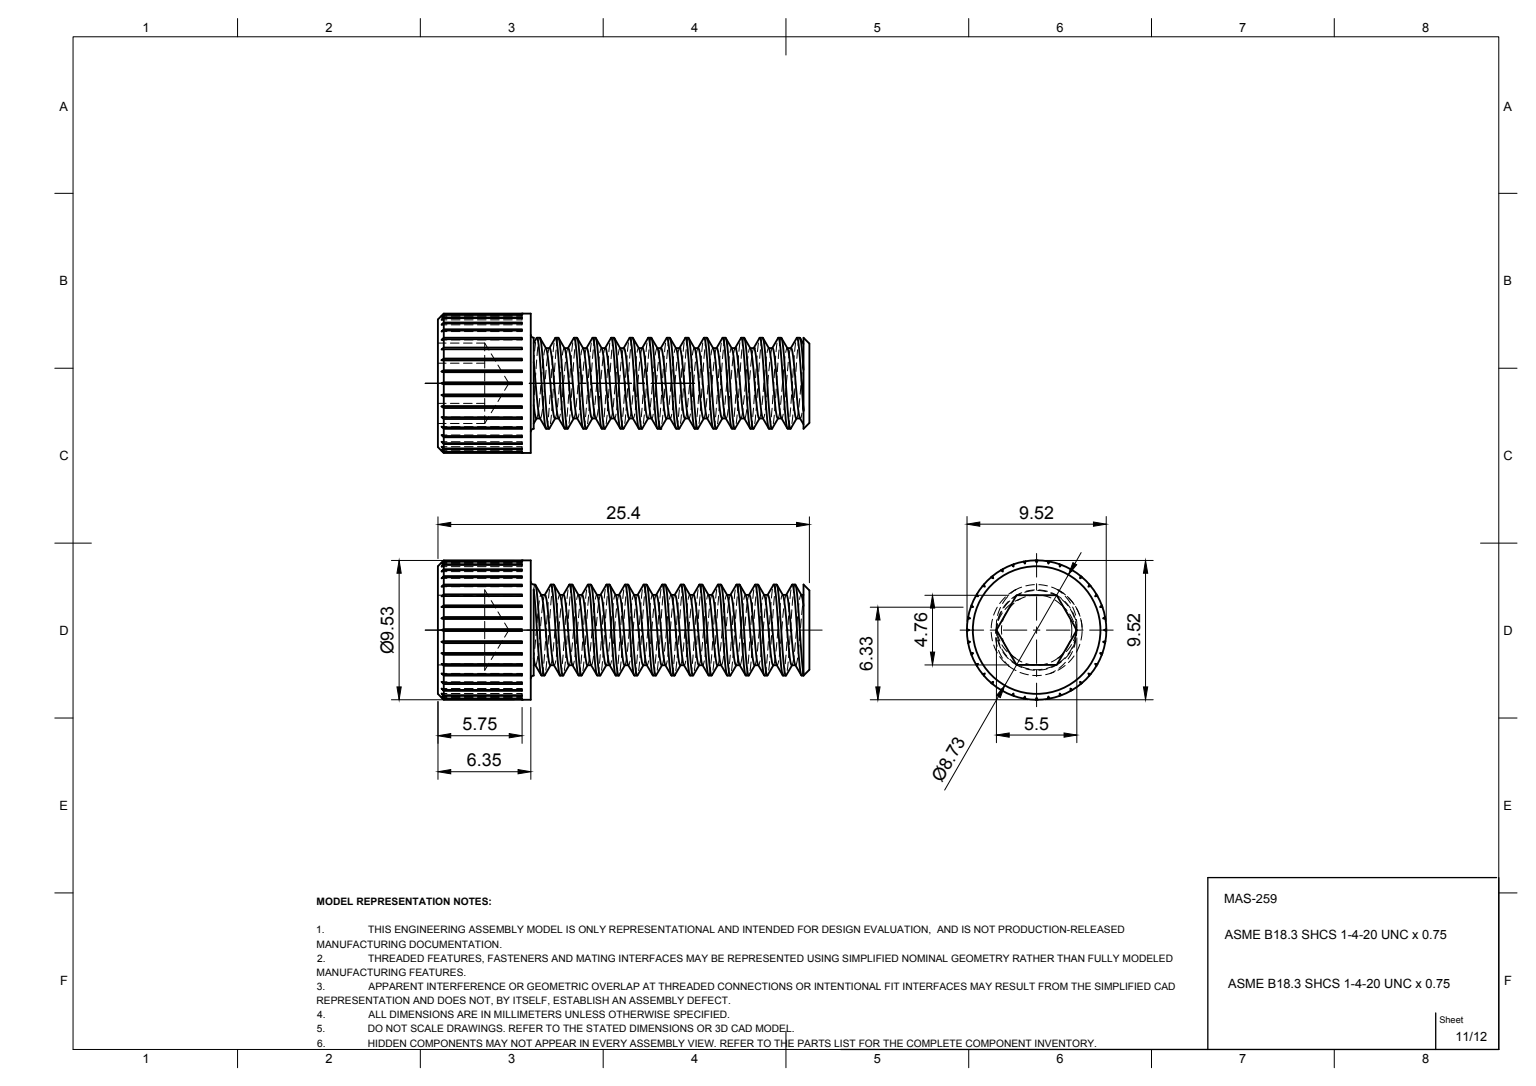
ISO-10303-21;
HEADER;
/* Generated by software containing ST-Developer
 * from STEP Tools, Inc. (www.steptools.com) 
 */

FILE_DESCRIPTION(
/* description */ (''),
/* implementation_level */ '2;1');

FILE_NAME(
/* name */ 'ASME B18.3 SHCS 1-4-20 UNC x 0.75.step',
/* time_stamp */ '2026-10-15T13:30:17-07:00',
/* author */ (''),
/* organization */ (''),
/* preprocessor_version */ 'ST-DEVELOPER v20.2',
/* originating_system */ 'Autodesk Translation Framework v15.15.0.0',
/* authorisation */ '');

FILE_SCHEMA (('AUTOMOTIVE_DESIGN { 1 0 10303 214 3 1 1 }'));
ENDSEC;

DATA;
#10=MECHANICAL_DESIGN_GEOMETRIC_PRESENTATION_REPRESENTATION('',(#1042),#71795);
#931=(
BOUNDED_CURVE()
B_SPLINE_CURVE(2,(#70734,#70735,#70736),.UNSPECIFIED.,.F.,.F.)
B_SPLINE_CURVE_WITH_KNOTS((3,3),(0.,0.0215367144649105),.UNSPECIFIED.)
CURVE()
GEOMETRIC_REPRESENTATION_ITEM()
RATIONAL_B_SPLINE_CURVE((1.,1.00042008979832,1.00053542481542))
REPRESENTATION_ITEM('')
);
#932=(
BOUNDED_CURVE()
B_SPLINE_CURVE(2,(#70741,#70742,#70743),.UNSPECIFIED.,.F.,.F.)
B_SPLINE_CURVE_WITH_KNOTS((3,3),(0.0378379342266191,0.0593746486914489),
 .UNSPECIFIED.)
CURVE()
GEOMETRIC_REPRESENTATION_ITEM()
RATIONAL_B_SPLINE_CURVE((1.00053542482002,1.00042008980193,1.))
REPRESENTATION_ITEM('')
);
#933=(
BOUNDED_CURVE()
B_SPLINE_CURVE(2,(#70750,#70751,#70752),.UNSPECIFIED.,.F.,.F.)
B_SPLINE_CURVE_WITH_KNOTS((3,3),(0.0378379342265495,0.0593746486914482),
 .UNSPECIFIED.)
CURVE()
GEOMETRIC_REPRESENTATION_ITEM()
RATIONAL_B_SPLINE_CURVE((1.00053542481289,1.00042008979634,1.))
REPRESENTATION_ITEM('')
);
#934=(
BOUNDED_CURVE()
B_SPLINE_CURVE(2,(#70756,#70757,#70758),.UNSPECIFIED.,.F.,.F.)
B_SPLINE_CURVE_WITH_KNOTS((3,3),(0.,0.0215367144649402),.UNSPECIFIED.)
CURVE()
GEOMETRIC_REPRESENTATION_ITEM()
RATIONAL_B_SPLINE_CURVE((1.,1.00042008979471,1.00053542481081))
REPRESENTATION_ITEM('')
);
#935=(
BOUNDED_CURVE()
B_SPLINE_CURVE(2,(#70760,#70761,#70762),.UNSPECIFIED.,.F.,.F.)
B_SPLINE_CURVE_WITH_KNOTS((3,3),(0.0378379342265241,0.0593746486914486),
 .UNSPECIFIED.)
CURVE()
GEOMETRIC_REPRESENTATION_ITEM()
RATIONAL_B_SPLINE_CURVE((1.00053542481258,1.0004200897961,1.))
REPRESENTATION_ITEM('')
);
#936=(
BOUNDED_CURVE()
B_SPLINE_CURVE(2,(#70766,#70767,#70768),.UNSPECIFIED.,.F.,.F.)
B_SPLINE_CURVE_WITH_KNOTS((3,3),(0.,0.0215367144649098),.UNSPECIFIED.)
CURVE()
GEOMETRIC_REPRESENTATION_ITEM()
RATIONAL_B_SPLINE_CURVE((1.,1.00042008979542,1.00053542481172))
REPRESENTATION_ITEM('')
);
#937=(
BOUNDED_CURVE()
B_SPLINE_CURVE(2,(#70770,#70771,#70772),.UNSPECIFIED.,.F.,.F.)
B_SPLINE_CURVE_WITH_KNOTS((3,3),(0.0378379342265049,0.0593746486914484),
 .UNSPECIFIED.)
CURVE()
GEOMETRIC_REPRESENTATION_ITEM()
RATIONAL_B_SPLINE_CURVE((1.00053542481297,1.0004200897964,1.))
REPRESENTATION_ITEM('')
);
#938=(
BOUNDED_CURVE()
B_SPLINE_CURVE(2,(#70776,#70777,#70778),.UNSPECIFIED.,.F.,.F.)
B_SPLINE_CURVE_WITH_KNOTS((3,3),(0.,0.0215367144648988),.UNSPECIFIED.)
CURVE()
GEOMETRIC_REPRESENTATION_ITEM()
RATIONAL_B_SPLINE_CURVE((1.,1.00042008979632,1.00053542481287))
REPRESENTATION_ITEM('')
);
#939=(
BOUNDED_CURVE()
B_SPLINE_CURVE(2,(#70780,#70781,#70782),.UNSPECIFIED.,.F.,.F.)
B_SPLINE_CURVE_WITH_KNOTS((3,3),(0.0378379342265885,0.0593746486914481),
 .UNSPECIFIED.)
CURVE()
GEOMETRIC_REPRESENTATION_ITEM()
RATIONAL_B_SPLINE_CURVE((1.00053542481452,1.00042008979762,1.))
REPRESENTATION_ITEM('')
);
#940=(
BOUNDED_CURVE()
B_SPLINE_CURVE(2,(#70786,#70787,#70788),.UNSPECIFIED.,.F.,.F.)
B_SPLINE_CURVE_WITH_KNOTS((3,3),(0.,0.021536714464922),.UNSPECIFIED.)
CURVE()
GEOMETRIC_REPRESENTATION_ITEM()
RATIONAL_B_SPLINE_CURVE((1.,1.0004200897977,1.00053542481463))
REPRESENTATION_ITEM('')
);
#941=(
BOUNDED_CURVE()
B_SPLINE_CURVE(2,(#70790,#70791,#70792),.UNSPECIFIED.,.F.,.F.)
B_SPLINE_CURVE_WITH_KNOTS((3,3),(0.0378379342265092,0.0593746486914482),
 .UNSPECIFIED.)
CURVE()
GEOMETRIC_REPRESENTATION_ITEM()
RATIONAL_B_SPLINE_CURVE((1.00053542481205,1.00042008979567,1.))
REPRESENTATION_ITEM('')
);
#942=(
BOUNDED_CURVE()
B_SPLINE_CURVE(2,(#70796,#70797,#70798),.UNSPECIFIED.,.F.,.F.)
B_SPLINE_CURVE_WITH_KNOTS((3,3),(0.,0.0215367144648869),.UNSPECIFIED.)
CURVE()
GEOMETRIC_REPRESENTATION_ITEM()
RATIONAL_B_SPLINE_CURVE((1.,1.00042008979756,1.00053542481445))
REPRESENTATION_ITEM('')
);
#943=(
BOUNDED_CURVE()
B_SPLINE_CURVE(2,(#70800,#70801,#70802),.UNSPECIFIED.,.F.,.F.)
B_SPLINE_CURVE_WITH_KNOTS((3,3),(0.0378379342265307,0.0593746486914478),
 .UNSPECIFIED.)
CURVE()
GEOMETRIC_REPRESENTATION_ITEM()
RATIONAL_B_SPLINE_CURVE((1.00053542481432,1.00042008979746,1.))
REPRESENTATION_ITEM('')
);
#944=(
BOUNDED_CURVE()
B_SPLINE_CURVE(2,(#70806,#70807,#70808),.UNSPECIFIED.,.F.,.F.)
B_SPLINE_CURVE_WITH_KNOTS((3,3),(0.,0.0215367144649457),.UNSPECIFIED.)
CURVE()
GEOMETRIC_REPRESENTATION_ITEM()
RATIONAL_B_SPLINE_CURVE((1.,1.00042008979626,1.00053542481279))
REPRESENTATION_ITEM('')
);
#945=(
BOUNDED_CURVE()
B_SPLINE_CURVE(2,(#70810,#70811,#70812),.UNSPECIFIED.,.F.,.F.)
B_SPLINE_CURVE_WITH_KNOTS((3,3),(0.0378379342264978,0.0593746486914476),
 .UNSPECIFIED.)
CURVE()
GEOMETRIC_REPRESENTATION_ITEM()
RATIONAL_B_SPLINE_CURVE((1.00053542480725,1.00042008979192,1.))
REPRESENTATION_ITEM('')
);
#946=(
BOUNDED_CURVE()
B_SPLINE_CURVE(2,(#70816,#70817,#70818),.UNSPECIFIED.,.F.,.F.)
B_SPLINE_CURVE_WITH_KNOTS((3,3),(0.,0.0215367144648818),.UNSPECIFIED.)
CURVE()
GEOMETRIC_REPRESENTATION_ITEM()
RATIONAL_B_SPLINE_CURVE((1.,1.00042008979656,1.00053542481317))
REPRESENTATION_ITEM('')
);
#947=(
BOUNDED_CURVE()
B_SPLINE_CURVE(2,(#70820,#70821,#70822),.UNSPECIFIED.,.F.,.F.)
B_SPLINE_CURVE_WITH_KNOTS((3,3),(0.0378379342265614,0.0593746486914475),
 .UNSPECIFIED.)
CURVE()
GEOMETRIC_REPRESENTATION_ITEM()
RATIONAL_B_SPLINE_CURVE((1.00053542481625,1.00042008979897,1.))
REPRESENTATION_ITEM('')
);
#948=(
BOUNDED_CURVE()
B_SPLINE_CURVE(2,(#70826,#70827,#70828),.UNSPECIFIED.,.F.,.F.)
B_SPLINE_CURVE_WITH_KNOTS((3,3),(0.,0.0215367144648944),.UNSPECIFIED.)
CURVE()
GEOMETRIC_REPRESENTATION_ITEM()
RATIONAL_B_SPLINE_CURVE((1.,1.00042008979746,1.00053542481432))
REPRESENTATION_ITEM('')
);
#949=(
BOUNDED_CURVE()
B_SPLINE_CURVE(2,(#70830,#70831,#70832),.UNSPECIFIED.,.F.,.F.)
B_SPLINE_CURVE_WITH_KNOTS((3,3),(0.0378379342265643,0.0593746486914474),
 .UNSPECIFIED.)
CURVE()
GEOMETRIC_REPRESENTATION_ITEM()
RATIONAL_B_SPLINE_CURVE((1.00053542481547,1.00042008979836,1.))
REPRESENTATION_ITEM('')
);
#950=(
BOUNDED_CURVE()
B_SPLINE_CURVE(2,(#70836,#70837,#70838),.UNSPECIFIED.,.F.,.F.)
B_SPLINE_CURVE_WITH_KNOTS((3,3),(0.,0.0215367144648979),.UNSPECIFIED.)
CURVE()
GEOMETRIC_REPRESENTATION_ITEM()
RATIONAL_B_SPLINE_CURVE((1.,1.00042008979658,1.00053542481321))
REPRESENTATION_ITEM('')
);
#951=(
BOUNDED_CURVE()
B_SPLINE_CURVE(2,(#70840,#70841,#70842),.UNSPECIFIED.,.F.,.F.)
B_SPLINE_CURVE_WITH_KNOTS((3,3),(0.037837934226498,0.0593746486914474),
 .UNSPECIFIED.)
CURVE()
GEOMETRIC_REPRESENTATION_ITEM()
RATIONAL_B_SPLINE_CURVE((1.00053542481105,1.0004200897949,1.))
REPRESENTATION_ITEM('')
);
#952=(
BOUNDED_CURVE()
B_SPLINE_CURVE(2,(#70846,#70847,#70848),.UNSPECIFIED.,.F.,.F.)
B_SPLINE_CURVE_WITH_KNOTS((3,3),(0.,0.021536714464896),.UNSPECIFIED.)
CURVE()
GEOMETRIC_REPRESENTATION_ITEM()
RATIONAL_B_SPLINE_CURVE((1.,1.00042008979607,1.00053542481255))
REPRESENTATION_ITEM('')
);
#953=(
BOUNDED_CURVE()
B_SPLINE_CURVE(2,(#70850,#70851,#70852),.UNSPECIFIED.,.F.,.F.)
B_SPLINE_CURVE_WITH_KNOTS((3,3),(0.0378379342264847,0.0593746486914478),
 .UNSPECIFIED.)
CURVE()
GEOMETRIC_REPRESENTATION_ITEM()
RATIONAL_B_SPLINE_CURVE((1.00053542480987,1.00042008979397,1.))
REPRESENTATION_ITEM('')
);
#954=(
BOUNDED_CURVE()
B_SPLINE_CURVE(2,(#70856,#70857,#70858),.UNSPECIFIED.,.F.,.F.)
B_SPLINE_CURVE_WITH_KNOTS((3,3),(0.,0.0215367144649515),.UNSPECIFIED.)
CURVE()
GEOMETRIC_REPRESENTATION_ITEM()
RATIONAL_B_SPLINE_CURVE((1.,1.00042008979379,1.00053542480965))
REPRESENTATION_ITEM('')
);
#955=(
BOUNDED_CURVE()
B_SPLINE_CURVE(2,(#70860,#70861,#70862),.UNSPECIFIED.,.F.,.F.)
B_SPLINE_CURVE_WITH_KNOTS((3,3),(0.0378379342265934,0.0593746486914471),
 .UNSPECIFIED.)
CURVE()
GEOMETRIC_REPRESENTATION_ITEM()
RATIONAL_B_SPLINE_CURVE((1.00053542481303,1.00042008979644,1.))
REPRESENTATION_ITEM('')
);
#956=(
BOUNDED_CURVE()
B_SPLINE_CURVE(2,(#70866,#70867,#70868),.UNSPECIFIED.,.F.,.F.)
B_SPLINE_CURVE_WITH_KNOTS((3,3),(0.,0.0215367144649196),.UNSPECIFIED.)
CURVE()
GEOMETRIC_REPRESENTATION_ITEM()
RATIONAL_B_SPLINE_CURVE((1.,1.00042008979619,1.00053542481271))
REPRESENTATION_ITEM('')
);
#957=(
BOUNDED_CURVE()
B_SPLINE_CURVE(2,(#70870,#70871,#70872),.UNSPECIFIED.,.F.,.F.)
B_SPLINE_CURVE_WITH_KNOTS((3,3),(0.0378379342265594,0.0593746486914476),
 .UNSPECIFIED.)
CURVE()
GEOMETRIC_REPRESENTATION_ITEM()
RATIONAL_B_SPLINE_CURVE((1.00053542481439,1.00042008979752,1.))
REPRESENTATION_ITEM('')
);
#958=(
BOUNDED_CURVE()
B_SPLINE_CURVE(2,(#70876,#70877,#70878),.UNSPECIFIED.,.F.,.F.)
B_SPLINE_CURVE_WITH_KNOTS((3,3),(0.,0.0215367144649124),.UNSPECIFIED.)
CURVE()
GEOMETRIC_REPRESENTATION_ITEM()
RATIONAL_B_SPLINE_CURVE((1.,1.00042008979906,1.00053542481637))
REPRESENTATION_ITEM('')
);
#959=(
BOUNDED_CURVE()
B_SPLINE_CURVE(2,(#70880,#70881,#70882),.UNSPECIFIED.,.F.,.F.)
B_SPLINE_CURVE_WITH_KNOTS((3,3),(0.0378379342265818,0.0593746486914467),
 .UNSPECIFIED.)
CURVE()
GEOMETRIC_REPRESENTATION_ITEM()
RATIONAL_B_SPLINE_CURVE((1.00053542480684,1.00042008979159,1.))
REPRESENTATION_ITEM('')
);
#960=(
BOUNDED_CURVE()
B_SPLINE_CURVE(2,(#70886,#70887,#70888),.UNSPECIFIED.,.F.,.F.)
B_SPLINE_CURVE_WITH_KNOTS((3,3),(0.,0.021536714464952),.UNSPECIFIED.)
CURVE()
GEOMETRIC_REPRESENTATION_ITEM()
RATIONAL_B_SPLINE_CURVE((1.,1.00042008979707,1.00053542481383))
REPRESENTATION_ITEM('')
);
#961=(
BOUNDED_CURVE()
B_SPLINE_CURVE(2,(#70890,#70891,#70892),.UNSPECIFIED.,.F.,.F.)
B_SPLINE_CURVE_WITH_KNOTS((3,3),(0.0378379342265293,0.0593746486914474),
 .UNSPECIFIED.)
CURVE()
GEOMETRIC_REPRESENTATION_ITEM()
RATIONAL_B_SPLINE_CURVE((1.00053542480889,1.0004200897932,1.))
REPRESENTATION_ITEM('')
);
#962=(
BOUNDED_CURVE()
B_SPLINE_CURVE(2,(#70896,#70897,#70898),.UNSPECIFIED.,.F.,.F.)
B_SPLINE_CURVE_WITH_KNOTS((3,3),(0.,0.0215367144649713),.UNSPECIFIED.)
CURVE()
GEOMETRIC_REPRESENTATION_ITEM()
RATIONAL_B_SPLINE_CURVE((1.,1.00042008978867,1.00053542480312))
REPRESENTATION_ITEM('')
);
#963=(
BOUNDED_CURVE()
B_SPLINE_CURVE(2,(#70900,#70901,#70902),.UNSPECIFIED.,.F.,.F.)
B_SPLINE_CURVE_WITH_KNOTS((3,3),(0.0378379342265233,0.0593746486914479),
 .UNSPECIFIED.)
CURVE()
GEOMETRIC_REPRESENTATION_ITEM()
RATIONAL_B_SPLINE_CURVE((1.00053542481454,1.00042008979763,1.))
REPRESENTATION_ITEM('')
);
#964=(
BOUNDED_CURVE()
B_SPLINE_CURVE(2,(#70906,#70907,#70908),.UNSPECIFIED.,.F.,.F.)
B_SPLINE_CURVE_WITH_KNOTS((3,3),(0.,0.0215367144648066),.UNSPECIFIED.)
CURVE()
GEOMETRIC_REPRESENTATION_ITEM()
RATIONAL_B_SPLINE_CURVE((1.,1.00042008980092,1.00053542481873))
REPRESENTATION_ITEM('')
);
#965=(
BOUNDED_CURVE()
B_SPLINE_CURVE(2,(#70910,#70911,#70912),.UNSPECIFIED.,.F.,.F.)
B_SPLINE_CURVE_WITH_KNOTS((3,3),(0.0378379342265035,0.0593746486914475),
 .UNSPECIFIED.)
CURVE()
GEOMETRIC_REPRESENTATION_ITEM()
RATIONAL_B_SPLINE_CURVE((1.00053542481437,1.0004200897975,1.))
REPRESENTATION_ITEM('')
);
#966=(
BOUNDED_CURVE()
B_SPLINE_CURVE(2,(#70916,#70917,#70918),.UNSPECIFIED.,.F.,.F.)
B_SPLINE_CURVE_WITH_KNOTS((3,3),(0.,0.0215367144649832),.UNSPECIFIED.)
CURVE()
GEOMETRIC_REPRESENTATION_ITEM()
RATIONAL_B_SPLINE_CURVE((1.,1.00042008978849,1.00053542480288))
REPRESENTATION_ITEM('')
);
#967=(
BOUNDED_CURVE()
B_SPLINE_CURVE(2,(#70920,#70921,#70922),.UNSPECIFIED.,.F.,.F.)
B_SPLINE_CURVE_WITH_KNOTS((3,3),(0.0378379342264869,0.0593746486914472),
 .UNSPECIFIED.)
CURVE()
GEOMETRIC_REPRESENTATION_ITEM()
RATIONAL_B_SPLINE_CURVE((1.00053542480856,1.00042008979294,1.))
REPRESENTATION_ITEM('')
);
#968=(
BOUNDED_CURVE()
B_SPLINE_CURVE(2,(#70926,#70927,#70928),.UNSPECIFIED.,.F.,.F.)
B_SPLINE_CURVE_WITH_KNOTS((3,3),(0.,0.0215367144648701),.UNSPECIFIED.)
CURVE()
GEOMETRIC_REPRESENTATION_ITEM()
RATIONAL_B_SPLINE_CURVE((1.,1.00042008979633,1.00053542481289))
REPRESENTATION_ITEM('')
);
#969=(
BOUNDED_CURVE()
B_SPLINE_CURVE(2,(#70930,#70931,#70932),.UNSPECIFIED.,.F.,.F.)
B_SPLINE_CURVE_WITH_KNOTS((3,3),(0.0378379342266196,0.0593746486914466),
 .UNSPECIFIED.)
CURVE()
GEOMETRIC_REPRESENTATION_ITEM()
RATIONAL_B_SPLINE_CURVE((1.00053542481627,1.00042008979899,1.))
REPRESENTATION_ITEM('')
);
#970=(
BOUNDED_CURVE()
B_SPLINE_CURVE(2,(#70937,#70938,#70939),.UNSPECIFIED.,.F.,.F.)
B_SPLINE_CURVE_WITH_KNOTS((3,3),(0.,0.0215367144649364),.UNSPECIFIED.)
CURVE()
GEOMETRIC_REPRESENTATION_ITEM()
RATIONAL_B_SPLINE_CURVE((1.,1.00042008979495,1.00053542481112))
REPRESENTATION_ITEM('')
);
#971=(
BOUNDED_CURVE()
B_SPLINE_CURVE(2,(#70941,#70942,#70943),.UNSPECIFIED.,.F.,.F.)
B_SPLINE_CURVE_WITH_KNOTS((3,3),(0.0378379342265907,0.0593746486914489),
 .UNSPECIFIED.)
CURVE()
GEOMETRIC_REPRESENTATION_ITEM()
RATIONAL_B_SPLINE_CURVE((1.00053542481339,1.00042008979673,1.))
REPRESENTATION_ITEM('')
);
#972=(
BOUNDED_CURVE()
B_SPLINE_CURVE(2,(#70947,#70948,#70949),.UNSPECIFIED.,.F.,.F.)
B_SPLINE_CURVE_WITH_KNOTS((3,3),(0.,0.0215367144648983),.UNSPECIFIED.)
CURVE()
GEOMETRIC_REPRESENTATION_ITEM()
RATIONAL_B_SPLINE_CURVE((1.,1.00042008979758,1.00053542481447))
REPRESENTATION_ITEM('')
);
#973=(
BOUNDED_CURVE()
B_SPLINE_CURVE(2,(#70951,#70952,#70953),.UNSPECIFIED.,.F.,.F.)
B_SPLINE_CURVE_WITH_KNOTS((3,3),(0.0378379342266009,0.0593746486914487),
 .UNSPECIFIED.)
CURVE()
GEOMETRIC_REPRESENTATION_ITEM()
RATIONAL_B_SPLINE_CURVE((1.00053542481762,1.00042008980005,1.))
REPRESENTATION_ITEM('')
);
#974=(
BOUNDED_CURVE()
B_SPLINE_CURVE(2,(#70957,#70958,#70959),.UNSPECIFIED.,.F.,.F.)
B_SPLINE_CURVE_WITH_KNOTS((3,3),(0.,0.0215367144648523),.UNSPECIFIED.)
CURVE()
GEOMETRIC_REPRESENTATION_ITEM()
RATIONAL_B_SPLINE_CURVE((1.,1.00042008980162,1.00053542481963))
REPRESENTATION_ITEM('')
);
#975=(
BOUNDED_CURVE()
B_SPLINE_CURVE(2,(#70961,#70962,#70963),.UNSPECIFIED.,.F.,.F.)
B_SPLINE_CURVE_WITH_KNOTS((3,3),(0.0378379342266166,0.0593746486914488),
 .UNSPECIFIED.)
CURVE()
GEOMETRIC_REPRESENTATION_ITEM()
RATIONAL_B_SPLINE_CURVE((1.00053542482459,1.00042008980551,1.))
REPRESENTATION_ITEM('')
);
#976=(
BOUNDED_CURVE()
B_SPLINE_CURVE(2,(#70967,#70968,#70969),.UNSPECIFIED.,.F.,.F.)
B_SPLINE_CURVE_WITH_KNOTS((3,3),(0.,0.0215367144649508),.UNSPECIFIED.)
CURVE()
GEOMETRIC_REPRESENTATION_ITEM()
RATIONAL_B_SPLINE_CURVE((1.,1.00042008979412,1.00053542481006))
REPRESENTATION_ITEM('')
);
#977=(
BOUNDED_CURVE()
B_SPLINE_CURVE(2,(#70971,#70972,#70973),.UNSPECIFIED.,.F.,.F.)
B_SPLINE_CURVE_WITH_KNOTS((3,3),(0.0378379342265848,0.0593746486914484),
 .UNSPECIFIED.)
CURVE()
GEOMETRIC_REPRESENTATION_ITEM()
RATIONAL_B_SPLINE_CURVE((1.00053542481552,1.0004200897984,1.))
REPRESENTATION_ITEM('')
);
#978=(
BOUNDED_CURVE()
B_SPLINE_CURVE(2,(#70977,#70978,#70979),.UNSPECIFIED.,.F.,.F.)
B_SPLINE_CURVE_WITH_KNOTS((3,3),(0.,0.0215367144649591),.UNSPECIFIED.)
CURVE()
GEOMETRIC_REPRESENTATION_ITEM()
RATIONAL_B_SPLINE_CURVE((1.,1.00042008979621,1.00053542481272))
REPRESENTATION_ITEM('')
);
#979=(
BOUNDED_CURVE()
B_SPLINE_CURVE(2,(#70981,#70982,#70983),.UNSPECIFIED.,.F.,.F.)
B_SPLINE_CURVE_WITH_KNOTS((3,3),(0.037837934226528,0.0593746486914486),
 .UNSPECIFIED.)
CURVE()
GEOMETRIC_REPRESENTATION_ITEM()
RATIONAL_B_SPLINE_CURVE((1.00053542481249,1.00042008979602,1.))
REPRESENTATION_ITEM('')
);
#980=(
BOUNDED_CURVE()
B_SPLINE_CURVE(2,(#70987,#70988,#70989),.UNSPECIFIED.,.F.,.F.)
B_SPLINE_CURVE_WITH_KNOTS((3,3),(0.,0.0215367144649439),.UNSPECIFIED.)
CURVE()
GEOMETRIC_REPRESENTATION_ITEM()
RATIONAL_B_SPLINE_CURVE((1.,1.00042008979311,1.00053542480878))
REPRESENTATION_ITEM('')
);
#981=(
BOUNDED_CURVE()
B_SPLINE_CURVE(2,(#70991,#70992,#70993),.UNSPECIFIED.,.F.,.F.)
B_SPLINE_CURVE_WITH_KNOTS((3,3),(0.0378379342265471,0.0593746486914486),
 .UNSPECIFIED.)
CURVE()
GEOMETRIC_REPRESENTATION_ITEM()
RATIONAL_B_SPLINE_CURVE((1.00053542480963,1.00042008979378,1.))
REPRESENTATION_ITEM('')
);
#982=(
BOUNDED_CURVE()
B_SPLINE_CURVE(2,(#70997,#70998,#70999),.UNSPECIFIED.,.F.,.F.)
B_SPLINE_CURVE_WITH_KNOTS((3,3),(0.,0.0215367144649546),.UNSPECIFIED.)
CURVE()
GEOMETRIC_REPRESENTATION_ITEM()
RATIONAL_B_SPLINE_CURVE((1.,1.00042008979267,1.00053542480822))
REPRESENTATION_ITEM('')
);
#983=(
BOUNDED_CURVE()
B_SPLINE_CURVE(2,(#71001,#71002,#71003),.UNSPECIFIED.,.F.,.F.)
B_SPLINE_CURVE_WITH_KNOTS((3,3),(0.0378379342265707,0.0593746486914487),
 .UNSPECIFIED.)
CURVE()
GEOMETRIC_REPRESENTATION_ITEM()
RATIONAL_B_SPLINE_CURVE((1.0005354248134,1.00042008979673,1.))
REPRESENTATION_ITEM('')
);
#984=(
BOUNDED_CURVE()
B_SPLINE_CURVE(2,(#71007,#71008,#71009),.UNSPECIFIED.,.F.,.F.)
B_SPLINE_CURVE_WITH_KNOTS((3,3),(0.,0.0215367144649525),.UNSPECIFIED.)
CURVE()
GEOMETRIC_REPRESENTATION_ITEM()
RATIONAL_B_SPLINE_CURVE((1.,1.0004200897947,1.0005354248108))
REPRESENTATION_ITEM('')
);
#985=(
BOUNDED_CURVE()
B_SPLINE_CURVE(2,(#71011,#71012,#71013),.UNSPECIFIED.,.F.,.F.)
B_SPLINE_CURVE_WITH_KNOTS((3,3),(0.0378379342265302,0.059374648691449),
 .UNSPECIFIED.)
CURVE()
GEOMETRIC_REPRESENTATION_ITEM()
RATIONAL_B_SPLINE_CURVE((1.00053542480972,1.00042008979385,1.))
REPRESENTATION_ITEM('')
);
#986=(
BOUNDED_CURVE()
B_SPLINE_CURVE(2,(#71017,#71018,#71019),.UNSPECIFIED.,.F.,.F.)
B_SPLINE_CURVE_WITH_KNOTS((3,3),(0.,0.0215367144649366),.UNSPECIFIED.)
CURVE()
GEOMETRIC_REPRESENTATION_ITEM()
RATIONAL_B_SPLINE_CURVE((1.,1.00042008979726,1.00053542481407))
REPRESENTATION_ITEM('')
);
#987=(
BOUNDED_CURVE()
B_SPLINE_CURVE(2,(#71021,#71022,#71023),.UNSPECIFIED.,.F.,.F.)
B_SPLINE_CURVE_WITH_KNOTS((3,3),(0.0378379342265197,0.0593746486914487),
 .UNSPECIFIED.)
CURVE()
GEOMETRIC_REPRESENTATION_ITEM()
RATIONAL_B_SPLINE_CURVE((1.00053542480866,1.00042008979301,1.))
REPRESENTATION_ITEM('')
);
#988=(
BOUNDED_CURVE()
B_SPLINE_CURVE(2,(#71027,#71028,#71029),.UNSPECIFIED.,.F.,.F.)
B_SPLINE_CURVE_WITH_KNOTS((3,3),(0.,0.0215367144649012),.UNSPECIFIED.)
CURVE()
GEOMETRIC_REPRESENTATION_ITEM()
RATIONAL_B_SPLINE_CURVE((1.,1.00042008979525,1.0005354248115))
REPRESENTATION_ITEM('')
);
#989=(
BOUNDED_CURVE()
B_SPLINE_CURVE(2,(#71031,#71032,#71033),.UNSPECIFIED.,.F.,.F.)
B_SPLINE_CURVE_WITH_KNOTS((3,3),(0.0378379342265321,0.0593746486914488),
 .UNSPECIFIED.)
CURVE()
GEOMETRIC_REPRESENTATION_ITEM()
RATIONAL_B_SPLINE_CURVE((1.00053542481087,1.00042008979475,1.))
REPRESENTATION_ITEM('')
);
#990=(
BOUNDED_CURVE()
B_SPLINE_CURVE(2,(#71037,#71038,#71039),.UNSPECIFIED.,.F.,.F.)
B_SPLINE_CURVE_WITH_KNOTS((3,3),(0.,0.0215367144649128),.UNSPECIFIED.)
CURVE()
GEOMETRIC_REPRESENTATION_ITEM()
RATIONAL_B_SPLINE_CURVE((1.,1.00042008979245,1.00053542480793))
REPRESENTATION_ITEM('')
);
#991=(
BOUNDED_CURVE()
B_SPLINE_CURVE(2,(#71041,#71042,#71043),.UNSPECIFIED.,.F.,.F.)
B_SPLINE_CURVE_WITH_KNOTS((3,3),(0.0378379342265115,0.0593746486914485),
 .UNSPECIFIED.)
CURVE()
GEOMETRIC_REPRESENTATION_ITEM()
RATIONAL_B_SPLINE_CURVE((1.0005354248112,1.00042008979501,1.))
REPRESENTATION_ITEM('')
);
#992=(
BOUNDED_CURVE()
B_SPLINE_CURVE(2,(#71047,#71048,#71049),.UNSPECIFIED.,.F.,.F.)
B_SPLINE_CURVE_WITH_KNOTS((3,3),(0.,0.0215367144649508),.UNSPECIFIED.)
CURVE()
GEOMETRIC_REPRESENTATION_ITEM()
RATIONAL_B_SPLINE_CURVE((1.,1.00042008979591,1.00053542481235))
REPRESENTATION_ITEM('')
);
#993=(
BOUNDED_CURVE()
B_SPLINE_CURVE(2,(#71051,#71052,#71053),.UNSPECIFIED.,.F.,.F.)
B_SPLINE_CURVE_WITH_KNOTS((3,3),(0.0378379342265331,0.0593746486914485),
 .UNSPECIFIED.)
CURVE()
GEOMETRIC_REPRESENTATION_ITEM()
RATIONAL_B_SPLINE_CURVE((1.00053542481272,1.0004200897962,1.))
REPRESENTATION_ITEM('')
);
#994=(
BOUNDED_CURVE()
B_SPLINE_CURVE(2,(#71057,#71058,#71059),.UNSPECIFIED.,.F.,.F.)
B_SPLINE_CURVE_WITH_KNOTS((3,3),(0.,0.0215367144649045),.UNSPECIFIED.)
CURVE()
GEOMETRIC_REPRESENTATION_ITEM()
RATIONAL_B_SPLINE_CURVE((1.,1.0004200897958,1.00053542481221))
REPRESENTATION_ITEM('')
);
#995=(
BOUNDED_CURVE()
B_SPLINE_CURVE(2,(#71061,#71062,#71063),.UNSPECIFIED.,.F.,.F.)
B_SPLINE_CURVE_WITH_KNOTS((3,3),(0.0378379342265301,0.0593746486914479),
 .UNSPECIFIED.)
CURVE()
GEOMETRIC_REPRESENTATION_ITEM()
RATIONAL_B_SPLINE_CURVE((1.00053542481236,1.00042008979592,1.))
REPRESENTATION_ITEM('')
);
#996=(
BOUNDED_CURVE()
B_SPLINE_CURVE(2,(#71067,#71068,#71069),.UNSPECIFIED.,.F.,.F.)
B_SPLINE_CURVE_WITH_KNOTS((3,3),(0.,0.0215367144649068),.UNSPECIFIED.)
CURVE()
GEOMETRIC_REPRESENTATION_ITEM()
RATIONAL_B_SPLINE_CURVE((1.,1.00042008979466,1.00053542481075))
REPRESENTATION_ITEM('')
);
#997=(
BOUNDED_CURVE()
B_SPLINE_CURVE(2,(#71071,#71072,#71073),.UNSPECIFIED.,.F.,.F.)
B_SPLINE_CURVE_WITH_KNOTS((3,3),(0.0378379342265604,0.0593746486914483),
 .UNSPECIFIED.)
CURVE()
GEOMETRIC_REPRESENTATION_ITEM()
RATIONAL_B_SPLINE_CURVE((1.00053542481646,1.00042008979914,1.))
REPRESENTATION_ITEM('')
);
#998=(
BOUNDED_CURVE()
B_SPLINE_CURVE(2,(#71077,#71078,#71079),.UNSPECIFIED.,.F.,.F.)
B_SPLINE_CURVE_WITH_KNOTS((3,3),(0.,0.0215367144649594),.UNSPECIFIED.)
CURVE()
GEOMETRIC_REPRESENTATION_ITEM()
RATIONAL_B_SPLINE_CURVE((1.,1.00042008979357,1.00053542480936))
REPRESENTATION_ITEM('')
);
#999=(
BOUNDED_CURVE()
B_SPLINE_CURVE(2,(#71081,#71082,#71083),.UNSPECIFIED.,.F.,.F.)
B_SPLINE_CURVE_WITH_KNOTS((3,3),(0.0378379342265812,0.0593746486914485),
 .UNSPECIFIED.)
CURVE()
GEOMETRIC_REPRESENTATION_ITEM()
RATIONAL_B_SPLINE_CURVE((1.00053542481548,1.00042008979837,1.))
REPRESENTATION_ITEM('')
);
#1000=(
BOUNDED_CURVE()
B_SPLINE_CURVE(2,(#71087,#71088,#71089),.UNSPECIFIED.,.F.,.F.)
B_SPLINE_CURVE_WITH_KNOTS((3,3),(0.,0.0215367144649258),.UNSPECIFIED.)
CURVE()
GEOMETRIC_REPRESENTATION_ITEM()
RATIONAL_B_SPLINE_CURVE((1.,1.00042008979633,1.00053542481288))
REPRESENTATION_ITEM('')
);
#1001=(
BOUNDED_CURVE()
B_SPLINE_CURVE(2,(#71091,#71092,#71093),.UNSPECIFIED.,.F.,.F.)
B_SPLINE_CURVE_WITH_KNOTS((3,3),(0.0378379342265631,0.0593746486914488),
 .UNSPECIFIED.)
CURVE()
GEOMETRIC_REPRESENTATION_ITEM()
RATIONAL_B_SPLINE_CURVE((1.00053542481617,1.00042008979891,1.))
REPRESENTATION_ITEM('')
);
#1002=(
BOUNDED_CURVE()
B_SPLINE_CURVE(2,(#71096,#71097,#71098),.UNSPECIFIED.,.F.,.F.)
B_SPLINE_CURVE_WITH_KNOTS((3,3),(0.,0.0215367144650048),.UNSPECIFIED.)
CURVE()
GEOMETRIC_REPRESENTATION_ITEM()
RATIONAL_B_SPLINE_CURVE((1.,1.00042008979356,1.00053542480934))
REPRESENTATION_ITEM('')
);
#1005=TOROIDAL_SURFACE('',#14637,3.31023,0.2);
#1010=B_SPLINE_SURFACE_WITH_KNOTS('',3,3,((#69746,#69747,#69748,#69749,
#69750,#69751,#69752,#69753,#69754,#69755,#69756,#69757,#69758,#69759,#69760,
#69761,#69762,#69763,#69764,#69765,#69766,#69767,#69768,#69769,#69770,#69771,
#69772,#69773,#69774,#69775,#69776,#69777,#69778,#69779,#69780,#69781,#69782,
#69783,#69784,#69785,#69786,#69787,#69788,#69789,#69790,#69791,#69792,#69793,
#69794,#69795,#69796,#69797,#69798,#69799,#69800,#69801,#69802,#69803,#69804,
#69805,#69806,#69807,#69808,#69809,#69810,#69811,#69812,#69813,#69814,#69815,
#69816,#69817,#69818,#69819,#69820,#69821,#69822,#69823,#69824,#69825,#69826,
#69827,#69828,#69829,#69830,#69831,#69832,#69833,#69834,#69835,#69836,#69837,
#69838,#69839,#69840,#69841,#69842),(#69843,#69844,#69845,#69846,#69847,
#69848,#69849,#69850,#69851,#69852,#69853,#69854,#69855,#69856,#69857,#69858,
#69859,#69860,#69861,#69862,#69863,#69864,#69865,#69866,#69867,#69868,#69869,
#69870,#69871,#69872,#69873,#69874,#69875,#69876,#69877,#69878,#69879,#69880,
#69881,#69882,#69883,#69884,#69885,#69886,#69887,#69888,#69889,#69890,#69891,
#69892,#69893,#69894,#69895,#69896,#69897,#69898,#69899,#69900,#69901,#69902,
#69903,#69904,#69905,#69906,#69907,#69908,#69909,#69910,#69911,#69912,#69913,
#69914,#69915,#69916,#69917,#69918,#69919,#69920,#69921,#69922,#69923,#69924,
#69925,#69926,#69927,#69928,#69929,#69930,#69931,#69932,#69933,#69934,#69935,
#69936,#69937,#69938,#69939),(#69940,#69941,#69942,#69943,#69944,#69945,
#69946,#69947,#69948,#69949,#69950,#69951,#69952,#69953,#69954,#69955,#69956,
#69957,#69958,#69959,#69960,#69961,#69962,#69963,#69964,#69965,#69966,#69967,
#69968,#69969,#69970,#69971,#69972,#69973,#69974,#69975,#69976,#69977,#69978,
#69979,#69980,#69981,#69982,#69983,#69984,#69985,#69986,#69987,#69988,#69989,
#69990,#69991,#69992,#69993,#69994,#69995,#69996,#69997,#69998,#69999,#70000,
#70001,#70002,#70003,#70004,#70005,#70006,#70007,#70008,#70009,#70010,#70011,
#70012,#70013,#70014,#70015,#70016,#70017,#70018,#70019,#70020,#70021,#70022,
#70023,#70024,#70025,#70026,#70027,#70028,#70029,#70030,#70031,#70032,#70033,
#70034,#70035,#70036),(#70037,#70038,#70039,#70040,#70041,#70042,#70043,
#70044,#70045,#70046,#70047,#70048,#70049,#70050,#70051,#70052,#70053,#70054,
#70055,#70056,#70057,#70058,#70059,#70060,#70061,#70062,#70063,#70064,#70065,
#70066,#70067,#70068,#70069,#70070,#70071,#70072,#70073,#70074,#70075,#70076,
#70077,#70078,#70079,#70080,#70081,#70082,#70083,#70084,#70085,#70086,#70087,
#70088,#70089,#70090,#70091,#70092,#70093,#70094,#70095,#70096,#70097,#70098,
#70099,#70100,#70101,#70102,#70103,#70104,#70105,#70106,#70107,#70108,#70109,
#70110,#70111,#70112,#70113,#70114,#70115,#70116,#70117,#70118,#70119,#70120,
#70121,#70122,#70123,#70124,#70125,#70126,#70127,#70128,#70129,#70130,#70131,
#70132,#70133)),.UNSPECIFIED.,.F.,.F.,.F.,(4,4),(4,1,1,1,1,1,1,1,1,1,1,
1,1,1,1,1,1,1,1,1,1,1,1,1,1,1,1,1,1,1,1,1,1,1,1,1,1,1,1,1,1,1,1,1,1,1,1,
1,1,1,1,1,1,1,1,1,1,1,1,1,1,1,1,1,1,1,1,1,1,1,1,1,1,1,1,1,1,1,1,1,1,1,1,
1,1,1,1,1,1,1,1,1,1,1,4),(-0.000489567166405237,0.0818460149219149),(8.32561554604337,
9.31809068326254,10.3105658204817,11.3030409577009,12.29551609492,13.2879912321392,
14.2804663693584,15.2729415065776,16.2654166437967,17.2578917810159,18.2503669182351,
19.2428420554542,20.2353171926734,21.2277923298926,22.2202674671117,23.2127426043309,
24.2052177415501,25.1976928787692,26.1901680159884,27.1826431532076,28.1751182904267,
29.1675934276459,30.1600685648651,31.1525437020842,32.1450188393034,33.1374939765226,
34.1299691137418,35.1224442509609,36.1149193881801,37.1073945253993,38.0998696626184,
39.0923447998376,40.0848199370568,41.0772950742759,42.0697702114951,43.0622453487143,
44.0547204859334,45.0471956231526,46.0396707603718,47.032145897591,48.0246210348101,
49.0170961720293,50.0095713092485,51.0020464464676,51.9945215836868,52.986996720906,
53.9794718581251,54.9719469953443,55.9644221325635,56.9568972697826,57.9493724070018,
58.941847544221,59.9343226814401,60.9267978186593,61.9192729558785,62.9117480930976,
63.9042232303168,64.896698367536,65.8891735047551,66.8816486419743,67.8741237791935,
68.8665989164127,69.8590740536318,70.851549190851,71.8440243280702,72.8364994652893,
73.8289746025085,74.8214497397277,75.8139248769468,76.806400014166,77.7988751513852,
78.7913502886043,79.7838254258235,80.7763005630427,81.7687757002619,82.761250837481,
83.7537259747002,84.7462011119194,85.7386762491385,86.7311513863577,87.7236265235769,
88.716101660796,89.7085767980152,90.7010519352344,91.6935270724535,92.6860022096727,
93.6784773468919,94.670952484111,95.6634276213302,96.6559027585494,97.6483778957685,
98.6408530329877,99.6333281702069,100.625803307426,101.618768011811),
 .UNSPECIFIED.);
#1011=B_SPLINE_SURFACE_WITH_KNOTS('',3,3,((#70322,#70323,#70324,#70325,
#70326,#70327,#70328,#70329,#70330,#70331,#70332,#70333,#70334,#70335,#70336,
#70337,#70338,#70339,#70340,#70341,#70342,#70343,#70344,#70345,#70346,#70347,
#70348,#70349,#70350,#70351,#70352,#70353,#70354,#70355,#70356,#70357,#70358,
#70359,#70360,#70361,#70362,#70363,#70364,#70365,#70366,#70367,#70368,#70369,
#70370,#70371,#70372,#70373,#70374,#70375,#70376,#70377,#70378,#70379,#70380,
#70381,#70382,#70383,#70384,#70385,#70386,#70387,#70388,#70389,#70390,#70391,
#70392,#70393,#70394,#70395,#70396,#70397,#70398,#70399,#70400,#70401,#70402,
#70403,#70404,#70405,#70406,#70407,#70408,#70409,#70410,#70411,#70412,#70413,
#70414,#70415,#70416,#70417,#70418),(#70419,#70420,#70421,#70422,#70423,
#70424,#70425,#70426,#70427,#70428,#70429,#70430,#70431,#70432,#70433,#70434,
#70435,#70436,#70437,#70438,#70439,#70440,#70441,#70442,#70443,#70444,#70445,
#70446,#70447,#70448,#70449,#70450,#70451,#70452,#70453,#70454,#70455,#70456,
#70457,#70458,#70459,#70460,#70461,#70462,#70463,#70464,#70465,#70466,#70467,
#70468,#70469,#70470,#70471,#70472,#70473,#70474,#70475,#70476,#70477,#70478,
#70479,#70480,#70481,#70482,#70483,#70484,#70485,#70486,#70487,#70488,#70489,
#70490,#70491,#70492,#70493,#70494,#70495,#70496,#70497,#70498,#70499,#70500,
#70501,#70502,#70503,#70504,#70505,#70506,#70507,#70508,#70509,#70510,#70511,
#70512,#70513,#70514,#70515),(#70516,#70517,#70518,#70519,#70520,#70521,
#70522,#70523,#70524,#70525,#70526,#70527,#70528,#70529,#70530,#70531,#70532,
#70533,#70534,#70535,#70536,#70537,#70538,#70539,#70540,#70541,#70542,#70543,
#70544,#70545,#70546,#70547,#70548,#70549,#70550,#70551,#70552,#70553,#70554,
#70555,#70556,#70557,#70558,#70559,#70560,#70561,#70562,#70563,#70564,#70565,
#70566,#70567,#70568,#70569,#70570,#70571,#70572,#70573,#70574,#70575,#70576,
#70577,#70578,#70579,#70580,#70581,#70582,#70583,#70584,#70585,#70586,#70587,
#70588,#70589,#70590,#70591,#70592,#70593,#70594,#70595,#70596,#70597,#70598,
#70599,#70600,#70601,#70602,#70603,#70604,#70605,#70606,#70607,#70608,#70609,
#70610,#70611,#70612),(#70613,#70614,#70615,#70616,#70617,#70618,#70619,
#70620,#70621,#70622,#70623,#70624,#70625,#70626,#70627,#70628,#70629,#70630,
#70631,#70632,#70633,#70634,#70635,#70636,#70637,#70638,#70639,#70640,#70641,
#70642,#70643,#70644,#70645,#70646,#70647,#70648,#70649,#70650,#70651,#70652,
#70653,#70654,#70655,#70656,#70657,#70658,#70659,#70660,#70661,#70662,#70663,
#70664,#70665,#70666,#70667,#70668,#70669,#70670,#70671,#70672,#70673,#70674,
#70675,#70676,#70677,#70678,#70679,#70680,#70681,#70682,#70683,#70684,#70685,
#70686,#70687,#70688,#70689,#70690,#70691,#70692,#70693,#70694,#70695,#70696,
#70697,#70698,#70699,#70700,#70701,#70702,#70703,#70704,#70705,#70706,#70707,
#70708,#70709)),.UNSPECIFIED.,.F.,.F.,.F.,(4,4),(4,1,1,1,1,1,1,1,1,1,1,
1,1,1,1,1,1,1,1,1,1,1,1,1,1,1,1,1,1,1,1,1,1,1,1,1,1,1,1,1,1,1,1,1,1,1,1,
1,1,1,1,1,1,1,1,1,1,1,1,1,1,1,1,1,1,1,1,1,1,1,1,1,1,1,1,1,1,1,1,1,1,1,1,
1,1,1,1,1,1,1,1,1,1,1,4),(-0.000437088768894676,0.0818785329593794),(11.6517262692733,
12.6446908720042,13.6371660092234,14.6296411464425,15.6221162836617,16.6145914208809,
17.6070665581,18.5995416953192,19.5920168325384,20.5844919697575,21.5769671069767,
22.5694422441959,23.5619173814151,24.5543925186342,25.5468676558534,26.5393427930726,
27.5318179302917,28.5242930675109,29.5167682047301,30.5092433419492,31.5017184791684,
32.4941936163876,33.4866687536067,34.4791438908259,35.4716190280451,36.4640941652642,
37.4565693024834,38.4490444397026,39.4415195769218,40.4339947141409,41.4264698513601,
42.4189449885793,43.4114201257984,44.4038952630176,45.3963704002368,46.3888455374559,
47.3813206746751,48.3737958118943,49.3662709491134,50.3587460863326,51.3512212235518,
52.3436963607709,53.3361714979901,54.3286466352093,55.3211217724285,56.3135969096476,
57.3060720468668,58.298547184086,59.2910223213051,60.2834974585243,61.2759725957435,
62.2684477329626,63.2609228701818,64.253398007401,65.2458731446201,66.2383482818393,
67.2308234190585,68.2232985562776,69.2157736934968,70.208248830716,71.2007239679351,
72.1931991051543,73.1856742423735,74.1781493795927,75.1706245168118,76.163099654031,
77.1555747912502,78.1480499284693,79.1405250656885,80.1330002029077,81.1254753401268,
82.117950477346,83.1104256145652,84.1029007517843,85.0953758890035,86.0878510262227,
87.0803261634419,88.072801300661,89.0652764378802,90.0577515750994,91.0502267123185,
92.0427018495377,93.0351769867569,94.027652123976,95.0201272611952,96.0126023984144,
97.0050775356335,97.9975526728527,98.9900278100719,99.982502947291,100.97497808451,
101.967453221729,102.959928358949,103.952403496168,104.944878633387),
 .UNSPECIFIED.);
#1022=SHAPE_REPRESENTATION_RELATIONSHIP('SRR','None',#72026,#1032);
#1032=ADVANCED_BREP_SHAPE_REPRESENTATION('',(#1052),#71794);
#1042=STYLED_ITEM('',(#72085),#1052);
#1052=MANIFOLD_SOLID_BREP('Body1',#13644);
#1100=CONICAL_SURFACE('',#14642,2.91023,0.785398163397448);
#1101=CONICAL_SURFACE('',#14649,4.5625,0.785398163397448);
#1102=CONICAL_SURFACE('',#14842,2.74963065701559,1.02974425867665);
#1399=B_SPLINE_CURVE_WITH_KNOTS('',3,(#59763,#59764,#59765,#59766,#59767,
#59768,#59769,#59770,#59771,#59772,#59773,#59774,#59775,#59776,#59777,#59778,
#59779,#59780,#59781,#59782,#59783,#59784,#59785,#59786,#59787,#59788,#59789,
#59790,#59791,#59792,#59793,#59794,#59795,#59796,#59797,#59798,#59799,#59800,
#59801,#59802,#59803,#59804,#59805,#59806,#59807,#59808,#59809,#59810,#59811,
#59812,#59813,#59814,#59815,#59816,#59817,#59818,#59819,#59820,#59821,#59822,
#59823,#59824,#59825,#59826,#59827,#59828,#59829,#59830,#59831,#59832,#59833,
#59834,#59835,#59836,#59837,#59838,#59839,#59840,#59841,#59842,#59843,#59844,
#59845,#59846,#59847,#59848,#59849,#59850,#59851,#59852,#59853,#59854,#59855,
#59856,#59857,#59858,#59859,#59860,#59861,#59862,#59863,#59864,#59865,#59866,
#59867,#59868,#59869,#59870,#59871,#59872,#59873,#59874,#59875,#59876,#59877,
#59878,#59879,#59880,#59881,#59882,#59883,#59884,#59885,#59886,#59887,#59888,
#59889,#59890,#59891,#59892,#59893,#59894,#59895,#59896,#59897,#59898,#59899,
#59900,#59901,#59902,#59903,#59904,#59905,#59906,#59907,#59908,#59909,#59910,
#59911,#59912,#59913,#59914,#59915,#59916),.UNSPECIFIED.,.F.,.F.,(4,3,3,
3,3,3,3,3,3,3,3,3,3,3,3,3,3,3,3,3,3,3,3,3,3,3,3,3,3,3,3,3,3,3,3,3,3,3,3,
3,3,3,3,3,3,3,3,3,3,3,3,4),(10.3390665670415,10.4389102386922,10.5386120657231,
10.6382011799414,10.7377295317413,10.8372284404688,10.9367291874285,11.0363271732773,
11.1359765274803,11.2357929021649,11.3030409577009,11.4034304911592,11.5036806043933,
11.6038203870021,11.7039000735038,11.8039502250711,11.9040013654047,12.0041527633794,
12.1043532357862,12.2047323921906,12.29551609492,12.3956256070617,12.495590671401,
12.5954391831491,12.6952239510319,12.7949759540912,12.8947261306514,12.9945742327021,
13.0944696581655,13.1945443542051,13.2879912321392,13.3882408851107,13.4883478478747,
13.5883402367819,13.6882700202373,13.788167975337,13.8880648394668,13.9880597667956,
14.0881023267245,14.1883229634351,14.2804663693584,14.3807107513822,14.4808127485467,
14.5808006601333,14.6807262662731,14.7806203507897,14.880513658085,14.9805055515609,
15.0805453590138,15.1807637564913,15.2729415065776,15.3376015162611),
 .UNSPECIFIED.);
#1400=B_SPLINE_CURVE_WITH_KNOTS('',3,(#59919,#59920,#59921,#59922,#59923,
#59924,#59925,#59926,#59927,#59928,#59929,#59930,#59931,#59932,#59933,#59934,
#59935,#59936,#59937,#59938,#59939,#59940,#59941,#59942,#59943,#59944,#59945,
#59946,#59947,#59948,#59949,#59950,#59951,#59952,#59953,#59954,#59955,#59956,
#59957,#59958,#59959,#59960,#59961,#59962,#59963,#59964,#59965,#59966,#59967,
#59968,#59969,#59970,#59971,#59972,#59973,#59974,#59975,#59976,#59977,#59978,
#59979,#59980,#59981,#59982,#59983,#59984,#59985,#59986,#59987,#59988,#59989,
#59990,#59991,#59992,#59993,#59994,#59995,#59996,#59997,#59998,#59999,#60000,
#60001,#60002,#60003,#60004,#60005,#60006,#60007,#60008,#60009,#60010,#60011,
#60012,#60013,#60014,#60015,#60016,#60017,#60018,#60019,#60020,#60021,#60022,
#60023,#60024,#60025,#60026,#60027,#60028,#60029,#60030),.UNSPECIFIED.,
 .F.,.F.,(4,3,3,3,3,3,3,3,3,3,3,3,3,3,3,3,3,3,3,3,3,3,3,3,3,3,3,3,3,3,3,
3,3,3,3,3,3,4),(11.652215734785,11.7547070075903,11.8571355266317,11.9595527584582,
12.0619674638986,12.1644046457875,12.2668893252805,12.3695249047339,12.4722399736612,
12.5751521582194,12.6446908720042,12.7439827386589,12.8431176847019,12.9423737252671,
13.0413040056414,13.1401936380512,13.239074595373,13.3385974488356,13.437614586494,
13.5373902978587,13.6371660092234,13.7375076850693,13.8377063835552,13.9377896041002,
14.0378096181711,14.1377970659549,14.2377825472796,14.3378640637924,14.4379922357335,
14.5382958050033,14.6296411464425,14.7300085256656,14.8302468999216,14.9303870192367,
15.0319699674751,15.132021670872,15.2343702415311,15.3367188121902),
 .UNSPECIFIED.);
#1401=B_SPLINE_CURVE_WITH_KNOTS('',3,(#60036,#60037,#60038,#60039,#60040,
#60041,#60042,#60043,#60044,#60045,#60046,#60047,#60048,#60049,#60050,#60051,
#60052,#60053,#60054,#60055,#60056,#60057,#60058,#60059,#60060,#60061,#60062,
#60063,#60064,#60065,#60066,#60067,#60068,#60069,#60070,#60071,#60072,#60073,
#60074,#60075,#60076,#60077,#60078,#60079,#60080,#60081,#60082,#60083,#60084,
#60085,#60086,#60087,#60088,#60089,#60090,#60091,#60092,#60093,#60094,#60095,
#60096,#60097,#60098,#60099,#60100,#60101,#60102,#60103,#60104,#60105,#60106,
#60107,#60108,#60109,#60110,#60111,#60112,#60113,#60114,#60115,#60116,#60117,
#60118,#60119,#60120,#60121,#60122,#60123,#60124,#60125,#60126,#60127,#60128,
#60129,#60130,#60131,#60132,#60133,#60134,#60135,#60136,#60137,#60138,#60139,
#60140,#60141,#60142,#60143,#60144,#60145,#60146,#60147,#60148,#60149,#60150,
#60151,#60152,#60153,#60154,#60155,#60156,#60157,#60158,#60159,#60160,#60161,
#60162,#60163,#60164,#60165,#60166,#60167,#60168,#60169,#60170,#60171,#60172,
#60173,#60174,#60175,#60176,#60177,#60178,#60179,#60180,#60181,#60182,#60183,
#60184,#60185,#60186,#60187,#60188,#60189,#60190,#60191,#60192,#60193,#60194,
#60195,#60196,#60197,#60198,#60199,#60200,#60201,#60202,#60203,#60204,#60205,
#60206,#60207,#60208,#60209,#60210,#60211,#60212,#60213,#60214,#60215,#60216,
#60217,#60218,#60219),.UNSPECIFIED.,.F.,.F.,(4,2,2,2,2,2,2,2,2,2,2,2,2,
2,2,2,2,2,2,2,2,2,2,2,2,2,2,2,2,2,2,2,2,2,2,2,2,2,2,2,2,2,2,2,2,2,2,2,2,
2,2,2,2,2,2,2,2,2,2,2,2,2,2,2,2,2,2,2,2,2,2,2,2,2,2,2,2,2,2,2,2,2,2,2,2,
2,2,2,2,2,2,4),(-1.42848528216476,-1.42739208805283,-1.40622437849851,-1.37846524486598,
-1.34657535696718,-1.33883007564381,-1.33489574589015,-1.33162098640515,
-1.32724990685484,-1.31707848245199,-1.30184135568175,-1.2440054143437,
-1.22640650465069,-1.21930244668961,-1.21340903375455,-1.20728796914555,
-1.19797336948744,-1.16486381749814,-1.13832634160604,-1.10687028411865,
-1.09914870424514,-1.09521904201124,-1.0919435878892,-1.0875655697369,-1.07735263012905,
-1.06202631501776,-1.02701163633883,-0.99072024806915,-0.981091898523054,
-0.974907304539464,-0.968985415790711,-0.960729553647196,-0.93895219195785,
-0.902576709035968,-0.867259014621424,-0.859527123122242,-0.85559532311957,
-0.852649105374209,-0.848472133247894,-0.839432498748516,-0.82652740309081,
-0.781966379937639,-0.750621313112192,-0.74121096101936,-0.735070976584003,
-0.72912287543821,-0.720713336379773,-0.697669608872822,-0.655842253620788,
-0.624860267805108,-0.618726418991694,-0.615124692485654,-0.611749712508817,
-0.606697270805978,-0.59153848349238,-0.526698428947319,-0.507822294607592,
-0.500570464141505,-0.495179109831771,-0.489204942127855,-0.480653259324066,
-0.45636568118876,-0.409544142972789,-0.384772235321615,-0.378832639248688,
-0.37527212144002,-0.371868856187233,-0.366677083966318,-0.350238001381969,
-0.313600705714356,-0.275411889141533,-0.263978910450126,-0.257359804474307,
-0.251621122789868,-0.244348652964047,-0.229148024112924,-0.208004865655459,
-0.180208760771186,-0.148302160491255,-0.140555510837425,-0.136620566999789,
-0.133347468785993,-0.128980844388615,-0.118823328013448,-0.0841312902037792,
-0.0601569568124256,-0.0311100578728027,-0.0219411437467501,-0.0164602522482374,
-0.0109348595217452,-0.00583149434787779,-0.000697598800115113),
 .UNSPECIFIED.);
#1402=B_SPLINE_CURVE_WITH_KNOTS('',3,(#60220,#60221,#60222,#60223,#60224,
#60225,#60226,#60227,#60228,#60229,#60230,#60231,#60232),.UNSPECIFIED.,
 .F.,.F.,(4,3,3,3,4),(15.3376015162611,15.4459524370878,15.5540381009166,
15.6617322199476,15.7079632677065),.UNSPECIFIED.);
#1403=B_SPLINE_CURVE_WITH_KNOTS('',3,(#60234,#60235,#60236,#60237,#60238,
#60239,#60240,#60241,#60242,#60243,#60244,#60245,#60246),.UNSPECIFIED.,
 .F.,.F.,(4,3,3,3,4),(15.3367188121902,15.4369232050171,15.5373043800419,
15.6221162836617,15.7079632679489),.UNSPECIFIED.);
#1404=B_SPLINE_CURVE_WITH_KNOTS('',3,(#60247,#60248,#60249,#60250,#60251,
#60252,#60253,#60254,#60255,#60256,#60257,#60258,#60259,#60260,#60261,#60262,
#60263,#60264,#60265,#60266,#60267,#60268,#60269,#60270,#60271,#60272,#60273,
#60274,#60275,#60276,#60277,#60278,#60279,#60280,#60281,#60282,#60283,#60284,
#60285,#60286,#60287,#60288,#60289,#60290,#60291,#60292,#60293,#60294,#60295,
#60296,#60297,#60298,#60299,#60300,#60301,#60302,#60303,#60304,#60305,#60306,
#60307,#60308,#60309,#60310,#60311,#60312,#60313,#60314,#60315,#60316,#60317,
#60318,#60319,#60320,#60321,#60322,#60323,#60324,#60325,#60326,#60327,#60328,
#60329,#60330,#60331,#60332,#60333,#60334,#60335,#60336,#60337,#60338,#60339,
#60340,#60341,#60342,#60343,#60344,#60345,#60346,#60347,#60348,#60349,#60350,
#60351,#60352,#60353,#60354,#60355,#60356,#60357,#60358,#60359,#60360,#60361,
#60362,#60363,#60364,#60365,#60366,#60367,#60368,#60369,#60370,#60371,#60372,
#60373,#60374,#60375,#60376,#60377,#60378,#60379,#60380,#60381,#60382,#60383,
#60384,#60385,#60386,#60387,#60388,#60389,#60390,#60391,#60392,#60393,#60394,
#60395,#60396,#60397,#60398,#60399,#60400,#60401,#60402,#60403,#60404,#60405,
#60406,#60407,#60408,#60409,#60410,#60411,#60412,#60413,#60414,#60415,#60416,
#60417,#60418,#60419,#60420,#60421,#60422,#60423,#60424,#60425,#60426,#60427,
#60428,#60429,#60430),.UNSPECIFIED.,.F.,.F.,(4,3,3,3,3,3,3,3,3,3,3,3,3,
3,3,3,3,3,3,3,3,3,3,3,3,3,3,3,3,3,3,3,3,3,3,3,3,3,3,3,3,3,3,3,3,3,3,3,3,
3,3,3,3,3,3,3,3,3,3,3,3,4),(15.7079632682029,15.8069001649058,15.9078615719027,
16.0065672226263,16.105223531544,16.2038627572048,16.3065449231238,16.4053067134902,
16.504134708423,16.6031149328184,16.6145914208809,16.7148412113139,16.814948312949,
16.9149408421862,17.0148707667914,17.1147688636603,17.2146658699796,17.3146609391629,
17.4147036409847,17.5149244179969,17.6070665581,17.7073109691657,17.8074129962093,
17.9074009388044,18.0073265766264,18.1072206934565,18.2071140336548,18.3071059607411,
18.4071458022442,18.5073642341291,18.5995416953192,18.6997523138288,18.7998199110768,
18.8997726256092,18.9996625659994,19.0995205661086,19.1993774199548,19.2993325318716,
19.3993353204137,19.4995167269311,19.5920168325384,19.6922477331165,19.7923358882727,
19.8923094785937,19.9922204783603,20.0920996917434,20.1919778832322,20.2919543795833,
20.3919786118565,20.4921813122795,20.5844919697575,20.684720363369,20.7848060235463,
20.8847771493862,20.984685704486,21.0845624965693,21.1844382936973,21.2844124553515,
21.3844343818922,21.4846348531285,21.5769671069767,21.6206806328394),
 .UNSPECIFIED.);
#1405=B_SPLINE_CURVE_WITH_KNOTS('',3,(#60435,#60436,#60437,#60438,#60439,
#60440,#60441,#60442,#60443,#60444,#60445,#60446,#60447,#60448,#60449,#60450,
#60451,#60452,#60453,#60454,#60455,#60456,#60457,#60458,#60459,#60460,#60461,
#60462,#60463,#60464,#60465,#60466,#60467,#60468,#60469,#60470,#60471,#60472,
#60473,#60474,#60475,#60476,#60477,#60478,#60479,#60480,#60481,#60482,#60483,
#60484,#60485,#60486,#60487,#60488,#60489,#60490,#60491,#60492,#60493,#60494,
#60495,#60496,#60497,#60498,#60499,#60500,#60501,#60502,#60503,#60504,#60505,
#60506,#60507,#60508,#60509,#60510,#60511,#60512,#60513,#60514,#60515,#60516,
#60517,#60518,#60519,#60520,#60521,#60522,#60523,#60524,#60525,#60526,#60527,
#60528,#60529,#60530,#60531,#60532,#60533,#60534,#60535,#60536,#60537,#60538,
#60539,#60540,#60541,#60542,#60543,#60544,#60545,#60546,#60547,#60548,#60549,
#60550,#60551,#60552,#60553,#60554,#60555,#60556,#60557,#60558,#60559,#60560,
#60561,#60562,#60563,#60564,#60565,#60566,#60567,#60568,#60569,#60570,#60571,
#60572,#60573,#60574,#60575,#60576,#60577,#60578,#60579,#60580,#60581,#60582,
#60583,#60584,#60585,#60586,#60587,#60588,#60589,#60590,#60591,#60592,#60593,
#60594,#60595,#60596,#60597,#60598,#60599,#60600,#60601,#60602,#60603,#60604,
#60605,#60606,#60607,#60608,#60609,#60610,#60611,#60612,#60613,#60614,#60615,
#60616,#60617,#60618,#60619,#60620,#60621,#60622),.UNSPECIFIED.,.F.,.F.,
(4,2,2,2,2,2,2,2,2,2,2,2,2,2,2,2,2,2,2,2,2,2,2,2,2,2,2,2,2,2,2,2,2,2,2,
2,2,2,2,2,2,2,2,2,2,2,2,2,2,2,2,2,2,2,2,2,2,2,2,2,2,2,2,2,2,2,2,2,2,2,2,
2,2,2,2,2,2,2,2,2,2,2,2,2,2,2,2,2,2,2,2,2,2,4),(-2.94547660919547,-2.92715951863759,
-2.90491281398846,-2.89658309479856,-2.89065023542024,-2.88449051745253,
-2.87497678642284,-2.84188205597475,-2.79891063631364,-2.78017752241277,
-2.77477174139842,-2.77132673082468,-2.76782588801094,-2.76215869957292,
-2.74216853520164,-2.69697053561332,-2.66704132024668,-2.65795951456132,
-2.6518859347408,-2.64596039778645,-2.63734050048888,-2.61435597554483,
-2.5557181451002,-2.53996704981601,-2.53485000233545,-2.53146327982842,
-2.52833043434775,-2.52277723967755,-2.50397545608757,-2.4576406988326,
-2.42746780756053,-2.41836637106877,-2.41228870741671,-2.40636589255893,
-2.39913762629131,-2.38057510656985,-2.32369276554082,-2.30865138491331,
-2.29857321265352,-2.29421807217505,-2.2909749043216,-2.28704487873791,
-2.27931864954599,-2.24397780354891,-2.20761978748256,-2.18591629316678,
-2.17767160516265,-2.17175292792489,-2.16556747572321,-2.15592902911769,
-2.11919719196462,-2.08438688513021,-2.06918249298325,-2.05902805959242,
-2.05466039020284,-2.05138665475765,-2.04745158870617,-2.03969957014487,
-2.00767291423227,-1.97966500619704,-1.94845983158126,-1.93927952133529,
-1.93318607931048,-1.92727499095709,-1.92009479439843,-1.90198554166627,
-1.84450148839802,-1.82946409779941,-1.81938762936905,-1.81503261857501,
-1.81178928627479,-1.80785872123584,-1.80013056578035,-1.7648674211659,
-1.72853639704151,-1.71373626053258,-1.70200281033097,-1.69538864939144,
-1.68959791623671,-1.68229926328989,-1.66693457796284,-1.59028407420276,
-1.57982636048455,-1.57540866172712,-1.57215880505185,-1.56826987461383,
-1.56097542836035,-1.51819938272134,-1.47364490395837,-1.46222720235396,
-1.45561289864828,-1.44987621721666,-1.44260354589539,-1.42848528216476),
 .UNSPECIFIED.);
#1406=B_SPLINE_CURVE_WITH_KNOTS('',3,(#60624,#60625,#60626,#60627,#60628,
#60629,#60630,#60631,#60632,#60633,#60634,#60635,#60636),.UNSPECIFIED.,
 .F.,.F.,(4,3,3,3,4),(21.6206806328394,21.7304850229789,21.8399813708388,
21.9490014055409,21.9911485751285),.UNSPECIFIED.);
#1407=B_SPLINE_CURVE_WITH_KNOTS('',3,(#60637,#60638,#60639,#60640,#60641,
#60642,#60643,#60644,#60645,#60646),.UNSPECIFIED.,.F.,.F.,(4,1,1,1,1,1,
1,4),(21.9911485751285,22.5694422441959,23.5619173814151,24.5543925186342,
25.5468676558534,26.5393427930726,27.5318179302917,27.9042171936241),
 .UNSPECIFIED.);
#1408=B_SPLINE_CURVE_WITH_KNOTS('',3,(#60652,#60653,#60654,#60655,#60656,
#60657,#60658,#60659,#60660,#60661),.UNSPECIFIED.,.F.,.F.,(4,1,1,1,1,1,
1,4),(28.2743423585487,29.1675934276459,30.1600685648651,31.1525437020842,
32.1450188393034,33.1374939765226,34.1299691137418,34.1871485763958),
 .UNSPECIFIED.);
#1409=B_SPLINE_CURVE_WITH_KNOTS('',3,(#60662,#60663,#60664,#60665,#60666,
#60667,#60668,#60669,#60670,#60671,#60672,#60673,#60674,#60675,#60676,#60677,
#60678,#60679),.UNSPECIFIED.,.F.,.F.,(4,2,2,2,2,2,2,2,4),(-3.03482422073094,
-3.02093589767063,-3.01648477335601,-3.01320992380041,-3.01000493469182,
-3.0061869062627,-2.99921991151881,-2.96963288453497,-2.94547660919547),
 .UNSPECIFIED.);
#1410=B_SPLINE_CURVE_WITH_KNOTS('',3,(#60681,#60682,#60683,#60684),
 .UNSPECIFIED.,.F.,.F.,(4,4),(27.9042171936241,28.2743338823081),
 .UNSPECIFIED.);
#1411=B_SPLINE_CURVE_WITH_KNOTS('',3,(#60685,#60686,#60687,#60688,#60689,
#60690,#60691,#60692,#60693,#60694,#60695,#60696,#60697,#60698,#60699,#60700,
#60701,#60702,#60703,#60704,#60705,#60706,#60707,#60708,#60709,#60710,#60711,
#60712,#60713,#60714,#60715,#60716,#60717,#60718,#60719,#60720,#60721,#60722,
#60723,#60724,#60725,#60726,#60727,#60728,#60729,#60730,#60731,#60732,#60733,
#60734,#60735,#60736,#60737,#60738,#60739,#60740,#60741,#60742,#60743,#60744,
#60745,#60746,#60747,#60748,#60749,#60750,#60751,#60752,#60753,#60754,#60755,
#60756,#60757,#60758,#60759,#60760,#60761,#60762,#60763,#60764,#60765,#60766,
#60767,#60768,#60769,#60770,#60771,#60772,#60773,#60774,#60775,#60776,#60777,
#60778,#60779,#60780,#60781,#60782,#60783,#60784,#60785,#60786,#60787,#60788,
#60789,#60790,#60791,#60792,#60793,#60794,#60795,#60796,#60797,#60798,#60799,
#60800,#60801,#60802,#60803,#60804,#60805,#60806,#60807,#60808,#60809,#60810,
#60811,#60812,#60813,#60814,#60815,#60816,#60817,#60818,#60819,#60820,#60821,
#60822,#60823,#60824,#60825,#60826,#60827,#60828,#60829,#60830,#60831,#60832,
#60833,#60834,#60835,#60836,#60837,#60838,#60839,#60840,#60841,#60842,#60843,
#60844,#60845,#60846,#60847,#60848,#60849,#60850,#60851,#60852,#60853,#60854,
#60855,#60856,#60857,#60858,#60859,#60860,#60861,#60862,#60863,#60864,#60865,
#60866,#60867,#60868),.UNSPECIFIED.,.F.,.F.,(4,2,2,2,2,2,2,2,2,2,2,2,2,
2,2,2,2,2,2,2,2,2,2,2,2,2,2,2,2,2,2,2,2,2,2,2,2,2,2,2,2,2,2,2,2,2,2,2,2,
2,2,2,2,2,2,2,2,2,2,2,2,2,2,2,2,2,2,2,2,2,2,2,2,2,2,2,2,2,2,2,2,2,2,2,2,
2,2,2,2,2,2,4),(-3.03525809594091,-2.99530510455854,-2.98648465697967,-2.98153112966352,
-2.97715190408744,-2.97387772211438,-2.96995227776847,-2.96224708361332,
-2.92617184921776,-2.8900353978971,-2.87551811930468,-2.86416755335944,
-2.86355662129243,-2.86297158538743,-2.86240273472369,-2.86184056032287,
-2.8557304818867,-2.8498335138595,-2.84270782976043,-2.82495866459474,-2.76759922190144,
-2.75217560558485,-2.74191930528804,-2.7375352662932,-2.73426049483457,
-2.73033801647843,-2.72288007573829,-2.67560075104725,-2.64679427291659,
-2.62812637763949,-2.62029788425523,-2.61444593320707,-2.6081142940785,
-2.59775935510852,-2.53896765011272,-2.50862575543308,-2.50095197670286,
-2.49703243920211,-2.4937570172262,-2.48944373613989,-2.47973881677227,
-2.4288368497774,-2.40442990828462,-2.38766264458717,-2.3801286386934,-2.374314951281,
-2.36784332257269,-2.35680862029876,-2.28743411801071,-2.2724777429273,
-2.26243907974251,-2.25809030174714,-2.25481791905695,-2.25086890059642,
-2.24328603372607,-2.2069682738424,-2.17025447330345,-2.14947286402478,
-2.14134712036435,-2.13544814062835,-2.12922483550164,-2.1194017489489,
-2.0790861103925,-2.04081829647575,-2.02466899008175,-2.01950918265168,
-2.01611389187263,-2.0125466334586,-2.00657231114134,-1.98087515647114,
-1.9348634158103,-1.91076585898542,-1.9022365321442,-1.89626734347457,-1.89015886705032,
-1.88090381567415,-1.85098553563016,-1.80491683310782,-1.78561302608664,
-1.7801580636809,-1.77670231403423,-1.77363404125072,-1.7684249814729,-1.75308146713379,
-1.70813827133112,-1.68471288182818,-1.66840178175483,-1.66094215067751,
-1.6551360838361,-1.648621777786,-1.63738098762808,-1.60771239371903),
 .UNSPECIFIED.);
#1412=B_SPLINE_CURVE_WITH_KNOTS('',3,(#60874,#60875,#60876,#60877,#60878,
#60879,#60880,#60881,#60882,#60883,#60884,#60885,#60886,#60887,#60888,#60889,
#60890,#60891,#60892,#60893,#60894,#60895,#60896,#60897,#60898,#60899,#60900,
#60901,#60902,#60903,#60904,#60905,#60906,#60907,#60908,#60909,#60910,#60911,
#60912,#60913,#60914,#60915,#60916,#60917,#60918,#60919,#60920,#60921,#60922,
#60923,#60924,#60925,#60926,#60927,#60928,#60929,#60930,#60931,#60932,#60933,
#60934,#60935,#60936,#60937,#60938,#60939,#60940,#60941,#60942,#60943,#60944,
#60945,#60946,#60947,#60948,#60949,#60950,#60951,#60952,#60953,#60954,#60955,
#60956,#60957,#60958,#60959,#60960,#60961,#60962,#60963,#60964,#60965,#60966,
#60967,#60968,#60969,#60970,#60971,#60972,#60973,#60974,#60975,#60976,#60977,
#60978,#60979,#60980,#60981,#60982,#60983,#60984,#60985,#60986,#60987,#60988,
#60989,#60990,#60991,#60992,#60993,#60994,#60995,#60996,#60997,#60998,#60999,
#61000,#61001,#61002,#61003,#61004,#61005,#61006,#61007,#61008,#61009,#61010,
#61011,#61012,#61013,#61014,#61015,#61016,#61017,#61018,#61019,#61020,#61021,
#61022,#61023,#61024,#61025,#61026,#61027,#61028,#61029,#61030,#61031,#61032,
#61033,#61034,#61035,#61036,#61037,#61038,#61039,#61040,#61041,#61042,#61043,
#61044,#61045,#61046,#61047,#61048,#61049),.UNSPECIFIED.,.F.,.F.,(4,2,2,
2,2,2,2,2,2,2,2,2,2,2,2,2,2,2,2,2,2,2,2,2,2,2,2,2,2,2,2,2,2,2,2,2,2,2,2,
2,2,2,2,2,2,2,2,2,2,2,2,2,2,2,2,2,2,2,2,2,2,2,2,2,2,2,2,2,2,2,2,2,2,2,2,
2,2,2,2,2,2,2,2,2,2,2,2,4),(-1.42901813234523,-1.40868918639051,-1.38082821385019,
-1.34889189041069,-1.341142083987,-1.33720611739261,-1.33393038528493,-1.32955850340953,
-1.31938728428427,-1.30415255338032,-1.24562145912397,-1.22847768934837,
-1.22144371224105,-1.21556573631506,-1.20941650070952,-1.19996771526432,
-1.16466995722726,-1.1189272236897,-1.10434979953971,-1.09923082955223,
-1.09617765291173,-1.09269654495528,-1.08712798846818,-1.06640069741722,
-1.01073415151283,-0.99002340742071,-0.981689381315718,-0.975811935944632,
-0.969661929679125,-0.960209201978839,-0.924839737117272,-0.878821125394451,
-0.86452435312988,-0.859440316816066,-0.856092115270448,-0.852509918715487,
-0.846470918604121,-0.816991460743075,-0.756380869664702,-0.745158785979234,
-0.738585376845186,-0.733366636134898,-0.726290996277387,-0.71218053347784,
-0.693147610310051,-0.663078028557834,-0.627038852563289,-0.620813755110829,
-0.617191859349139,-0.61382648714436,-0.608828812233951,-0.594153733754266,
-0.523948374676302,-0.5080485897618,-0.500656679893208,-0.494855961053586,
-0.488298055215494,-0.47684927032268,-0.439193070240063,-0.39611072986621,
-0.384253838712058,-0.379505126310676,-0.376182750311603,-0.372462110122931,
-0.365769912031505,-0.357166039822251,-0.336462832183888,-0.284363510761708,
-0.268386507001057,-0.260981645092294,-0.255179790536097,-0.248630064165351,
-0.237220994085274,-0.199872769812796,-0.157423527947901,-0.144826906813248,
-0.13996128996307,-0.136652652997935,-0.132993966334978,-0.126595094124896,
-0.118483480024856,-0.0613115477139129,-0.0328598753366852,-0.0237337666203509,
-0.0182573289756244,-0.012733045052215,-0.00686466933992766,-0.000717267781909915),
 .UNSPECIFIED.);
#1413=B_SPLINE_CURVE_WITH_KNOTS('',3,(#61050,#61051,#61052,#61053),
 .UNSPECIFIED.,.F.,.F.,(4,4),(34.1871485763958,34.5575142542),
 .UNSPECIFIED.);
#1414=B_SPLINE_CURVE_WITH_KNOTS('',3,(#61054,#61055,#61056,#61057,#61058,
#61059,#61060,#61061,#61062,#61063,#61064,#61065,#61066,#61067,#61068,#61069,
#61070,#61071,#61072,#61073,#61074,#61075,#61076,#61077,#61078,#61079,#61080,
#61081,#61082,#61083,#61084,#61085,#61086,#61087,#61088,#61089,#61090,#61091,
#61092,#61093,#61094,#61095,#61096,#61097,#61098,#61099,#61100,#61101,#61102,
#61103,#61104,#61105,#61106,#61107,#61108,#61109,#61110,#61111,#61112,#61113,
#61114,#61115,#61116,#61117,#61118,#61119,#61120,#61121,#61122,#61123,#61124,
#61125,#61126,#61127,#61128,#61129,#61130,#61131,#61132,#61133,#61134,#61135,
#61136,#61137,#61138,#61139,#61140,#61141,#61142,#61143,#61144,#61145,#61146,
#61147,#61148,#61149,#61150,#61151,#61152,#61153,#61154,#61155,#61156,#61157,
#61158,#61159,#61160,#61161,#61162,#61163,#61164,#61165,#61166,#61167,#61168,
#61169,#61170,#61171,#61172,#61173,#61174,#61175,#61176,#61177,#61178,#61179,
#61180,#61181,#61182,#61183,#61184,#61185,#61186,#61187,#61188,#61189,#61190,
#61191,#61192,#61193,#61194,#61195,#61196,#61197,#61198,#61199,#61200,#61201,
#61202,#61203,#61204,#61205,#61206,#61207,#61208,#61209,#61210,#61211,#61212,
#61213,#61214,#61215,#61216,#61217,#61218,#61219,#61220,#61221,#61222,#61223,
#61224,#61225,#61226,#61227,#61228,#61229,#61230,#61231,#61232,#61233,#61234,
#61235,#61236,#61237,#61238,#61239,#61240,#61241,#61242,#61243,#61244,#61245,
#61246,#61247,#61248,#61249,#61250,#61251),.UNSPECIFIED.,.F.,.F.,(4,2,2,
2,2,2,2,2,2,2,2,2,2,2,2,2,2,2,2,2,2,2,2,2,2,2,2,2,2,2,2,2,2,2,2,2,2,2,2,
2,2,2,2,2,2,2,2,2,2,2,2,2,2,2,2,2,2,2,2,2,2,2,2,2,2,2,2,2,2,2,2,2,2,2,2,
2,2,2,2,2,2,2,2,2,2,2,2,2,2,2,2,2,2,2,2,2,2,2,4),(-1.60771239371903,-1.58563232463443,
-1.54840195198594,-1.54161572852876,-1.53787602866725,-1.5345611530345,
-1.52985711170048,-1.51828242587957,-1.49938915117538,-1.43588506213879,
-1.42514860532117,-1.41873759394151,-1.4129082316278,-1.40525211849731,
-1.38772508560634,-1.36162369375314,-1.32186689920125,-1.30585903271183,
-1.30057415911958,-1.29749198579621,-1.29405362894285,-1.28868192036419,
-1.27034209092257,-1.22935250564103,-1.19401513014059,-1.18441277683645,
-1.17823426950886,-1.17231077052991,-1.1640403669311,-1.14214020236068,
-1.10581254455995,-1.07059933557428,-1.0628655918787,-1.05893380673687,
-1.05565923122297,-1.05128599563974,-1.0410996057581,-1.0258301172431,-0.971066521313685,
-0.951219963718141,-0.943021165674417,-0.937168388556777,-0.930982541490285,
-0.921344042240624,-0.881994264506287,-0.841803736747118,-0.826361613906376,
-0.821140750775315,-0.818070249532416,-0.814617069181905,-0.809174946846298,
-0.790022969790914,-0.74479562126903,-0.714154249915272,-0.70478946959568,
-0.69865879577729,-0.692704804882873,-0.684261284134163,-0.660925791722852,
-0.618006043352791,-0.588440109606404,-0.582325987843649,-0.578728568103269,
-0.575351456241607,-0.570286861002946,-0.555017707422506,-0.491431433983151,
-0.471733119521139,-0.463564449598397,-0.457658213014066,-0.451448529497508,
-0.441692850745728,-0.398778972855953,-0.352020667522152,-0.343940377447059,
-0.339941187063523,-0.337000583153999,-0.332903517818516,-0.324303506431401,
-0.31225617506193,-0.274048395568041,-0.235500715995794,-0.225757784064002,
-0.219550477930858,-0.214058167563003,-0.213409934812446,-0.212873479311974,
-0.212390648398338,-0.211928280322896,-0.211462625087586,-0.205030353579788,
-0.19554681253086,-0.167410218601886,-0.121909949769982,-0.107091260004682,
-0.101943963336318,-0.0988865612075943,-0.0954147961160319,-0.0901927161961946),
 .UNSPECIFIED.);
#1415=B_SPLINE_CURVE_WITH_KNOTS('',3,(#61256,#61257,#61258,#61259,#61260,
#61261,#61262,#61263,#61264,#61265,#61266,#61267,#61268,#61269,#61270,#61271,
#61272,#61273,#61274,#61275,#61276,#61277,#61278,#61279,#61280,#61281,#61282,
#61283,#61284,#61285,#61286,#61287,#61288,#61289,#61290,#61291,#61292,#61293,
#61294,#61295,#61296,#61297,#61298,#61299,#61300,#61301,#61302,#61303,#61304,
#61305,#61306,#61307,#61308,#61309,#61310,#61311,#61312,#61313,#61314,#61315,
#61316,#61317,#61318,#61319,#61320,#61321,#61322,#61323,#61324,#61325,#61326,
#61327,#61328,#61329,#61330,#61331,#61332,#61333,#61334,#61335,#61336,#61337,
#61338,#61339,#61340,#61341,#61342,#61343,#61344,#61345,#61346,#61347,#61348,
#61349,#61350,#61351,#61352,#61353,#61354,#61355,#61356,#61357,#61358,#61359,
#61360,#61361,#61362,#61363,#61364,#61365,#61366,#61367,#61368,#61369,#61370,
#61371,#61372,#61373,#61374,#61375,#61376,#61377,#61378,#61379,#61380,#61381,
#61382,#61383,#61384,#61385,#61386,#61387,#61388,#61389,#61390,#61391,#61392,
#61393,#61394,#61395,#61396,#61397,#61398,#61399,#61400,#61401,#61402,#61403,
#61404,#61405,#61406,#61407,#61408,#61409,#61410,#61411,#61412,#61413,#61414,
#61415,#61416,#61417,#61418,#61419,#61420,#61421,#61422,#61423,#61424,#61425,
#61426,#61427,#61428,#61429,#61430,#61431,#61432,#61433,#61434,#61435,#61436,
#61437,#61438,#61439,#61440,#61441,#61442,#61443,#61444,#61445,#61446,#61447,
#61448,#61449),.UNSPECIFIED.,.F.,.F.,(4,2,2,2,2,2,2,2,2,2,2,2,2,2,2,2,2,
2,2,2,2,2,2,2,2,2,2,2,2,2,2,2,2,2,2,2,2,2,2,2,2,2,2,2,2,2,2,2,2,2,2,2,2,
2,2,2,2,2,2,2,2,2,2,2,2,2,2,2,2,2,2,2,2,2,2,2,2,2,2,2,2,2,2,2,2,2,2,2,2,
2,2,2,2,2,2,2,4),(-2.94656220223364,-2.93107157250197,-2.90797912015355,
-2.89956315218436,-2.89361301984311,-2.88747302235605,-2.87806691297442,
-2.84680988552935,-2.80210780122725,-2.78918075954208,-2.78013051841647,
-2.77595108272143,-2.77300427068659,-2.769073291396,-2.76134674760497,-2.72586603616624,
-2.68944658537902,-2.66786572504297,-2.65963455908693,-2.65371651274769,
-2.64826260731479,-2.63926585838981,-2.61243376898799,-2.56330187262677,
-2.54348931356536,-2.53799166875045,-2.53452607891713,-2.53146302746631,
-2.52628695963156,-2.51123270060586,-2.46600501977972,-2.43085657052876,
-2.42141802421395,-2.41527132918213,-2.4093928232568,-2.40235459270603,
-2.38486164014381,-2.32665822285386,-2.31141090628959,-2.30123502262828,
-2.29686257175623,-2.29358707646706,-2.28965212164009,-2.28190641247196,
-2.25002586350779,-2.22226666793862,-2.19066748122149,-2.1814552974564,
-2.17535354957512,-2.16944379043507,-2.16227684142528,-2.14427713905496,
-2.08659909619292,-2.07155602553697,-2.06147548744532,-2.05711855501576,
-2.05387373706919,-2.04994131688916,-2.04220931722343,-2.00694322932635,
-1.97060118404076,-1.94879031191285,-1.94052920568066,-1.93460536335289,
-1.92842030129443,-1.91879467064947,-1.88279554603591,-1.84737247307824,
-1.83204383725341,-1.82182992023604,-1.8174510865857,-1.81417488392062,
-1.81024405432679,-1.80252001829571,-1.77103674633988,-1.74439987043636,
-1.71143818871409,-1.70213193664404,-1.69601123128642,-1.69011443012222,
-1.68166983281236,-1.66016213402194,-1.60536671541315,-1.59139282959725,
-1.58182324519615,-1.57755228477352,-1.57459623208069,-1.57073230872319,
-1.56355882476752,-1.51875550452783,-1.47603426478969,-1.46459152267197,
-1.45797059449349,-1.45223271153204,-1.44496454922729,-1.42978686594534,
-1.42901813234523),.UNSPECIFIED.);
#1416=B_SPLINE_CURVE_WITH_KNOTS('',3,(#61451,#61452,#61453,#61454,#61455,
#61456,#61457,#61458),.UNSPECIFIED.,.F.,.F.,(4,2,2,4),(-0.0901927161961946,
-0.0898859350082424,-0.0696626742519121,-0.00069517407964766),
 .UNSPECIFIED.);
#1417=B_SPLINE_CURVE_WITH_KNOTS('',3,(#61459,#61460,#61461,#61462,#61463,
#61464,#61465,#61466,#61467,#61468,#61469,#61470,#61471,#61472,#61473,#61474,
#61475,#61476,#61477,#61478,#61479,#61480,#61481,#61482,#61483,#61484,#61485,
#61486,#61487,#61488,#61489,#61490,#61491,#61492,#61493,#61494,#61495,#61496,
#61497,#61498,#61499,#61500,#61501,#61502,#61503,#61504,#61505,#61506,#61507,
#61508,#61509,#61510,#61511,#61512,#61513,#61514,#61515,#61516,#61517,#61518,
#61519,#61520,#61521,#61522,#61523,#61524,#61525,#61526,#61527,#61528,#61529,
#61530,#61531,#61532,#61533,#61534,#61535,#61536,#61537,#61538,#61539,#61540,
#61541,#61542,#61543,#61544,#61545,#61546,#61547,#61548,#61549,#61550,#61551,
#61552,#61553,#61554,#61555,#61556,#61557,#61558,#61559,#61560,#61561,#61562,
#61563,#61564,#61565,#61566,#61567,#61568,#61569,#61570,#61571,#61572,#61573,
#61574,#61575,#61576,#61577,#61578,#61579,#61580,#61581,#61582,#61583,#61584,
#61585,#61586,#61587,#61588,#61589,#61590,#61591,#61592,#61593,#61594,#61595,
#61596,#61597,#61598,#61599,#61600,#61601,#61602,#61603,#61604,#61605,#61606,
#61607,#61608,#61609,#61610,#61611,#61612,#61613,#61614,#61615,#61616,#61617,
#61618,#61619,#61620,#61621,#61622,#61623,#61624,#61625,#61626,#61627,#61628,
#61629,#61630,#61631,#61632,#61633,#61634,#61635,#61636),.UNSPECIFIED.,
 .F.,.F.,(4,2,2,2,2,2,2,2,2,2,2,2,2,2,2,2,2,2,2,2,2,2,2,2,2,2,2,2,2,2,2,
2,2,2,2,2,2,2,2,2,2,2,2,2,2,2,2,2,2,2,2,2,2,2,2,2,2,2,2,2,2,2,2,2,2,2,2,
2,2,2,2,2,2,2,2,2,2,2,2,2,2,2,2,2,2,2,2,2,4),(-3.03528425599135,-3.02396005249311,
-3.01821358683809,-3.01268720184321,-3.00720482041017,-2.9980336783293,
-2.96896968647659,-2.91266369537032,-2.90953754827863,-2.89989664775877,
-2.89561540810208,-2.89266009869233,-2.88880857383738,-2.88168501434852,
-2.83631742787498,-2.79315532775536,-2.7821219362015,-2.77565119907522,
-2.76983832760626,-2.76243075545287,-2.74594381814187,-2.69436048568999,
-2.66411404658158,-2.65805087440207,-2.65446504640402,-2.65112268622414,
-2.64606135836705,-2.63192637368942,-2.5907630621108,-2.55335300487471,
-2.54241432349103,-2.53596270165716,-2.53014505464891,-2.52270124197044,
-2.50599231645271,-2.44587343122491,-2.43085503741057,-2.42078758064652,
-2.41643436596033,-2.41316199265588,-2.40921708739238,-2.40165258090245,
-2.36512766873907,-2.32834068630927,-2.30775772511052,-2.29965912861901,
-2.293765156788,-2.28753392246816,-2.27766950112804,-2.23660984209929,-2.20052138600566,
-2.18326929602024,-2.17799890007728,-2.17458178139168,-2.17148161467711,
-2.1660987422454,-2.14916956010022,-2.10573551548009,-2.07107094692933,
-2.0616631535585,-2.05552465527732,-2.04964565738719,-2.04259683073055,
-2.02501647593209,-1.96660132232056,-1.95156915718805,-1.94149507868237,
-1.93714063149586,-1.93389759071763,-1.92996737037985,-1.92224003247172,
-1.89064639072072,-1.86367457468669,-1.83113425382627,-1.82185942249268,
-1.81574723687957,-1.80984992834648,-1.8027259133918,-1.78499279174484,
-1.72694380532815,-1.71190772053385,-1.7018315967207,-1.69747662867949,
-1.69420376659426,-1.69025928797621,-1.68269818608245,-1.64605070440242,
-1.60921153310692,-1.60751603659748),.UNSPECIFIED.);
#1418=B_SPLINE_CURVE_WITH_KNOTS('',3,(#61642,#61643,#61644,#61645,#61646,
#61647,#61648,#61649,#61650,#61651,#61652,#61653,#61654,#61655,#61656,#61657,
#61658,#61659,#61660,#61661,#61662,#61663,#61664,#61665,#61666,#61667,#61668,
#61669,#61670,#61671,#61672,#61673,#61674,#61675,#61676,#61677,#61678,#61679,
#61680,#61681,#61682,#61683,#61684,#61685,#61686,#61687,#61688,#61689,#61690,
#61691,#61692,#61693,#61694,#61695,#61696,#61697,#61698,#61699,#61700,#61701,
#61702,#61703,#61704,#61705,#61706,#61707,#61708,#61709,#61710,#61711,#61712,
#61713,#61714,#61715,#61716,#61717,#61718,#61719,#61720,#61721,#61722,#61723,
#61724,#61725,#61726,#61727,#61728,#61729,#61730,#61731,#61732,#61733,#61734,
#61735,#61736,#61737,#61738,#61739,#61740,#61741,#61742,#61743,#61744,#61745,
#61746,#61747,#61748,#61749,#61750,#61751,#61752,#61753,#61754,#61755,#61756,
#61757,#61758,#61759,#61760,#61761,#61762,#61763,#61764,#61765,#61766,#61767,
#61768,#61769,#61770,#61771,#61772,#61773,#61774,#61775,#61776,#61777,#61778,
#61779,#61780,#61781,#61782,#61783,#61784,#61785,#61786,#61787,#61788,#61789,
#61790,#61791,#61792,#61793,#61794,#61795,#61796,#61797,#61798,#61799,#61800,
#61801,#61802,#61803,#61804,#61805,#61806,#61807,#61808,#61809,#61810,#61811,
#61812,#61813,#61814,#61815,#61816,#61817,#61818,#61819,#61820,#61821,#61822,
#61823,#61824,#61825,#61826,#61827,#61828,#61829,#61830,#61831,#61832,#61833,
#61834,#61835,#61836,#61837,#61838,#61839,#61840,#61841,#61842,#61843,#61844,
#61845,#61846,#61847,#61848,#61849,#61850,#61851,#61852,#61853,#61854,#61855,
#61856,#61857,#61858,#61859,#61860,#61861,#61862,#61863,#61864,#61865,#61866,
#61867,#61868,#61869,#61870,#61871,#61872,#61873,#61874,#61875,#61876,#61877,
#61878,#61879,#61880,#61881,#61882,#61883,#61884,#61885),.UNSPECIFIED.,
 .F.,.F.,(4,2,2,2,2,2,2,2,2,2,2,2,2,2,2,2,2,2,2,2,2,2,2,2,2,2,2,2,2,2,2,
2,2,2,2,2,2,2,2,2,2,2,2,2,2,2,2,2,2,2,2,2,2,2,2,2,2,2,2,2,2,2,2,2,2,2,2,
2,2,2,2,2,2,2,2,2,2,2,2,2,2,2,2,2,2,2,2,2,2,2,2,2,2,2,2,2,2,2,2,2,2,2,2,
2,2,2,2,2,2,2,2,2,2,2,2,2,2,2,2,2,2,4),(-1.42845108479066,-1.42143216311403,
-1.41758627357992,-1.41462899073518,-1.41033661236475,-1.40063413152217,
-1.38638506044704,-1.32809077973996,-1.30963254464462,-1.30241329235493,
-1.29649229261596,-1.29041096578148,-1.28129322476405,-1.25092988990403,
-1.20375959232591,-1.18578806005888,-1.18030639936041,-1.17718711163717,
-1.17378764847098,-1.16860727252622,-1.1522584519666,-1.11493846960333,
-1.07414430063867,-1.0642556710435,-1.05801878957064,-1.05212596392673,
-1.0440393376434,-1.02355317112203,-0.986690161992489,-0.950047148183531,
-0.942483440886864,-0.938538274846616,-0.93526514916804,-0.930910167126929,
-0.920834734191991,-0.905801979162551,-0.848912044381502,-0.830386547693013,
-0.823161212722347,-0.81723851696378,-0.811158738900404,-0.802049809877046,
-0.77180323958155,-0.72518152112645,-0.706622602390665,-0.701090568418409,
-0.697961487151243,-0.694570508182388,-0.689433808381316,-0.673502902656044,
-0.63446189318228,-0.59460958159339,-0.584851694904917,-0.578641341993393,
-0.572734876945046,-0.564566503029301,-0.543465588412021,-0.506842146047196,
-0.470918783349053,-0.463173005355096,-0.459238741253637,-0.455964220132156,
-0.451593684452382,-0.441424450938279,-0.426191495766157,-0.368087255942739,
-0.350576365455206,-0.343536975728104,-0.337659312475759,-0.331515422549332,
-0.322085271345438,-0.287068915929982,-0.242361170518768,-0.226738444819332,
-0.221496770065138,-0.218422374284001,-0.215084828686073,-0.215047741239131,
-0.215011024064946,-0.214974615849982,-0.214938457914119,-0.214902493739294,
-0.214866668611279,-0.214830929268752,-0.214795223557888,-0.21475950011054,
-0.2147237079959,-0.214687796485903,-0.214651714799997,-0.21461541177425,
-0.214578835577679,-0.214541933469283,-0.214504651522058,-0.214466934257536,
-0.214428724394927,-0.214389962543958,-0.214350586853511,-0.214310532635308,
-0.214269731962686,-0.214228113321684,-0.214185601096374,-0.214142115101583,
-0.214097570059814,-0.214051874961794,-0.214004932461522,-0.2139566381116,
-0.213906879592602,-0.213855535806203,-0.21380247587604,-0.213747558012905,
-0.213690628277317,-0.209633536400428,-0.203161230754096,-0.18992986547316,
-0.142565256877873,-0.114263719858855,-0.10501542840349,-0.0989078195222654,
-0.0929367070542661,-0.08439970750449,-0.0602410135355151,-0.000695333887311579),
 .UNSPECIFIED.);
#1419=B_SPLINE_CURVE_WITH_KNOTS('',3,(#61886,#61887,#61888,#61889,#61890,
#61891,#61892,#61893,#61894,#61895,#61896,#61897,#61898,#61899,#61900,#61901,
#61902,#61903),.UNSPECIFIED.,.F.,.F.,(4,2,2,2,2,2,2,2,4),(-3.03596232598265,
-3.02651077198456,-3.0199354130703,-3.01655933429411,-3.0134607107987,-3.00984676424624,
-3.00365792931449,-2.97487168403078,-2.94656220223364),.UNSPECIFIED.);
#1420=B_SPLINE_CURVE_WITH_KNOTS('',3,(#61904,#61905,#61906,#61907,#61908,
#61909,#61910,#61911,#61912,#61913,#61914,#61915,#61916,#61917,#61918,#61919,
#61920,#61921,#61922,#61923,#61924,#61925,#61926,#61927,#61928,#61929,#61930,
#61931,#61932,#61933,#61934,#61935,#61936,#61937,#61938,#61939,#61940,#61941,
#61942,#61943,#61944,#61945,#61946,#61947,#61948,#61949,#61950,#61951,#61952,
#61953,#61954,#61955,#61956,#61957,#61958,#61959,#61960,#61961,#61962,#61963,
#61964,#61965,#61966,#61967,#61968,#61969,#61970,#61971,#61972,#61973,#61974,
#61975,#61976,#61977,#61978,#61979,#61980,#61981,#61982,#61983,#61984,#61985,
#61986,#61987,#61988,#61989,#61990,#61991,#61992,#61993,#61994,#61995,#61996,
#61997,#61998,#61999,#62000,#62001,#62002,#62003,#62004,#62005,#62006,#62007,
#62008,#62009,#62010,#62011,#62012,#62013,#62014,#62015,#62016,#62017,#62018,
#62019,#62020,#62021,#62022,#62023,#62024,#62025,#62026,#62027,#62028,#62029,
#62030,#62031,#62032,#62033,#62034,#62035,#62036,#62037,#62038,#62039,#62040,
#62041,#62042,#62043,#62044,#62045,#62046,#62047,#62048,#62049,#62050,#62051,
#62052,#62053,#62054,#62055,#62056,#62057,#62058,#62059,#62060,#62061,#62062,
#62063,#62064,#62065,#62066,#62067,#62068,#62069,#62070,#62071,#62072,#62073,
#62074,#62075,#62076,#62077,#62078,#62079,#62080,#62081,#62082,#62083,#62084,
#62085,#62086,#62087,#62088,#62089,#62090,#62091,#62092,#62093),
 .UNSPECIFIED.,.F.,.F.,(4,2,2,2,2,2,2,2,2,2,2,2,2,2,2,2,2,2,2,2,2,2,2,2,
2,2,2,2,2,2,2,2,2,2,2,2,2,2,2,2,2,2,2,2,2,2,2,2,2,2,2,2,2,2,2,2,2,2,2,2,
2,2,2,2,2,2,2,2,2,2,2,2,2,2,2,2,2,2,2,2,2,2,2,2,2,2,2,2,2,2,2,2,2,2,4),
(-1.60751603659748,-1.58874532652916,-1.58066179055868,-1.57476972114249,
-1.56853232732708,-1.55864024971192,-1.51777931087869,-1.47422828083003,
-1.46293308922925,-1.45872534371252,-1.45538855481355,-1.4517907796266,
-1.44567437905709,-1.41366240458484,-1.35715132647057,-1.3451507595116,
-1.33841407579451,-1.332635186044,-1.325505690886,-1.31109072274315,-1.30042488523193,
-1.26413623461994,-1.22902332242951,-1.22128859974243,-1.21735681476033,
-1.21408253849505,-1.20971009489354,-1.19952721966985,-1.18426474873691,
-1.12895382027006,-1.10947073894241,-1.10215417084762,-1.09674867171552,
-1.09079194128018,-1.08233060087535,-1.05883566297541,-1.01529488135641,
-0.986525026668314,-0.980431659506431,-0.976838923648086,-0.973459632044182,
-0.968382285070097,-0.952995474299193,-0.890659216879083,-0.870185227995624,
-0.861887667860104,-0.856018736833323,-0.849862886221126,-0.840370460046385,
-0.804199345277004,-0.754971655366581,-0.743821264141982,-0.739626202596394,
-0.736292707079823,-0.732689325679836,-0.726546268582389,-0.693476016035368,
-0.634875141860273,-0.624498461368961,-0.618161942184082,-0.612310847809796,
-0.604491688982575,-0.585891656639177,-0.557251531090971,-0.51053376052804,
-0.502422381453692,-0.498417586841131,-0.495477764859172,-0.491388083729115,
-0.482826022098898,-0.470850881481872,-0.433118132058109,-0.393905080040855,
-0.384200422285627,-0.378001527108626,-0.372090363869801,-0.363889938682951,
-0.342536814621959,-0.306012053221888,-0.270412825170174,-0.262603496706861,
-0.258657115929539,-0.255384558852583,-0.251032545615987,-0.240973516492402,
-0.22597559994144,-0.16429582581797,-0.148658257254241,-0.141312948541282,
-0.135518707487021,-0.128936309828955,-0.117358294392849,-0.112633652509009,
-0.0992878568064811,-0.0901262604413663),.UNSPECIFIED.);
#1421=B_SPLINE_CURVE_WITH_KNOTS('',3,(#62098,#62099,#62100,#62101,#62102,
#62103,#62104,#62105,#62106,#62107,#62108,#62109,#62110,#62111,#62112,#62113,
#62114,#62115,#62116,#62117,#62118,#62119,#62120,#62121,#62122,#62123,#62124,
#62125,#62126,#62127,#62128,#62129,#62130,#62131,#62132,#62133,#62134,#62135,
#62136,#62137,#62138,#62139,#62140,#62141,#62142,#62143,#62144,#62145,#62146,
#62147,#62148,#62149,#62150,#62151,#62152,#62153,#62154,#62155,#62156,#62157,
#62158,#62159,#62160,#62161,#62162,#62163,#62164,#62165,#62166,#62167,#62168,
#62169,#62170,#62171,#62172,#62173,#62174,#62175,#62176,#62177,#62178,#62179,
#62180,#62181,#62182,#62183,#62184,#62185,#62186,#62187,#62188,#62189,#62190,
#62191,#62192,#62193,#62194,#62195,#62196,#62197,#62198,#62199,#62200,#62201,
#62202,#62203,#62204,#62205,#62206,#62207,#62208,#62209,#62210,#62211,#62212,
#62213,#62214,#62215,#62216,#62217,#62218,#62219,#62220,#62221,#62222,#62223,
#62224,#62225,#62226,#62227,#62228,#62229,#62230,#62231,#62232,#62233,#62234,
#62235,#62236,#62237,#62238,#62239,#62240,#62241,#62242,#62243,#62244,#62245,
#62246,#62247,#62248,#62249,#62250,#62251,#62252,#62253,#62254,#62255,#62256,
#62257,#62258,#62259,#62260,#62261,#62262,#62263,#62264,#62265,#62266,#62267,
#62268,#62269,#62270,#62271,#62272,#62273,#62274,#62275,#62276,#62277,#62278,
#62279,#62280,#62281,#62282,#62283,#62284,#62285,#62286,#62287,#62288,#62289,
#62290,#62291,#62292,#62293,#62294,#62295,#62296,#62297,#62298,#62299,#62300,
#62301,#62302,#62303,#62304,#62305,#62306,#62307,#62308,#62309,#62310,#62311,
#62312,#62313,#62314,#62315,#62316,#62317,#62318,#62319,#62320,#62321,#62322,
#62323,#62324,#62325,#62326,#62327,#62328,#62329,#62330,#62331,#62332,#62333,
#62334,#62335,#62336,#62337,#62338,#62339,#62340,#62341,#62342,#62343,#62344,
#62345,#62346,#62347,#62348,#62349,#62350,#62351,#62352,#62353,#62354,#62355,
#62356,#62357,#62358,#62359,#62360,#62361,#62362,#62363,#62364,#62365,#62366,
#62367,#62368,#62369),.UNSPECIFIED.,.F.,.F.,(4,2,2,2,2,2,2,2,2,2,2,2,2,
2,2,2,2,2,2,2,2,2,2,2,2,2,2,2,2,2,2,2,2,2,2,2,2,2,2,2,2,2,2,2,2,2,2,2,2,
2,2,2,2,2,2,2,2,2,2,2,2,2,2,2,2,2,2,2,2,2,2,2,2,2,2,2,2,2,2,2,2,2,2,2,2,
2,2,2,2,2,2,2,2,2,2,2,2,2,2,2,2,2,2,2,2,2,2,2,2,2,2,2,2,2,2,2,2,2,2,2,2,
2,2,2,2,2,2,2,2,2,2,2,2,2,2,4),(-2.94522627611978,-2.9278260567548,-2.88209537165937,
-2.86904939939296,-2.86022824290779,-2.86012762899294,-2.86003321938999,
-2.85994447229088,-2.85986090262605,-2.85978207532565,-2.85970759940869,
-2.85963712287195,-2.85957032823019,-2.85950692860159,-2.85944666427833,
-2.85938929973542,-2.85933462101949,-2.85928243343705,-2.85923255950263,
-2.85918483717171,-2.85913911825154,-2.85909526696991,-2.85905315881138,
-2.85901267931485,-2.85897372316421,-2.85893619334639,-2.85890000029291,
-2.85886506119732,-2.85883129945282,-2.85879864407773,-2.8587670291803,
-2.85873639351689,-2.85870668014095,-2.85867783597254,-2.85858012111323,
-2.85848407999915,-2.85838959708076,-2.85829656093362,-2.85820486387315,
-2.85811440161406,-2.85802507290806,-2.85793677919645,-2.85784942430879,
-2.85776291410638,-2.85767715617137,-2.85759205950617,-2.85750753421965,
-2.85742349117799,-2.85733984171817,-2.85725649731425,-2.85383273884977,
-2.85073935320882,-2.84539135417927,-2.82879005941319,-2.78506671315378,
-2.7503379832641,-2.74092770273516,-2.73478915674464,-2.72891117263452,
-2.72055647766217,-2.69967501603011,-2.64635493763055,-2.63106082520032,
-2.62086499746477,-2.61649090726033,-2.61321702191833,-2.60928746787096,
-2.60156184225795,-2.56625414439879,-2.52991195498661,-2.50818290104245,
-2.49993578941481,-2.49401735709842,-2.48783389766611,-2.47820222356469,
-2.44171333151579,-2.40688756654073,-2.39154852184529,-2.38133183481815,
-2.37695436121585,-2.37368021593805,-2.36975312446663,-2.36203988399547,
-2.3260237310847,-2.28940604106807,-2.26841192383277,-2.26025943828437,
-2.25435699980941,-2.24814421656735,-2.23836824285325,-2.19833688616145,
-2.15956242226595,-2.14356056535607,-2.1384171183554,-2.13502554231489,
-2.13145433008986,-2.12545931626638,-2.0992411852945,-2.05369650959472,
-2.02971447160205,-2.02119947198221,-2.015233819974,-2.00983895352222,-2.00256536460833,
-1.98340947856826,-1.91892515319589,-1.90375492269643,-1.89870201804694,
-1.89532764781893,-1.89172731317724,-1.8855974912203,-1.85473878782276,
-1.81289030001618,-1.79728601394542,-1.78508095864178,-1.77837300077994,
-1.77259256650636,-1.76542740239465,-1.7540931702843,-1.6980986404642,-1.66626321796789,
-1.66015138432425,-1.65655478368268,-1.65321763512158,-1.64818631853087,
-1.63428879976942,-1.59294087438025,-1.56624837414105,-1.54846438275313,
-1.54076878823646,-1.53493448118191,-1.52854257305925,-1.51789811129468,
-1.47428171580287,-1.42852668002049,-1.42845108479066),.UNSPECIFIED.);
#1422=B_SPLINE_CURVE_WITH_KNOTS('',3,(#62371,#62372,#62373,#62374,#62375,
#62376,#62377,#62378,#62379,#62380,#62381,#62382,#62383,#62384,#62385,#62386,
#62387,#62388),.UNSPECIFIED.,.F.,.F.,(4,2,2,2,2,2,2,2,4),(-0.0901262604413663,
-0.050740347091941,-0.0273583609058817,-0.0214867594294149,-0.0179417442508245,
-0.0148777648982165,-0.0114578850196497,-0.00665285670582603,-0.000694003661653763),
 .UNSPECIFIED.);
#1423=B_SPLINE_CURVE_WITH_KNOTS('',3,(#62389,#62390,#62391,#62392,#62393,
#62394,#62395,#62396,#62397,#62398,#62399,#62400,#62401,#62402,#62403,#62404,
#62405,#62406,#62407,#62408,#62409,#62410,#62411,#62412,#62413,#62414,#62415,
#62416,#62417,#62418,#62419,#62420,#62421,#62422,#62423,#62424,#62425,#62426,
#62427,#62428,#62429,#62430,#62431,#62432,#62433,#62434,#62435,#62436,#62437,
#62438,#62439,#62440,#62441,#62442,#62443,#62444,#62445,#62446,#62447,#62448,
#62449,#62450,#62451,#62452,#62453,#62454,#62455,#62456,#62457,#62458,#62459,
#62460,#62461,#62462,#62463,#62464,#62465,#62466,#62467,#62468,#62469,#62470,
#62471,#62472,#62473,#62474,#62475,#62476,#62477,#62478,#62479,#62480,#62481,
#62482,#62483,#62484,#62485,#62486,#62487,#62488,#62489,#62490,#62491,#62492,
#62493,#62494,#62495,#62496,#62497,#62498,#62499,#62500,#62501,#62502,#62503,
#62504,#62505,#62506,#62507,#62508,#62509,#62510,#62511,#62512,#62513,#62514,
#62515,#62516,#62517,#62518,#62519,#62520,#62521,#62522,#62523,#62524,#62525,
#62526,#62527,#62528,#62529,#62530,#62531,#62532,#62533,#62534,#62535,#62536,
#62537,#62538,#62539,#62540,#62541,#62542,#62543,#62544,#62545,#62546,#62547,
#62548,#62549,#62550,#62551,#62552,#62553,#62554,#62555,#62556,#62557,#62558,
#62559,#62560,#62561,#62562,#62563,#62564,#62565,#62566,#62567,#62568,#62569,
#62570,#62571,#62572,#62573,#62574,#62575,#62576),.UNSPECIFIED.,.F.,.F.,
(4,2,2,2,2,2,2,2,2,2,2,2,2,2,2,2,2,2,2,2,2,2,2,2,2,2,2,2,2,2,2,2,2,2,2,
2,2,2,2,2,2,2,2,2,2,2,2,2,2,2,2,2,2,2,2,2,2,2,2,2,2,2,2,2,2,2,2,2,2,2,2,
2,2,2,2,2,2,2,2,2,2,2,2,2,2,2,2,2,2,2,2,2,2,4),(-3.03589799970467,-2.96791287576106,
-2.94642853128536,-2.93821240019877,-2.9322992873552,-2.92610657953658,
-2.91642922553783,-2.87792590980494,-2.83954868038511,-2.82747534841312,
-2.82138142172164,-2.81663901184802,-2.81658441314679,-2.81652992760057,
-2.81647543426394,-2.81642080975002,-2.81636592706931,-2.81631065435479,
-2.81625485339372,-2.81619837807209,-2.81614107252712,-2.81285634926421,
-2.80972862790769,-2.80420060556432,-2.78567240527661,-2.73906801988853,
-2.70883636433632,-2.69973082199681,-2.69365288502093,-2.68773168954697,
-2.67913387965057,-2.65635436189848,-2.59742774031163,-2.58168715932836,
-2.57657140156469,-2.57318509837418,-2.56960525170644,-2.56357058263477,
-2.53641413385352,-2.49162411804925,-2.46782118015233,-2.45932583692511,
-2.45336353629828,-2.44796493891926,-2.43927785077053,-2.41560691348531,
-2.3579385945619,-2.3420625666281,-2.33693207651549,-2.33354278861617,-2.33041318804702,
-2.32487656379686,-2.30625418978656,-2.25973167709141,-2.22951546843293,
-2.22041043080765,-2.21433214480538,-2.20841010130841,-2.19981013459804,
-2.17701671024055,-2.11810053533784,-2.10235656187319,-2.0972400808126,
-2.09385338721421,-2.09027322517966,-2.08423819901111,-2.057085677852,-2.01228541589481,
-1.98847862929008,-1.97998224450321,-1.97401929301848,-1.96862015868814,
-1.96133062537079,-1.94203652545307,-1.87774036954437,-1.86252795889626,
-1.85746971663518,-1.85409396628481,-1.850494706891,-1.84437158094169,-1.81423392915018,
-1.771808614623,-1.74860644240584,-1.74017899290998,-1.73422803031838,-1.72881577049308,
-1.72005282703135,-1.6955874318218,-1.64400095612153,-1.62381968244339,
-1.61829389179362,-1.61482292791769,-1.61176524667919,-1.60794378585001),
 .UNSPECIFIED.);
#1424=B_SPLINE_CURVE_WITH_KNOTS('',3,(#62582,#62583,#62584,#62585,#62586,
#62587,#62588,#62589,#62590,#62591,#62592,#62593,#62594,#62595,#62596,#62597,
#62598,#62599,#62600,#62601,#62602,#62603,#62604,#62605,#62606,#62607,#62608,
#62609,#62610,#62611,#62612,#62613,#62614,#62615,#62616,#62617,#62618,#62619,
#62620,#62621,#62622,#62623,#62624,#62625,#62626,#62627,#62628,#62629,#62630,
#62631,#62632,#62633,#62634,#62635,#62636,#62637,#62638,#62639,#62640,#62641,
#62642,#62643,#62644,#62645,#62646,#62647,#62648,#62649,#62650,#62651,#62652,
#62653,#62654,#62655,#62656,#62657,#62658,#62659,#62660,#62661,#62662,#62663,
#62664,#62665,#62666,#62667,#62668,#62669,#62670,#62671,#62672,#62673,#62674,
#62675,#62676,#62677,#62678,#62679,#62680,#62681,#62682,#62683,#62684,#62685,
#62686,#62687,#62688,#62689,#62690,#62691,#62692,#62693,#62694,#62695,#62696,
#62697,#62698,#62699,#62700,#62701,#62702,#62703,#62704,#62705,#62706,#62707,
#62708,#62709,#62710,#62711,#62712,#62713,#62714,#62715,#62716,#62717,#62718,
#62719,#62720,#62721,#62722,#62723,#62724,#62725,#62726,#62727,#62728,#62729,
#62730,#62731,#62732,#62733,#62734,#62735,#62736,#62737,#62738,#62739,#62740,
#62741,#62742,#62743,#62744,#62745,#62746,#62747,#62748,#62749,#62750,#62751,
#62752,#62753,#62754,#62755,#62756,#62757,#62758,#62759,#62760,#62761,#62762,
#62763,#62764,#62765,#62766,#62767,#62768,#62769,#62770,#62771,#62772,#62773,
#62774,#62775),.UNSPECIFIED.,.F.,.F.,(4,2,2,2,2,2,2,2,2,2,2,2,2,2,2,2,2,
2,2,2,2,2,2,2,2,2,2,2,2,2,2,2,2,2,2,2,2,2,2,2,2,2,2,2,2,2,2,2,2,2,2,2,2,
2,2,2,2,2,2,2,2,2,2,2,2,2,2,2,2,2,2,2,2,2,2,2,2,2,2,2,2,2,2,2,2,2,2,2,2,
2,2,2,2,2,2,2,4),(-1.42841089888011,-1.39743125910206,-1.38627017924954,
-1.37971024003408,-1.37449024409628,-1.36739713881939,-1.35318936919051,
-1.33397199569542,-1.30425467612233,-1.26821184225344,-1.26198698498176,
-1.25836536333979,-1.25500035935803,-1.25000339313463,-1.23533164811459,
-1.16510950920946,-1.14922548606105,-1.14183670814692,-1.1360367879022,
-1.12947804076786,-1.11802308202274,-1.08031352273074,-1.03711764803795,
-1.02539796242703,-1.02067181999798,-1.0173532107127,-1.01362279311818,
-1.00688280537667,-0.964307626410539,-0.918424412513452,-0.907028676291929,
-0.900418977923977,-0.895205902154449,-0.888182772956108,-0.874350769863942,
-0.831502867027447,-0.791039008700119,-0.78358331499852,-0.77966032431973,
-0.77638392736607,-0.771996082351945,-0.761723097388814,-0.746267710548788,
-0.691148415155324,-0.671753967625412,-0.664450734642208,-0.659047360334772,
-0.653085412857472,-0.644601701715289,-0.620923025878264,-0.576659721088888,
-0.548788350275378,-0.542723754773779,-0.539136586917193,-0.535752407258442,
-0.530652911746744,-0.515072306329791,-0.454838251416227,-0.432962182639879,
-0.424470552686589,-0.41856654163639,-0.412459729485191,-0.403217872933108,
-0.371192462615528,-0.343752583386746,-0.311981018327415,-0.304242367226241,
-0.30030924760718,-0.297034193176301,-0.292660996599385,-0.282477285733853,
-0.267213970295811,-0.211933234788478,-0.1924315678338,-0.18511089400292,
-0.179703543397623,-0.173745873371159,-0.173512973598671,-0.173333278919473,
-0.173190533760916,-0.173074616792294,-0.172510806331846,-0.171945837720901,
-0.171370056799897,-0.170773913773818,-0.170147435910445,-0.158407839669011,
-0.143238213392588,-0.103825627830268,-0.0722918285290809,-0.0645660267556695,
-0.0606354498802551,-0.0573601138789549,-0.054120789610304,-0.0497727212624637,
-0.0394267764559731,-0.000694732967017225),.UNSPECIFIED.);
#1425=B_SPLINE_CURVE_WITH_KNOTS('',3,(#62776,#62777,#62778,#62779,#62780,
#62781,#62782,#62783,#62784,#62785,#62786,#62787,#62788,#62789,#62790,#62791),
 .UNSPECIFIED.,.F.,.F.,(4,2,2,2,2,2,2,4),(-3.03489967675623,-2.99347372483665,
-2.98529204977498,-2.97935572956225,-2.97339855375462,-2.96727673357796,
-2.95794991026736,-2.94522627611978),.UNSPECIFIED.);
#1426=B_SPLINE_CURVE_WITH_KNOTS('',3,(#62792,#62793,#62794,#62795,#62796,
#62797,#62798,#62799,#62800,#62801,#62802,#62803,#62804,#62805,#62806,#62807,
#62808,#62809,#62810,#62811,#62812,#62813,#62814,#62815,#62816,#62817,#62818,
#62819,#62820,#62821,#62822,#62823,#62824,#62825,#62826,#62827,#62828,#62829,
#62830,#62831,#62832,#62833,#62834,#62835,#62836,#62837,#62838,#62839,#62840,
#62841,#62842,#62843,#62844,#62845,#62846,#62847,#62848,#62849,#62850,#62851,
#62852,#62853,#62854,#62855,#62856,#62857,#62858,#62859,#62860,#62861,#62862,
#62863,#62864,#62865,#62866,#62867,#62868,#62869,#62870,#62871,#62872,#62873,
#62874,#62875,#62876,#62877,#62878,#62879,#62880,#62881,#62882,#62883,#62884,
#62885,#62886,#62887,#62888,#62889,#62890,#62891,#62892,#62893,#62894,#62895,
#62896,#62897,#62898,#62899,#62900,#62901,#62902,#62903,#62904,#62905,#62906,
#62907,#62908,#62909,#62910,#62911,#62912,#62913,#62914,#62915,#62916,#62917,
#62918,#62919,#62920,#62921,#62922,#62923,#62924,#62925,#62926,#62927,#62928,
#62929,#62930,#62931,#62932,#62933,#62934,#62935,#62936,#62937,#62938,#62939,
#62940,#62941,#62942,#62943,#62944,#62945,#62946,#62947,#62948,#62949,#62950,
#62951,#62952,#62953,#62954,#62955,#62956,#62957,#62958,#62959,#62960,#62961,
#62962,#62963,#62964,#62965,#62966,#62967,#62968,#62969,#62970,#62971,#62972,
#62973,#62974,#62975,#62976,#62977,#62978,#62979,#62980,#62981,#62982,#62983,
#62984,#62985,#62986,#62987,#62988,#62989,#62990,#62991,#62992,#62993,#62994,
#62995,#62996,#62997,#62998,#62999,#63000,#63001,#63002,#63003,#63004,#63005,
#63006,#63007,#63008,#63009,#63010,#63011,#63012,#63013,#63014,#63015,#63016,
#63017,#63018,#63019,#63020,#63021,#63022,#63023,#63024,#63025,#63026,#63027,
#63028,#63029,#63030,#63031,#63032,#63033,#63034,#63035,#63036,#63037,#63038,
#63039,#63040,#63041,#63042,#63043,#63044,#63045,#63046,#63047,#63048,#63049,
#63050,#63051,#63052,#63053,#63054,#63055,#63056,#63057,#63058,#63059,#63060,
#63061,#63062,#63063,#63064,#63065,#63066,#63067,#63068,#63069,#63070,#63071),
 .UNSPECIFIED.,.F.,.F.,(4,2,2,2,2,2,2,2,2,2,2,2,2,2,2,2,2,2,2,2,2,2,2,2,
2,2,2,2,2,2,2,2,2,2,2,2,2,2,2,2,2,2,2,2,2,2,2,2,2,2,2,2,2,2,2,2,2,2,2,2,
2,2,2,2,2,2,2,2,2,2,2,2,2,2,2,2,2,2,2,2,2,2,2,2,2,2,2,2,2,2,2,2,2,2,2,2,
2,2,2,2,2,2,2,2,2,2,2,2,2,2,2,2,2,2,2,2,2,2,2,2,2,2,2,2,2,2,2,2,2,2,2,2,
2,2,2,2,2,2,2,4),(-1.60794378585001,-1.6066158861157,-1.59177736166794,
-1.55115553904906,-1.51854628348446,-1.50515840438898,-1.49813701178107,
-1.49236179629711,-1.48553263022734,-1.47271585801169,-1.43471963056368,
-1.38671505427769,-1.37986218412915,-1.37606821381087,-1.37276843159126,
-1.36817105785611,-1.35654148085098,-1.33800316922406,-1.27611797947543,
-1.26431251812801,-1.25761632678228,-1.25183359864333,-1.24464955941393,
-1.22993588235711,-1.21895620905585,-1.17872466213274,-1.14822555055159,
-1.14063653824262,-1.13668599883945,-1.13341335235904,-1.12906561020843,
-1.11903472094206,-1.10409753113472,-1.0349630755503,-1.0238058074265,-1.01730858573358,
-1.0114992411048,-1.00400944532224,-0.987516967753724,-0.963702091217662,
-0.916548228951036,-0.903395688130634,-0.898462383622608,-0.895142748715777,
-0.891511492739865,-0.885238612798559,-0.845741050902313,-0.795650688148293,
-0.784415561519985,-0.777841032989775,-0.772624942467169,-0.76555760157846,
-0.751482548225762,-0.732513896729955,-0.702416609605827,-0.666308545371244,
-0.66008156541868,-0.656460189012472,-0.653096750673222,-0.648104178589684,
-0.633461975544626,-0.562683402235284,-0.547150149963822,-0.539822810700446,
-0.534030182942953,-0.527436227594513,-0.515801029922933,-0.476642174124733,
-0.430305207357967,-0.421823393302142,-0.417748593392565,-0.41448461020491,
-0.410290227558175,-0.401150876899449,-0.388047103570359,-0.341808185496286,
-0.312128198316772,-0.302890352388055,-0.296785467201068,-0.290813964774743,
-0.2822711366414,-0.258053633019459,-0.211540007429808,-0.186386526791709,
-0.180434128460067,-0.176871650713859,-0.173473262210404,-0.173390655692988,
-0.173307892005637,-0.173224882450212,-0.173141538753151,-0.173057772752981,
-0.172973496037839,-0.172888619640973,-0.172803053745737,-0.172716707327175,
-0.172629487850089,-0.172541300975064,-0.172452050235491,-0.172361636691484,
-0.172269958605175,-0.172176911106818,-0.172082385857964,-0.17198627066799,
-0.171888449104264,-0.171788800128309,-0.171757287849786,-0.171724692046217,
-0.171690944169791,-0.171655970274543,-0.171619690469221,-0.171582018348421,
-0.17154286030542,-0.171502114816463,-0.171459671566905,-0.171415410575822,
-0.171369201107853,-0.171320900520313,-0.171270352934051,-0.171217387689528,
-0.171161817655816,-0.171103437331629,-0.171042020665314,-0.170977318504732,
-0.170909055815295,-0.170836928430975,-0.170760599338807,-0.170679694477294,
-0.170593797887025,-0.170502446143018,-0.170405121993403,-0.170301247048615,
-0.1701901733403,-0.17007117363754,-0.169943430328354,-0.169806022636715,
-0.158945166949799,-0.152234720465392,-0.120589434598602,-0.0904170319211295),
 .UNSPECIFIED.);
#1427=B_SPLINE_CURVE_WITH_KNOTS('',3,(#63076,#63077,#63078,#63079,#63080,
#63081,#63082,#63083,#63084,#63085,#63086,#63087,#63088,#63089,#63090,#63091,
#63092,#63093,#63094,#63095,#63096,#63097,#63098,#63099,#63100,#63101,#63102,
#63103,#63104,#63105,#63106,#63107,#63108,#63109,#63110,#63111,#63112,#63113,
#63114,#63115,#63116,#63117,#63118,#63119,#63120,#63121,#63122,#63123,#63124,
#63125,#63126,#63127,#63128,#63129,#63130,#63131,#63132,#63133,#63134,#63135,
#63136,#63137,#63138,#63139,#63140,#63141,#63142,#63143,#63144,#63145,#63146,
#63147,#63148,#63149,#63150,#63151,#63152,#63153,#63154,#63155,#63156,#63157,
#63158,#63159,#63160,#63161,#63162,#63163,#63164,#63165,#63166,#63167,#63168,
#63169,#63170,#63171,#63172,#63173,#63174,#63175,#63176,#63177,#63178,#63179,
#63180,#63181,#63182,#63183,#63184,#63185,#63186,#63187,#63188,#63189,#63190,
#63191,#63192,#63193,#63194,#63195,#63196,#63197,#63198,#63199,#63200,#63201,
#63202,#63203,#63204,#63205,#63206,#63207,#63208,#63209,#63210,#63211,#63212,
#63213,#63214,#63215,#63216,#63217,#63218,#63219,#63220,#63221,#63222,#63223,
#63224,#63225,#63226,#63227,#63228,#63229,#63230,#63231,#63232,#63233,#63234,
#63235,#63236,#63237,#63238,#63239,#63240,#63241,#63242,#63243,#63244,#63245,
#63246,#63247,#63248,#63249,#63250,#63251,#63252,#63253,#63254,#63255,#63256,
#63257,#63258,#63259,#63260,#63261,#63262,#63263,#63264,#63265,#63266,#63267,
#63268,#63269,#63270,#63271,#63272,#63273),.UNSPECIFIED.,.F.,.F.,(4,2,2,
2,2,2,2,2,2,2,2,2,2,2,2,2,2,2,2,2,2,2,2,2,2,2,2,2,2,2,2,2,2,2,2,2,2,2,2,
2,2,2,2,2,2,2,2,2,2,2,2,2,2,2,2,2,2,2,2,2,2,2,2,2,2,2,2,2,2,2,2,2,2,2,2,
2,2,2,2,2,2,2,2,2,2,2,2,2,2,2,2,2,2,2,2,2,2,2,4),(-2.94574554020504,-2.94263391637022,
-2.9380216451502,-2.93471991858296,-2.93093378306239,-2.92411683916993,
-2.87587854893091,-2.83876665948301,-2.82939216056483,-2.82300227906537,
-2.82247231816296,-2.8219405544679,-2.82137344699033,-2.82071838771216,
-2.81521747057133,-2.80905172400534,-2.79951378668693,-2.76579916297151,
-2.72335017003197,-2.70471569839339,-2.69931749059466,-2.69587344932726,
-2.6923695082861,-2.68669074246475,-2.66655554382784,-2.62147346205144,
-2.59156339601923,-2.58248133282319,-2.57640655770994,-2.57047909404194,
-2.56323577358459,-2.54448605555577,-2.48848806087467,-2.47303865797311,
-2.46276964812287,-2.45838264349705,-2.45510660362791,-2.45118362243595,
-2.44349572581563,-2.40611489576622,-2.36891202207806,-2.35550335480519,
-2.34460979159622,-2.33816598007048,-2.33234391117117,-2.3248785233301,
-2.30804491450854,-2.24810253692434,-2.23308072341452,-2.22301090488542,
-2.21865640254579,-2.21538289749203,-2.21143628845636,-2.20386745340013,
-2.16738806668926,-2.1306054782168,-2.10998194231242,-2.1018762054719,-2.09597947889058,
-2.08974746991473,-2.07988635061938,-2.03879731401897,-2.00172771303634,
-1.98529435238335,-1.98010439757153,-1.97670262553101,-1.97314300588603,
-1.96720654572637,-1.94248942485543,-1.89566384939458,-1.871377981766,-1.86282671637233,
-1.8568525433889,-1.8514609315774,-1.84420838736942,-1.8253348945646,-1.76041744827706,
-1.74527800153628,-1.74022711806984,-1.73685207904848,-1.73324878561934,
-1.72710978478299,-1.69487596940296,-1.65402552840008,-1.63859364088875,
-1.62648759868956,-1.61979748071452,-1.61401281901431,-1.60681697911757,
-1.59538032841674,-1.53949392164539,-1.51782831778016,-1.50518352924775,
-1.50031119422111,-1.49700132260882,-1.49334506109092,-1.48695803363345,
-1.44853616035284,-1.42841089888011),.UNSPECIFIED.);
#1428=B_SPLINE_CURVE_WITH_KNOTS('',3,(#63275,#63276,#63277,#63278,#63279,
#63280,#63281,#63282,#63283,#63284,#63285,#63286,#63287,#63288,#63289,#63290,
#63291,#63292),.UNSPECIFIED.,.F.,.F.,(4,2,2,2,2,2,2,2,4),(-0.0904170319211295,
-0.077397385079546,-0.0657139835705077,-0.0590439735663556,-0.0532594854266007,
-0.0476886497618599,-0.0406051108281494,-0.0267866391532106,-0.000694393962764245),
 .UNSPECIFIED.);
#1429=B_SPLINE_CURVE_WITH_KNOTS('',3,(#63293,#63294,#63295,#63296,#63297,
#63298,#63299,#63300,#63301,#63302),.UNSPECIFIED.,.F.,.F.,(4,1,1,1,1,1,
1,4),(65.9734485846553,66.2383482818393,67.2308234190585,68.2232985562776,
69.2157736934968,70.208248830716,71.2007239679351,71.8851149398144),
 .UNSPECIFIED.);
#1430=B_SPLINE_CURVE_WITH_KNOTS('',3,(#63308,#63309,#63310,#63311,#63312,
#63313,#63314,#63315,#63316,#63317),.UNSPECIFIED.,.F.,.F.,(4,1,1,1,1,1,
1,4),(72.2566310325652,72.8364994652893,73.8289746025085,74.8214497397277,
75.8139248769468,76.806400014166,77.7988751513852,78.1697058192857),
 .UNSPECIFIED.);
#1431=B_SPLINE_CURVE_WITH_KNOTS('',3,(#63318,#63319,#63320,#63321,#63322,
#63323,#63324,#63325),.UNSPECIFIED.,.F.,.F.,(4,2,2,4),(-3.035220816981,
-2.97315166642837,-2.95436542165648,-2.94574554020504),.UNSPECIFIED.);
#1432=B_SPLINE_CURVE_WITH_KNOTS('',3,(#63327,#63328,#63329,#63330,#63331),
 .UNSPECIFIED.,.F.,.F.,(4,1,4),(71.8851149398144,72.1931991051543,72.2566310325652),
 .UNSPECIFIED.);
#1433=B_SPLINE_CURVE_WITH_KNOTS('',3,(#63332,#63333,#63334,#63335,#63336,
#63337,#63338,#63339,#63340,#63341,#63342,#63343,#63344,#63345,#63346,#63347,
#63348,#63349,#63350,#63351,#63352,#63353,#63354,#63355,#63356,#63357,#63358,
#63359,#63360,#63361,#63362,#63363,#63364,#63365,#63366,#63367,#63368,#63369,
#63370,#63371,#63372,#63373,#63374,#63375,#63376,#63377,#63378,#63379,#63380,
#63381,#63382,#63383,#63384,#63385,#63386,#63387,#63388,#63389,#63390,#63391,
#63392,#63393,#63394,#63395,#63396,#63397,#63398,#63399,#63400,#63401,#63402,
#63403,#63404,#63405,#63406,#63407,#63408,#63409,#63410,#63411,#63412,#63413,
#63414,#63415,#63416,#63417,#63418,#63419,#63420,#63421,#63422,#63423,#63424,
#63425,#63426,#63427,#63428,#63429,#63430,#63431,#63432,#63433,#63434,#63435,
#63436,#63437,#63438,#63439,#63440,#63441,#63442,#63443,#63444,#63445,#63446,
#63447,#63448,#63449,#63450,#63451,#63452,#63453,#63454,#63455,#63456,#63457,
#63458,#63459,#63460,#63461,#63462,#63463,#63464,#63465,#63466,#63467,#63468,
#63469,#63470,#63471,#63472,#63473,#63474,#63475,#63476,#63477,#63478,#63479,
#63480,#63481,#63482,#63483,#63484,#63485,#63486,#63487,#63488,#63489,#63490,
#63491,#63492,#63493,#63494,#63495,#63496,#63497,#63498,#63499,#63500,#63501,
#63502,#63503,#63504,#63505,#63506,#63507,#63508,#63509,#63510,#63511,#63512,
#63513,#63514,#63515,#63516,#63517,#63518,#63519,#63520,#63521,#63522,#63523,
#63524,#63525,#63526,#63527,#63528,#63529,#63530,#63531,#63532,#63533,#63534,
#63535,#63536,#63537,#63538,#63539),.UNSPECIFIED.,.F.,.F.,(4,2,2,2,2,2,
2,2,2,2,2,2,2,2,2,2,2,2,2,2,2,2,2,2,2,2,2,2,2,2,2,2,2,2,2,2,2,2,2,2,2,2,
2,2,2,2,2,2,2,2,2,2,2,2,2,2,2,2,2,2,2,2,2,2,2,2,2,2,2,2,2,2,2,2,2,2,2,2,
2,2,2,2,2,2,2,2,2,2,2,2,2,2,2,2,2,2,2,2,2,2,2,2,2,4),(-7.40692637570555,
-7.33746437258257,-7.31576929720708,-7.30752912445337,-7.30161418438117,
-7.29543312973761,-7.28580270729364,-7.24920865613869,-7.2092814225013,
-7.19698698858259,-7.19082090059144,-7.18601372586172,-7.18595005520301,
-7.18588678551918,-7.18582375706269,-7.18576080878017,-7.18569777663025,
-7.18563449182612,-7.18557077886074,-7.18550645330422,-7.18544131927868,
-7.18537516657691,-7.1853077672651,-7.18523887163769,-7.18516820337284,
-7.18509545360177,-7.18502027361203,-7.18494226570937,-7.18486097167816,
-7.18477585804234,-7.18468629686798,-7.18459154048083,-7.1813183202842,
-7.17739909707478,-7.1697198043893,-7.1336669077005,-7.09707122502135,-7.07606809000857,
-7.06791695842809,-7.06201701247935,-7.05580825745978,-7.04604178956603,
-7.00467080220601,-6.9678474721791,-6.95135440212621,-6.94616150449742,
-6.94276135379914,-6.93920741626362,-6.93328752935679,-6.90892501571539,
-6.86184884812638,-6.83751650816176,-6.82896540451994,-6.82299537267477,
-6.81761015113748,-6.81037028795483,-6.79160161740801,-6.72662567342674,
-6.71148979386952,-6.70644234475273,-6.70307020960615,-6.69947081496129,
-6.69334010803431,-6.66185240968146,-6.62048937879845,-6.59758206117575,
-6.5891930023695,-6.58325176049818,-6.57711236280072,-6.56768977963242,
-6.53610458464198,-6.49175978595594,-6.47277125115529,-6.46734515395923,
-6.4638969215758,-6.46082644294791,-6.45559802315712,-6.44006871812096,
-6.4000178007572,-6.37381748163223,-6.35624973341649,-6.34859045612672,
-6.34276368012452,-6.33636042015771,-6.32564917113136,-6.26942833940005,
-6.23467507315847,-6.22849792247837,-6.22488840217855,-6.22156072941251,
-6.21738466586562,-6.20645904983877,-6.12907604803193,-6.11490518625184,
-6.10782319040023,-6.10260860717325,-6.09605201193141,-6.084888117701,-6.0338921044371,
-5.9950992869525,-5.98886992452876,-5.98524941537587,-5.98192771141387,
-5.97968578406166),.UNSPECIFIED.);
#1434=B_SPLINE_CURVE_WITH_KNOTS('',3,(#63545,#63546,#63547,#63548,#63549,
#63550,#63551,#63552,#63553,#63554,#63555,#63556,#63557,#63558,#63559,#63560,
#63561,#63562,#63563,#63564,#63565,#63566,#63567,#63568,#63569,#63570,#63571,
#63572,#63573,#63574,#63575,#63576,#63577,#63578,#63579,#63580,#63581,#63582,
#63583,#63584,#63585,#63586,#63587,#63588,#63589,#63590,#63591,#63592,#63593,
#63594,#63595,#63596,#63597,#63598,#63599,#63600,#63601,#63602,#63603,#63604,
#63605,#63606,#63607,#63608,#63609,#63610,#63611,#63612,#63613,#63614,#63615,
#63616,#63617,#63618,#63619,#63620,#63621,#63622,#63623,#63624,#63625,#63626,
#63627,#63628,#63629,#63630,#63631,#63632,#63633,#63634,#63635,#63636,#63637,
#63638,#63639,#63640,#63641,#63642,#63643,#63644,#63645,#63646,#63647,#63648,
#63649,#63650,#63651,#63652,#63653,#63654,#63655,#63656,#63657,#63658,#63659,
#63660,#63661,#63662,#63663,#63664,#63665,#63666,#63667,#63668,#63669,#63670,
#63671,#63672,#63673,#63674,#63675,#63676,#63677,#63678,#63679,#63680,#63681,
#63682,#63683,#63684,#63685,#63686,#63687,#63688,#63689,#63690,#63691,#63692,
#63693,#63694,#63695,#63696,#63697,#63698,#63699,#63700,#63701,#63702,#63703,
#63704,#63705,#63706,#63707,#63708,#63709,#63710,#63711,#63712,#63713,#63714,
#63715,#63716,#63717,#63718,#63719,#63720,#63721,#63722),.UNSPECIFIED.,
 .F.,.F.,(4,3,3,3,3,3,3,3,3,3,3,3,3,3,3,3,3,3,3,3,3,3,3,3,3,3,3,3,3,3,3,
3,3,3,3,3,3,3,3,3,3,3,3,3,3,3,3,3,3,3,3,3,3,3,3,3,3,3,3,4),(78.5398163397448,
78.6684221201328,78.7913502886043,78.8915768985185,78.9916607299099,79.0916299674899,
79.1915365989967,79.2914114348292,79.3912852456916,79.4912573874797,79.5912772725973,
79.691475689468,79.7838254258235,79.8840520360163,79.9841358676786,80.0841051055166,
80.1840117372737,80.2838865733481,80.3837603844441,80.4837325264511,80.5837524117798,
80.6839508288464,80.7763005630427,80.8765271760024,80.9766110104464,81.0765802510749,
81.1764868856266,81.2763617244957,81.3762355383828,81.4762076831553,81.5762275712401,
81.6764259910143,81.7687757002619,81.8690023062344,81.9690861336894,82.069055367359,
82.1689619949731,82.2688368269357,82.3687106339565,82.4686827719735,82.5687026533527,
82.6689010665837,82.761250837481,82.861477447805,82.9615612795589,83.0615305174294,
83.1614371491829,83.2613119852182,83.3611857962398,83.4611579381179,83.5611778232878,
83.6613762401475,83.7537259747002,83.8539302864532,83.9540022423295,84.0539728511632,
84.1538861754786,84.2537613122279,84.353676596689,84.4517779076862),
 .UNSPECIFIED.);
#1435=B_SPLINE_CURVE_WITH_KNOTS('',3,(#63723,#63724,#63725,#63726),
 .UNSPECIFIED.,.F.,.F.,(4,4),(78.1697058192857,78.5398163397448),
 .UNSPECIFIED.);
#1436=B_SPLINE_CURVE_WITH_KNOTS('',3,(#63727,#63728,#63729,#63730,#63731,
#63732,#63733,#63734,#63735,#63736,#63737,#63738,#63739,#63740,#63741,#63742,
#63743,#63744,#63745,#63746,#63747,#63748,#63749,#63750,#63751,#63752,#63753,
#63754,#63755,#63756,#63757,#63758,#63759,#63760,#63761,#63762,#63763,#63764,
#63765,#63766,#63767,#63768,#63769,#63770,#63771,#63772,#63773,#63774,#63775,
#63776,#63777,#63778,#63779,#63780,#63781,#63782,#63783,#63784,#63785,#63786,
#63787,#63788,#63789,#63790,#63791,#63792,#63793,#63794,#63795,#63796,#63797,
#63798,#63799,#63800,#63801,#63802,#63803,#63804,#63805,#63806,#63807,#63808,
#63809,#63810,#63811,#63812,#63813,#63814,#63815,#63816,#63817,#63818,#63819,
#63820,#63821,#63822,#63823,#63824,#63825,#63826,#63827,#63828,#63829,#63830,
#63831,#63832,#63833,#63834,#63835,#63836,#63837,#63838,#63839,#63840,#63841,
#63842,#63843,#63844,#63845,#63846,#63847,#63848,#63849,#63850,#63851,#63852,
#63853,#63854,#63855,#63856,#63857,#63858,#63859,#63860,#63861,#63862,#63863,
#63864,#63865,#63866,#63867,#63868,#63869,#63870,#63871,#63872,#63873,#63874,
#63875,#63876,#63877,#63878,#63879,#63880,#63881,#63882,#63883,#63884,#63885,
#63886,#63887,#63888,#63889,#63890,#63891,#63892,#63893,#63894,#63895,#63896,
#63897,#63898,#63899,#63900,#63901,#63902,#63903,#63904,#63905,#63906,#63907,
#63908,#63909,#63910),.UNSPECIFIED.,.F.,.F.,(4,2,2,2,2,2,2,2,2,2,2,2,2,
2,2,2,2,2,2,2,2,2,2,2,2,2,2,2,2,2,2,2,2,2,2,2,2,2,2,2,2,2,2,2,2,2,2,2,2,
2,2,2,2,2,2,2,2,2,2,2,2,2,2,2,2,2,2,2,2,2,2,2,2,2,2,2,2,2,2,2,2,2,2,2,2,
2,2,2,2,2,2,4),(-5.97968578406166,-5.97777524899889,-5.96707634600142,-5.91748140018603,
-5.89328770447047,-5.87662121589563,-5.86910587326657,-5.86329664062136,
-5.85681985478997,-5.84575034987089,-5.78380545876526,-5.75510400534421,
-5.74909749852156,-5.7455244880415,-5.74217609187747,-5.73707910099528,
-5.72265289987859,-5.67684586465858,-5.64155872287236,-5.63211814690166,
-5.62597455986409,-5.62010221364698,-5.61307526092356,-5.59563511192601,
-5.53704783298034,-5.52202247801489,-5.51195266290995,-5.50759987078933,
-5.50432841498464,-5.5003853507009,-5.49282624576918,-5.45623640489311,
-5.41943012074704,-5.39892935702118,-5.39084341047394,-5.38495287984466,
-5.37872008773172,-5.36884182474448,-5.32789109469462,-5.29074715594446,
-5.27432912047089,-5.26914291396222,-5.26574342111177,-5.26218611071873,
-5.25625354543958,-5.23156433738646,-5.18474060543174,-5.16046146113616,
-5.15191453724468,-5.14594401978716,-5.14055615412961,-5.13330938979103,
-5.11446582208134,-5.04956544469465,-5.0344166596197,-5.02936680749083,
-5.0259935326858,-5.02239343949439,-5.01626249761823,-4.98509416183607,
-4.94347411652509,-4.92049309607189,-4.91209370836017,-4.90614937295933,
-4.90001037365684,-4.89059574826412,-4.85915774427427,-4.81465357471461,
-4.80175423360786,-4.79271937558736,-4.78854430074904,-4.78559952472588,
-4.7816698806427,-4.77394237969323,-4.73872282011194,-4.70242150679562,
-4.68058501867143,-4.67232490112911,-4.66640480152499,-4.66022635419281,
-4.65061685025712,-4.6149944689493,-4.57918774502019,-4.56388220746901,
-4.55368117402625,-4.54930655534362,-4.5460330239758,-4.54210494808226,
-4.53438530686615,-4.50290763004632,-4.47625482696426,-4.46296054289888),
 .UNSPECIFIED.);
#1437=B_SPLINE_CURVE_WITH_KNOTS('',3,(#63916,#63917,#63918,#63919,#63920,
#63921,#63922,#63923,#63924,#63925,#63926,#63927,#63928,#63929,#63930,#63931,
#63932,#63933,#63934,#63935,#63936,#63937,#63938,#63939,#63940,#63941,#63942,
#63943,#63944,#63945,#63946,#63947,#63948,#63949,#63950,#63951,#63952,#63953,
#63954,#63955,#63956,#63957,#63958,#63959,#63960,#63961,#63962,#63963,#63964,
#63965,#63966,#63967,#63968,#63969,#63970,#63971,#63972,#63973,#63974,#63975,
#63976,#63977,#63978,#63979,#63980,#63981,#63982,#63983,#63984,#63985,#63986,
#63987,#63988,#63989,#63990,#63991,#63992,#63993,#63994,#63995,#63996,#63997,
#63998,#63999,#64000,#64001,#64002,#64003,#64004,#64005,#64006,#64007,#64008,
#64009,#64010,#64011,#64012,#64013,#64014,#64015,#64016,#64017,#64018,#64019,
#64020,#64021,#64022,#64023,#64024,#64025,#64026,#64027,#64028,#64029,#64030,
#64031,#64032,#64033,#64034,#64035,#64036,#64037,#64038,#64039,#64040,#64041,
#64042,#64043,#64044,#64045,#64046,#64047,#64048,#64049,#64050,#64051,#64052,
#64053,#64054,#64055,#64056,#64057,#64058,#64059,#64060,#64061,#64062,#64063,
#64064,#64065,#64066,#64067,#64068,#64069,#64070,#64071,#64072,#64073,#64074,
#64075,#64076,#64077,#64078,#64079,#64080,#64081,#64082,#64083,#64084,#64085,
#64086,#64087,#64088,#64089,#64090,#64091,#64092,#64093,#64094,#64095,#64096,
#64097,#64098,#64099,#64100,#64101,#64102,#64103,#64104,#64105,#64106,#64107,
#64108,#64109,#64110,#64111,#64112,#64113,#64114,#64115,#64116,#64117,#64118,
#64119,#64120,#64121,#64122,#64123,#64124,#64125,#64126,#64127,#64128,#64129,
#64130,#64131,#64132,#64133,#64134,#64135,#64136,#64137,#64138,#64139,#64140,
#64141,#64142,#64143,#64144,#64145,#64146,#64147,#64148,#64149,#64150,#64151,
#64152,#64153,#64154,#64155,#64156,#64157,#64158,#64159,#64160,#64161,#64162,
#64163,#64164,#64165,#64166,#64167,#64168,#64169,#64170,#64171,#64172,#64173),
 .UNSPECIFIED.,.F.,.F.,(4,2,2,2,2,2,2,2,2,2,2,2,2,2,2,2,2,2,2,2,2,2,2,2,
2,2,2,2,2,2,2,2,2,2,2,2,2,2,2,2,2,2,2,2,2,2,2,2,2,2,2,2,2,2,2,2,2,2,2,2,
2,2,2,2,2,2,2,2,2,2,2,2,2,2,2,2,2,2,2,2,2,2,2,2,2,2,2,2,2,2,2,2,2,2,2,2,
2,2,2,2,2,2,2,2,2,2,2,2,2,2,2,2,2,2,2,2,2,2,2,2,2,2,2,2,2,2,2,2,4),(-1.42837807589884,
-1.42524134414718,-1.42130813240249,-1.4180338660253,-1.41366302047601,
-1.40349121065487,-1.38825241851016,-1.33081896982025,-1.31295448713341,
-1.30580980368273,-1.29990690633567,-1.29380061282707,-1.28455822691273,
-1.25250836612072,-1.22510254701366,-1.19334907132251,-1.18561256150371,
-1.18168016668658,-1.17840559590932,-1.1740327817962,-1.16384836766296,
-1.14858228631447,-1.09386815109252,-1.07400654788409,-1.06580502126933,
-1.0599519619398,-1.05376722256114,-1.04413333325148,-1.00487797354269,
-0.964842987353306,-0.949216328408684,-0.943974538163219,-0.940900334670229,
-0.937452237205509,-0.9320336659137,-0.913155522800388,-0.869411685162678,
-0.837208113905973,-0.827743078855024,-0.82159245586301,-0.815652141982764,
-0.807284453152251,-0.784587988878946,-0.74400716229303,-0.711368328351309,
-0.705227638905959,-0.701624644024069,-0.698250872939404,-0.693203493137969,
-0.678085781538767,-0.613110999641547,-0.594332994057977,-0.587089214396346,
-0.581700420395482,-0.575725715152555,-0.567166528349918,-0.542801010319937,
-0.495627918297755,-0.471287683708212,-0.465364240543545,-0.461807880295868,
-0.458404978616514,-0.453207183529864,-0.436688279963417,-0.400032391087145,
-0.361885768785443,-0.35047887588711,-0.343867454283116,-0.338131314186896,
-0.330856719093743,-0.315630638434211,-0.294432454928553,-0.266719019019359,
-0.23483058153165,-0.227099407511814,-0.22316818432982,-0.220012930508764,
-0.219915748223137,-0.219825304576007,-0.21974064895348,-0.219660996951698,
-0.219585694081227,-0.219514188689558,-0.219446011404488,-0.219380759368339,
-0.219318083946978,-0.219257681068282,-0.219199283527306,-0.219142654786388,
-0.219087583953101,-0.219033881682199,-0.218981376761157,-0.218929913270291,
-0.218879348220789,-0.218829549545364,-0.218780394341606,-0.218731767403464,
-0.218683559903509,-0.218635668294907,-0.218587993259698,-0.218540438778011,
-0.218492911321806,-0.218445319092736,-0.218397571275159,-0.218349577330781,
-0.218301246341939,-0.218252486377718,-0.218203203830066,-0.218153302741946,
-0.218102684134915,-0.218051245310653,-0.217998879108618,-0.217945473125218,
-0.217890908873052,-0.217835060861853,-0.217777795598811,-0.21771897052681,
-0.217658432817669,-0.213752607898776,-0.207664338282858,-0.195609598126315,
-0.157343946092611,-0.118770999978118,-0.109091642139302,-0.102897455692032,
-0.0969826916772131,-0.0887638153535705,-0.0672701948442808,-0.000695735724638068),
 .UNSPECIFIED.);
#1438=B_SPLINE_CURVE_WITH_KNOTS('',3,(#64174,#64175,#64176,#64177,#64178,
#64179,#64180,#64181,#64182,#64183,#64184,#64185,#64186),.UNSPECIFIED.,
 .F.,.F.,(4,3,3,3,4),(84.4517779076862,84.5517966727696,84.6519945647983,
84.7462011119194,84.8230016469244),.UNSPECIFIED.);
#1439=B_SPLINE_CURVE_WITH_KNOTS('',3,(#64187,#64188,#64189,#64190,#64191,
#64192,#64193,#64194,#64195,#64196,#64197,#64198,#64199,#64200,#64201,#64202,
#64203,#64204,#64205,#64206,#64207,#64208,#64209,#64210,#64211,#64212,#64213,
#64214,#64215,#64216,#64217,#64218,#64219,#64220,#64221,#64222,#64223,#64224,
#64225,#64226,#64227,#64228,#64229,#64230,#64231,#64232,#64233,#64234,#64235,
#64236,#64237,#64238,#64239,#64240,#64241,#64242,#64243,#64244,#64245,#64246,
#64247,#64248,#64249,#64250,#64251,#64252,#64253,#64254,#64255,#64256,#64257,
#64258,#64259,#64260,#64261,#64262,#64263,#64264,#64265,#64266,#64267,#64268,
#64269,#64270,#64271,#64272,#64273,#64274,#64275,#64276,#64277,#64278,#64279,
#64280,#64281,#64282,#64283,#64284,#64285,#64286,#64287,#64288,#64289,#64290,
#64291,#64292,#64293,#64294,#64295,#64296,#64297,#64298,#64299,#64300,#64301,
#64302,#64303,#64304,#64305,#64306,#64307,#64308,#64309,#64310,#64311,#64312,
#64313,#64314,#64315,#64316,#64317,#64318,#64319,#64320,#64321,#64322,#64323,
#64324,#64325,#64326,#64327,#64328,#64329,#64330,#64331,#64332,#64333,#64334,
#64335,#64336,#64337,#64338,#64339,#64340,#64341,#64342,#64343,#64344,#64345,
#64346,#64347,#64348,#64349,#64350,#64351,#64352,#64353,#64354,#64355,#64356,
#64357,#64358,#64359,#64360,#64361,#64362,#64363,#64364,#64365,#64366,#64367,
#64368,#64369,#64370,#64371,#64372,#64373,#64374,#64375,#64376,#64377,#64378),
 .UNSPECIFIED.,.F.,.F.,(4,2,2,2,2,2,2,2,2,2,2,2,2,2,2,2,2,2,2,2,2,2,2,2,
2,2,2,2,2,2,2,2,2,2,2,2,2,2,2,2,2,2,2,2,2,2,2,2,2,2,2,2,2,2,2,2,2,2,2,2,
2,2,2,2,2,2,2,2,2,2,2,2,2,2,2,2,2,2,2,2,2,2,2,2,2,2,2,2,2,2,2,2,2,2,2,4),
(-4.46296054289888,-4.44334705562705,-4.43404958348456,-4.4279339977854,
-4.4220417148616,-4.41360295271457,-4.39210733336086,-4.33129100598783,
-4.31574691641167,-4.31065281438645,-4.30727088869646,-4.30368466750205,
-4.29761940742059,-4.26965358527184,-4.22553039061928,-4.20189355904667,
-4.19341755216622,-4.18745911162837,-4.1820576493129,-4.17475514689521,
-4.15535293696579,-4.09969282609683,-4.08454065386224,-4.07441075898397,
-4.07004747387351,-4.06677453186116,-4.06283750502988,-4.05507384244125,
-4.02286684187405,-3.99444982727113,-3.9637589638796,-3.95461776879782,
-3.94853266601384,-3.94261675738436,-3.93541467699021,-3.91712302935526,
-3.86004411962012,-3.84490421262699,-3.83477986048366,-3.83041731575201,
-3.82714424698754,-3.82320623065312,-3.81567453892662,-3.77796710796068,
-3.7406733280058,-3.727412380208,-3.71661043407204,-3.71018666307565,-3.70436187545414,
-3.69673534282109,-3.67939117588751,-3.65370241978786,-3.60144741373858,
-3.59393639821687,-3.59000256049281,-3.58672873562954,-3.5823597260441,
-3.57219686335738,-3.55697695049393,-3.52313994985118,-3.48554327900528,
-3.47588776628478,-3.46969888990834,-3.4637822578494,-3.45554938069427,
-3.4339423864121,-3.39751237417951,-3.36202029706523,-3.35429261997151,
-3.35036226778842,-3.34741659053971,-3.34323984950171,-3.33419959664806,
-3.32129278327236,-3.27671388122,-3.245388391687,-3.23598020646377,-3.22984124494449,
-3.22389387981815,-3.21548499296537,-3.19244091168747,-3.15061029285033,
-3.11963174995708,-3.11349842670924,-3.10989711780091,-3.1065227494267,
-3.10147147976953,-3.08631828945336,-3.02152848276922,-3.00261668519787,
-2.99536362704613,-2.98997293614038,-2.98400108874955,-2.97545597721663,
-2.95121688859845,-2.94580181291742),.UNSPECIFIED.);
#1440=B_SPLINE_CURVE_WITH_KNOTS('',3,(#64383,#64384,#64385,#64386,#64387,
#64388,#64389,#64390,#64391,#64392,#64393,#64394,#64395,#64396,#64397,#64398,
#64399,#64400,#64401,#64402,#64403,#64404,#64405,#64406,#64407,#64408,#64409,
#64410,#64411,#64412,#64413,#64414,#64415,#64416,#64417,#64418,#64419,#64420,
#64421,#64422,#64423,#64424,#64425,#64426,#64427,#64428,#64429,#64430,#64431,
#64432,#64433,#64434,#64435,#64436,#64437,#64438,#64439,#64440,#64441,#64442,
#64443,#64444,#64445,#64446,#64447,#64448,#64449,#64450,#64451,#64452,#64453,
#64454,#64455,#64456,#64457,#64458,#64459,#64460,#64461,#64462,#64463,#64464,
#64465,#64466,#64467,#64468,#64469,#64470,#64471,#64472,#64473,#64474,#64475,
#64476,#64477,#64478,#64479,#64480,#64481,#64482,#64483,#64484,#64485,#64486,
#64487,#64488,#64489,#64490,#64491,#64492,#64493,#64494,#64495,#64496,#64497,
#64498,#64499,#64500,#64501,#64502,#64503,#64504,#64505,#64506,#64507,#64508,
#64509,#64510,#64511,#64512,#64513,#64514,#64515,#64516,#64517,#64518,#64519,
#64520,#64521,#64522,#64523,#64524,#64525,#64526,#64527,#64528,#64529,#64530,
#64531,#64532,#64533,#64534,#64535,#64536,#64537,#64538,#64539,#64540,#64541,
#64542,#64543,#64544,#64545,#64546,#64547,#64548,#64549,#64550,#64551,#64552,
#64553,#64554,#64555,#64556,#64557,#64558,#64559,#64560,#64561,#64562,#64563,
#64564,#64565,#64566,#64567,#64568,#64569,#64570,#64571,#64572),
 .UNSPECIFIED.,.F.,.F.,(4,2,2,2,2,2,2,2,2,2,2,2,2,2,2,2,2,2,2,2,2,2,2,2,
2,2,2,2,2,2,2,2,2,2,2,2,2,2,2,2,2,2,2,2,2,2,2,2,2,2,2,2,2,2,2,2,2,2,2,2,
2,2,2,2,2,2,2,2,2,2,2,2,2,2,2,2,2,2,2,2,2,2,2,2,2,2,2,2,2,2,2,2,2,2,4),
(-2.94523236784797,-2.89412897057835,-2.87585892680347,-2.87199687465583,
-2.86442055324781,-2.86427548969014,-2.86414119233107,-2.8640166129821,
-2.86390082307732,-2.86379299865036,-2.85946083256039,-2.85620259674313,
-2.85227043674791,-2.84453338318664,-2.80990801160753,-2.77348898574701,
-2.75124899808426,-2.7429277620191,-2.73698705154369,-2.73080646540264,
-2.72123196771318,-2.68678242039236,-2.64530585489749,-2.6268780382423,
-2.62148894264644,-2.61803956528082,-2.61495270216126,-2.60965455558554,
-2.59354306914457,-2.54939496425623,-2.51456920830108,-2.50515264440698,
-2.49901148643024,-2.49313194344047,-2.48608479983668,-2.46852256403455,
-2.40160359846132,-2.38652379516422,-2.38148159343967,-2.37811005343167,
-2.37451002517544,-2.36837267859651,-2.33537605226832,-2.30873130461617,
-2.27476673196577,-2.26540624945676,-2.2592811113331,-2.25340260469101,
-2.24502423249094,-2.22394696151315,-2.16259905988378,-2.14701373847534,
-2.14191748829202,-2.13853666780573,-2.1349518515119,-2.12889534515261,
-2.10118564852403,-2.05686040946996,-2.03317154616355,-2.02468740468876,
-2.01872546561648,-2.01332215921277,-2.00461593107362,-1.98074941512188,
-1.92327105220116,-1.90749275391143,-1.90237124624896,-1.89898250999011,
-1.89584940771864,-1.89029635207755,-1.87150069347068,-1.82516514819071,
-1.79499290309654,-1.78589146527955,-1.77981369910301,-1.77389070552113,
-1.7666621346104,-1.74809801522878,-1.68280577363384,-1.66768216522862,
-1.66263425357083,-1.65926069278246,-1.65565859713215,-1.64952080810449,
-1.61707659581354,-1.57640063968567,-1.56100285568651,-1.54891789362754,
-1.542233720371,-1.53645116631866,-1.52925403651798,-1.51780712372874,-1.46891882869467,
-1.4329837807736,-1.42837807589884),.UNSPECIFIED.);
#1441=B_SPLINE_CURVE_WITH_KNOTS('',3,(#64573,#64574,#64575,#64576,#64577,
#64578,#64579,#64580,#64581,#64582,#64583,#64584,#64585,#64586,#64587,#64588,
#64589,#64590,#64591,#64592,#64593,#64594,#64595,#64596,#64597,#64598,#64599,
#64600,#64601,#64602,#64603,#64604,#64605,#64606,#64607,#64608,#64609,#64610,
#64611,#64612,#64613,#64614,#64615,#64616,#64617,#64618,#64619,#64620,#64621,
#64622,#64623,#64624,#64625,#64626,#64627,#64628,#64629,#64630,#64631,#64632,
#64633,#64634,#64635,#64636,#64637,#64638,#64639,#64640,#64641,#64642,#64643,
#64644,#64645,#64646,#64647,#64648,#64649,#64650,#64651,#64652,#64653,#64654,
#64655,#64656,#64657,#64658,#64659,#64660,#64661,#64662,#64663,#64664,#64665,
#64666,#64667,#64668,#64669,#64670,#64671,#64672,#64673,#64674,#64675,#64676,
#64677,#64678,#64679,#64680,#64681,#64682,#64683,#64684,#64685,#64686,#64687,
#64688,#64689,#64690,#64691,#64692,#64693,#64694,#64695,#64696,#64697,#64698,
#64699,#64700,#64701,#64702,#64703,#64704,#64705,#64706,#64707,#64708,#64709,
#64710,#64711,#64712,#64713,#64714,#64715,#64716,#64717,#64718,#64719,#64720,
#64721,#64722,#64723,#64724,#64725,#64726,#64727,#64728,#64729,#64730,#64731,
#64732,#64733,#64734,#64735,#64736,#64737,#64738,#64739,#64740,#64741,#64742,
#64743,#64744,#64745,#64746,#64747,#64748,#64749,#64750,#64751,#64752,#64753,
#64754,#64755,#64756,#64757,#64758,#64759,#64760),.UNSPECIFIED.,.F.,.F.,
(4,2,2,2,2,2,2,2,2,2,2,2,2,2,2,2,2,2,2,2,2,2,2,2,2,2,2,2,2,2,2,2,2,2,2,
2,2,2,2,2,2,2,2,2,2,2,2,2,2,2,2,2,2,2,2,2,2,2,2,2,2,2,2,2,2,2,2,2,2,2,2,
2,2,2,2,2,2,2,2,2,2,2,2,2,2,2,2,2,2,2,2,2,2,4),(-2.94580181291742,-2.90460817499543,
-2.87957057982993,-2.87362279539053,-2.87006135467304,-2.86666243233881,
-2.86148378575859,-2.84514975103675,-2.80769388954017,-2.76699648150796,
-2.75710869117688,-2.75087233969347,-2.74498008002403,-2.73689442948782,
-2.71641315089111,-2.67954814378088,-2.64288082941598,-2.63531715777725,
-2.63137219105095,-2.62809941468957,-2.62374530387194,-2.61367391329442,
-2.59864989086835,-2.54036867173092,-2.52282693656846,-2.51573252499838,
-2.50984227131804,-2.50371957771023,-2.49439260272701,-2.46107579791063,
-2.4347056638658,-2.40330639069313,-2.39558813285142,-2.39165958686182,
-2.38838478073055,-2.38400740923458,-2.37379534298358,-2.35847022784197,
-2.32342084827458,-2.28715451827096,-2.27752768260669,-2.27134423055541,
-2.2654236152994,-2.25716992115575,-2.23540234331792,-2.19902855419543,
-2.16368967106783,-2.15595854697814,-2.1520273602556,-2.14908177966834,
-2.14490607103522,-2.1358707893209,-2.1229737375826,-2.07847633986276,-2.04705775273901,
-2.03764330338641,-2.031503338738,-2.02555727575551,-2.01715417805907,-1.99415698908484,
-1.95249960551774,-1.92128425609789,-1.91514975410334,-1.91154833581123,
-1.90817433469293,-1.90312451294921,-1.88798375021566,-1.82275564409671,
-1.80417786895916,-1.79694843026936,-1.79102493033042,-1.78494694635427,
-1.77584597289201,-1.74569901618576,-1.69954658479955,-1.68050149940176,
-1.67491384650807,-1.67142947861358,-1.66796604998943,-1.66248058532875,
-1.64281917099795,-1.59458126778472,-1.56697662497112,-1.55790248733235,
-1.55243492120172,-1.54652696657721,-1.53835637895877,-1.51724841161208,
-1.48062542995621,-1.44468151589752,-1.43693716097271,-1.43300316341903,
-1.4297307922503,-1.42845765518849),.UNSPECIFIED.);
#1442=B_SPLINE_CURVE_WITH_KNOTS('',3,(#64764,#64765,#64766,#64767,#64768,
#64769,#64770,#64771,#64772,#64773,#64774,#64775,#64776,#64777,#64778,#64779,
#64780,#64781,#64782,#64783,#64784,#64785,#64786,#64787,#64788,#64789,#64790,
#64791,#64792,#64793,#64794,#64795,#64796,#64797,#64798,#64799,#64800,#64801,
#64802,#64803,#64804,#64805,#64806,#64807,#64808,#64809,#64810,#64811,#64812,
#64813,#64814,#64815,#64816,#64817,#64818,#64819,#64820,#64821,#64822,#64823,
#64824,#64825,#64826,#64827,#64828,#64829,#64830,#64831,#64832,#64833),
 .UNSPECIFIED.,.F.,.F.,(4,3,3,3,3,3,3,3,3,3,3,3,3,3,3,3,3,3,3,3,3,3,3,4),
(-4.05574753316386,-3.96990054887667,-3.87574120014698,-3.78170877927821,
-3.68777526208839,-3.59390997284874,-3.50007964416114,-3.4062590961083,
-3.3124231640359,-3.21849032913891,-3.1245041690831,-3.03037165160513,-2.9774254116575,
-2.88380029281574,-2.79029953948074,-2.69318460824238,-2.59984389426094,
-2.50653282197543,-2.41322559184539,-2.31989641457199,-2.22646577718421,
-2.1329748240063,-2.03934284451356,-2.01338008957384),.UNSPECIFIED.);
#1443=B_SPLINE_CURVE_WITH_KNOTS('',3,(#64837,#64838,#64839,#64840,#64841),
 .UNSPECIFIED.,.F.,.F.,(4,1,4),(0.,0.992475137219176,1.09916241472585),
 .UNSPECIFIED.);
#1444=B_SPLINE_CURVE_WITH_KNOTS('',3,(#64843,#64844,#64845,#64846,#64847,
#64848,#64849,#64850,#64851,#64852,#64853,#64854,#64855,#64856,#64857,#64858,
#64859,#64860,#64861,#64862,#64863,#64864,#64865,#64866,#64867,#64868,#64869,
#64870,#64871,#64872,#64873,#64874,#64875,#64876,#64877,#64878,#64879,#64880,
#64881,#64882,#64883,#64884,#64885,#64886,#64887,#64888,#64889,#64890,#64891,
#64892,#64893,#64894,#64895,#64896,#64897,#64898,#64899,#64900,#64901,#64902,
#64903,#64904,#64905,#64906,#64907,#64908,#64909,#64910,#64911,#64912,#64913,
#64914,#64915,#64916,#64917,#64918,#64919,#64920,#64921,#64922,#64923,#64924,
#64925,#64926,#64927,#64928,#64929,#64930,#64931,#64932,#64933,#64934,#64935,
#64936,#64937,#64938,#64939,#64940,#64941,#64942,#64943,#64944,#64945,#64946,
#64947,#64948,#64949,#64950,#64951,#64952,#64953,#64954,#64955,#64956,#64957,
#64958,#64959,#64960,#64961,#64962,#64963,#64964,#64965,#64966,#64967,#64968,
#64969,#64970,#64971,#64972,#64973,#64974,#64975,#64976,#64977,#64978,#64979,
#64980,#64981,#64982,#64983,#64984,#64985,#64986,#64987,#64988,#64989,#64990,
#64991,#64992,#64993,#64994,#64995,#64996,#64997,#64998,#64999,#65000,#65001,
#65002,#65003,#65004,#65005,#65006,#65007,#65008,#65009,#65010,#65011,#65012,
#65013,#65014,#65015,#65016,#65017,#65018,#65019,#65020,#65021,#65022,#65023,
#65024,#65025,#65026,#65027,#65028,#65029,#65030,#65031,#65032,#65033,#65034,
#65035,#65036,#65037,#65038,#65039,#65040,#65041,#65042,#65043,#65044,#65045,
#65046,#65047,#65048,#65049,#65050,#65051,#65052,#65053),.UNSPECIFIED.,
 .F.,.F.,(4,3,3,3,3,3,3,3,3,3,3,3,3,3,3,3,3,3,3,3,3,3,3,3,3,3,3,3,3,3,3,
3,3,3,3,3,3,3,3,3,3,3,3,3,3,3,3,3,3,3,3,3,3,3,3,3,3,3,3,3,3,3,3,3,3,3,3,
3,3,3,4),(1.09916241472585,1.19108189997564,1.28288257485515,1.37459207473264,
1.46625293783966,1.55789236719196,1.64953753678025,1.74127307032638,1.83305681701207,
1.92499004688988,1.98495027443835,2.07904726479922,2.17301758138154,2.26688931662874,
2.36069352084906,2.45446321554417,2.54822364236444,2.64200002812979,2.73587451626984,
2.82980292430621,2.92387915370253,2.97742541165751,3.07156802140755,3.16558709693299,
3.25951064804815,3.3533710377344,3.44719960305778,3.54102152138864,3.63486195742961,
3.72880403951816,3.82280214187751,3.91695071813298,3.96990054887668,4.06378056215249,
4.15753260692621,4.25118509216546,4.34476952351686,4.43831921063563,4.531859673343,
4.62541641671787,4.71907310930614,4.81278444856287,4.9066469062787,4.96237568609585,
5.05638711968008,5.15027213667652,5.24405895441764,5.3377791926669,5.43146554874222,
5.52514337660817,5.61883801603108,5.71263258107009,5.80648198314815,5.90048144632545,
5.95485082331501,6.04885731394597,6.14273765631534,6.23652007325052,6.3302363411792,
6.42391899533065,6.51759339540272,6.61128488712475,6.70507675502254,6.7989237106116,
6.89292115016949,6.94732596053418,7.0492143061606,7.15073816485904,7.25202703522367,
7.35297873667727,7.38234742361043),.UNSPECIFIED.);
#1445=B_SPLINE_CURVE_WITH_KNOTS('',3,(#65055,#65056,#65057,#65058,#65059,
#65060,#65061,#65062,#65063,#65064),.UNSPECIFIED.,.F.,.F.,(4,1,1,1,1,1,
1,4),(7.38234772190543,7.93980109775335,8.93227623497251,9.92475137219169,
10.9172265094109,11.90970164663,12.9021767838492,13.6655327805175),
 .UNSPECIFIED.);
#1446=B_SPLINE_CURVE_WITH_KNOTS('',3,(#65066,#65067,#65068,#65069,#65070,
#65071,#65072,#65073,#65074,#65075,#65076,#65077,#65078,#65079,#65080,#65081,
#65082,#65083,#65084,#65085,#65086,#65087,#65088,#65089,#65090,#65091,#65092,
#65093,#65094,#65095,#65096,#65097,#65098,#65099,#65100,#65101,#65102,#65103,
#65104,#65105,#65106,#65107,#65108,#65109,#65110,#65111,#65112,#65113,#65114,
#65115,#65116,#65117,#65118,#65119,#65120,#65121,#65122,#65123,#65124,#65125,
#65126,#65127,#65128,#65129,#65130,#65131,#65132,#65133,#65134,#65135,#65136,
#65137,#65138,#65139,#65140,#65141,#65142,#65143,#65144,#65145,#65146,#65147,
#65148,#65149,#65150,#65151,#65152,#65153,#65154,#65155,#65156,#65157,#65158,
#65159,#65160,#65161,#65162,#65163,#65164,#65165,#65166,#65167,#65168,#65169,
#65170,#65171,#65172,#65173,#65174,#65175,#65176,#65177,#65178,#65179,#65180,
#65181,#65182,#65183,#65184,#65185,#65186,#65187,#65188,#65189,#65190,#65191,
#65192,#65193,#65194,#65195,#65196,#65197,#65198,#65199,#65200,#65201,#65202,
#65203,#65204,#65205,#65206,#65207,#65208,#65209,#65210,#65211,#65212,#65213,
#65214,#65215,#65216,#65217,#65218,#65219,#65220,#65221,#65222,#65223,#65224,
#65225,#65226,#65227,#65228,#65229,#65230,#65231,#65232,#65233,#65234,#65235,
#65236,#65237,#65238,#65239,#65240,#65241,#65242,#65243,#65244,#65245,#65246,
#65247,#65248,#65249,#65250,#65251,#65252,#65253,#65254,#65255,#65256,#65257,
#65258,#65259,#65260,#65261,#65262,#65263,#65264,#65265,#65266,#65267,#65268,
#65269,#65270,#65271,#65272,#65273),.UNSPECIFIED.,.F.,.F.,(4,3,3,3,3,3,
3,3,3,3,3,3,3,3,3,3,3,3,3,3,3,3,3,3,3,3,3,3,3,3,3,3,3,3,3,3,3,3,3,3,3,3,
3,3,3,3,3,3,3,3,3,3,3,3,3,3,3,3,3,3,3,3,3,3,3,3,3,3,3,4),(13.665533029085,
13.7908310334317,13.8946519210684,13.988641850667,14.0825052861128,14.1762704756524,
14.2699691086556,14.363633882415,14.4572901782299,14.5509633632484,14.6447367251609,
14.7385650352236,14.8325437909839,14.8871270582875,14.9811168910591,15.0749802289659,
15.1687453203954,15.2624438548513,15.3561085298316,15.4497647267587,15.5434378129045,
15.6372110765735,15.7310392886046,15.8250179476368,15.8796021955067,15.9735919886998,
16.0674552860834,16.1612203361062,16.2549188280051,16.3485834597327,16.442239612763,
16.5359126544189,16.6296858729579,16.7235140394316,16.8174926526751,16.8720773327259,
16.966067173307,17.0599305187923,17.1536956175594,17.2473941589593,17.341058840637,
17.4347150440056,17.5283881363271,17.6221614057251,17.7159896232411,17.8099682873159,
17.864552469945,17.9585422943882,18.0524056235837,18.1461707059327,18.2398692307921,
18.33353389586,18.4271900825701,18.5208631582051,18.6146364109757,18.7084646118734,
18.8024432595083,18.8570276071642,18.9510174282501,19.0448807539868,19.1386458327808,
19.232344353956,19.3260090152612,19.4196651981345,19.5133382698629,19.6071115186433,
19.700939715498,19.7949183590452,19.8495027443834,19.9487183362646),
 .UNSPECIFIED.);
#1447=B_SPLINE_CURVE_WITH_KNOTS('',3,(#65275,#65276,#65277,#65278,#65279,
#65280,#65281,#65282,#65283,#65284,#65285,#65286,#65287,#65288,#65289,#65290,
#65291,#65292,#65293,#65294,#65295,#65296,#65297,#65298,#65299,#65300,#65301,
#65302,#65303,#65304,#65305,#65306,#65307,#65308,#65309,#65310,#65311,#65312,
#65313,#65314,#65315,#65316,#65317,#65318,#65319,#65320,#65321,#65322,#65323,
#65324,#65325,#65326,#65327,#65328,#65329,#65330,#65331,#65332,#65333,#65334,
#65335,#65336,#65337,#65338,#65339,#65340,#65341,#65342,#65343,#65344,#65345,
#65346,#65347,#65348,#65349,#65350,#65351,#65352,#65353,#65354,#65355,#65356,
#65357,#65358,#65359,#65360,#65361,#65362,#65363,#65364,#65365,#65366,#65367,
#65368,#65369,#65370,#65371,#65372,#65373,#65374,#65375,#65376,#65377,#65378,
#65379,#65380,#65381,#65382,#65383,#65384,#65385,#65386,#65387,#65388,#65389,
#65390,#65391,#65392,#65393,#65394,#65395,#65396,#65397,#65398,#65399,#65400,
#65401,#65402,#65403,#65404,#65405,#65406,#65407,#65408,#65409,#65410,#65411,
#65412,#65413,#65414,#65415,#65416,#65417,#65418,#65419,#65420,#65421,#65422,
#65423,#65424,#65425,#65426,#65427,#65428,#65429,#65430,#65431,#65432,#65433,
#65434,#65435,#65436,#65437,#65438,#65439,#65440,#65441,#65442,#65443,#65444,
#65445,#65446,#65447,#65448,#65449,#65450,#65451,#65452,#65453,#65454,#65455,
#65456,#65457,#65458,#65459,#65460,#65461,#65462,#65463,#65464,#65465,#65466,
#65467,#65468,#65469,#65470,#65471,#65472,#65473,#65474,#65475,#65476,#65477,
#65478,#65479,#65480,#65481,#65482,#65483,#65484,#65485),.UNSPECIFIED.,
 .F.,.F.,(4,3,3,3,3,3,3,3,3,3,3,3,3,3,3,3,3,3,3,3,3,3,3,3,3,3,3,3,3,3,3,
3,3,3,3,3,3,3,3,3,3,3,3,3,3,3,3,3,3,3,3,3,3,3,3,3,3,3,3,3,3,3,3,3,3,3,3,
3,3,3,4),(19.9487183364793,20.0414927127207,20.1341536551306,20.2267293285119,
20.3192599426483,20.4117721022213,20.5042923885719,20.5969045224113,20.6895660174233,
20.7823763144016,20.8419778816025,20.9359677062525,21.0298310356222,21.1235961181127,
21.2172946430643,21.3109593081937,21.4046154949344,21.4982885705689,21.5920618232911,
21.6858900241134,21.7798686716303,21.8344530188217,21.9284428432923,22.0223061724728,
22.1160712547648,22.209769779504,22.3034344444127,22.3970906309247,22.4907637063224,
22.5845369587974,22.678365159366,22.7723438066217,22.8269281560409,22.9209179812708,
23.0147813112232,23.1085463942984,23.2022449198351,23.2959095855495,23.3895657728746,
23.4832388490922,23.5770121023914,23.6708403037884,23.7648189518703,23.8194032932601,
23.9133931181127,24.0072564476835,24.1010215303731,24.1947200555196,24.2883847208415,
24.3820409077721,24.4757139835937,24.569487236497,24.6633154374973,24.7572940851858,
24.8118784304792,24.9058682553442,24.9997315849265,25.0934966676268,25.1871951927831,
25.2808598581141,25.374516045053,25.4681891208814,25.5619623737908,25.6557905747963,
25.7497692224888,25.8043535676984,25.9112410865558,26.0132189365589,26.1149468961578,
26.216320556494,26.2319036431278),.UNSPECIFIED.);
#1448=B_SPLINE_CURVE_WITH_KNOTS('',3,(#65487,#65488,#65489,#65490,#65491,
#65492,#65493,#65494,#65495,#65496,#65497,#65498,#65499,#65500,#65501,#65502,
#65503,#65504,#65505,#65506,#65507,#65508,#65509,#65510,#65511,#65512,#65513,
#65514,#65515,#65516,#65517,#65518,#65519,#65520,#65521,#65522,#65523,#65524,
#65525,#65526,#65527,#65528,#65529,#65530,#65531,#65532,#65533,#65534,#65535,
#65536,#65537,#65538,#65539,#65540,#65541,#65542,#65543,#65544,#65545,#65546,
#65547,#65548,#65549,#65550,#65551,#65552,#65553,#65554,#65555,#65556,#65557,
#65558,#65559,#65560,#65561,#65562,#65563,#65564,#65565,#65566,#65567,#65568,
#65569,#65570,#65571,#65572,#65573,#65574,#65575,#65576,#65577,#65578,#65579,
#65580,#65581,#65582,#65583,#65584,#65585,#65586,#65587,#65588,#65589,#65590,
#65591,#65592,#65593,#65594,#65595,#65596,#65597,#65598,#65599,#65600,#65601,
#65602,#65603,#65604,#65605,#65606,#65607,#65608,#65609,#65610,#65611,#65612,
#65613,#65614,#65615,#65616,#65617,#65618,#65619,#65620,#65621,#65622,#65623,
#65624,#65625,#65626,#65627,#65628,#65629,#65630,#65631,#65632,#65633,#65634,
#65635,#65636,#65637,#65638,#65639,#65640,#65641,#65642,#65643,#65644,#65645,
#65646,#65647,#65648,#65649,#65650,#65651,#65652,#65653,#65654,#65655,#65656,
#65657,#65658,#65659,#65660,#65661,#65662,#65663,#65664,#65665,#65666,#65667,
#65668,#65669,#65670,#65671,#65672,#65673,#65674,#65675,#65676,#65677,#65678,
#65679,#65680,#65681,#65682,#65683,#65684,#65685,#65686,#65687,#65688,#65689,
#65690,#65691,#65692,#65693,#65694,#65695,#65696,#65697),.UNSPECIFIED.,
 .F.,.F.,(4,3,3,3,3,3,3,3,3,3,3,3,3,3,3,3,3,3,3,3,3,3,3,3,3,3,3,3,3,3,3,
3,3,3,3,3,3,3,3,3,3,3,3,3,3,3,3,3,3,3,3,3,3,3,3,3,3,3,3,3,3,3,3,3,3,3,3,
3,3,3,4),(26.2319036434442,26.3276115682817,26.423375181536,26.519294850849,
26.6152944080368,26.7114937996171,26.7968287049176,26.8908185298198,26.9846818594401,
27.0784469421796,27.1721454673759,27.2658101327474,27.3594663197274,27.4531393955981,
27.54691264855,27.6407408495986,27.7347194973344,27.7893038421367,27.8832936670454,
27.9771569966723,28.0709220794184,28.164620604621,28.2582852699989,28.3519414569851,
28.4456145328617,28.5393877858197,28.6332159868743,28.7271946346159,28.7817789793559,
28.8757688042752,28.9696321339128,29.0633972166698,29.1570957418837,29.2507604072728,
29.3444165942707,29.4380896701591,29.5318629231286,29.625691124195,29.7196697719483,
29.7742541165751,29.8682439414868,29.9621072711167,30.0558723538656,30.1495708790716,
30.2432355444527,30.3368917314425,30.4305648073228,30.5243380602843,30.6181662613425,
30.7121449090877,30.7667292537942,30.8607190787074,30.954582408339,31.0483474910895,
31.142046016297,31.2357106816797,31.3293668686707,31.4230399445526,31.5168131975156,
31.6106413985755,31.7046200463222,31.7592043910134,31.8536899609647,31.9463790432336,
32.0389818453475,32.1315250528619,32.2274160273024,32.3199469364277,32.4124932923736,
32.5051109026203,32.5150889506238),.UNSPECIFIED.);
#1449=B_SPLINE_CURVE_WITH_KNOTS('',3,(#65699,#65700,#65701,#65702,#65703,
#65704,#65705,#65706,#65707,#65708,#65709),.UNSPECIFIED.,.F.,.F.,(4,1,1,
1,1,1,1,1,4),(32.5150893692119,32.7516795282326,33.7441546654517,34.7366298026709,
35.7291049398901,36.7215800771092,37.7140552143284,38.7065303515476,38.7982742578034),
 .UNSPECIFIED.);
#1450=B_SPLINE_CURVE_WITH_KNOTS('',3,(#65711,#65712,#65713,#65714,#65715,
#65716,#65717,#65718,#65719,#65720,#65721,#65722,#65723,#65724,#65725,#65726,
#65727,#65728,#65729,#65730,#65731,#65732,#65733,#65734,#65735,#65736,#65737,
#65738,#65739,#65740,#65741,#65742,#65743,#65744,#65745,#65746,#65747,#65748,
#65749,#65750,#65751,#65752,#65753,#65754,#65755,#65756,#65757,#65758,#65759,
#65760,#65761,#65762,#65763,#65764,#65765,#65766,#65767,#65768,#65769,#65770,
#65771,#65772,#65773,#65774,#65775,#65776,#65777,#65778,#65779,#65780,#65781,
#65782,#65783,#65784,#65785,#65786,#65787,#65788,#65789,#65790,#65791,#65792,
#65793,#65794,#65795,#65796,#65797,#65798,#65799,#65800,#65801,#65802,#65803,
#65804,#65805,#65806,#65807,#65808,#65809,#65810,#65811,#65812,#65813,#65814,
#65815,#65816,#65817,#65818,#65819,#65820,#65821,#65822,#65823,#65824,#65825,
#65826,#65827,#65828,#65829,#65830,#65831,#65832,#65833,#65834,#65835,#65836,
#65837,#65838,#65839,#65840,#65841,#65842,#65843,#65844,#65845,#65846,#65847,
#65848,#65849,#65850,#65851,#65852,#65853,#65854,#65855,#65856,#65857,#65858,
#65859,#65860,#65861,#65862,#65863,#65864,#65865,#65866,#65867,#65868,#65869,
#65870,#65871,#65872,#65873,#65874,#65875,#65876,#65877,#65878,#65879,#65880,
#65881,#65882,#65883,#65884,#65885,#65886,#65887,#65888,#65889,#65890,#65891,
#65892,#65893,#65894,#65895,#65896,#65897,#65898,#65899,#65900,#65901,#65902,
#65903,#65904,#65905,#65906,#65907,#65908,#65909,#65910,#65911,#65912,#65913,
#65914,#65915,#65916,#65917,#65918),.UNSPECIFIED.,.F.,.F.,(4,3,3,3,3,3,
3,3,3,3,3,3,3,3,3,3,3,3,3,3,3,3,3,3,3,3,3,3,3,3,3,3,3,3,3,3,3,3,3,3,3,3,
3,3,3,3,3,3,3,3,3,3,3,3,3,3,3,3,3,3,3,3,3,3,3,3,3,3,3,4),(38.7982742578034,
38.8911077810691,38.9838262178453,39.0764570669745,39.1690412837208,39.2616054304404,
39.3541760447021,39.4468376766205,39.5395470952447,39.632407528133,39.6990054887667,
39.7929953136803,39.8868586433119,39.9806237260628,40.0743222512708,40.1679869166541,
40.2616431036457,40.355316179528,40.4490894324914,40.5429176335517,40.636896281299,
40.6914806259859,40.7854704508995,40.8793337805316,40.9730988632824,41.0667973884904,
41.1604620538735,41.2541182408653,41.3477913167472,41.4415645697106,41.5353927707708,
41.6293714185179,41.6839557632051,41.7779455881187,41.8718089177506,41.9655740005019,
42.0592725257098,42.152937191093,42.2465933780846,42.340266453967,42.4340397069304,
42.5278679079905,42.6218465557376,42.6764309004243,42.770420725338,42.8642840549696,
42.9580491377205,43.0517476629285,43.1454123283117,43.2390685153034,43.3327415911854,
43.4265148441489,43.5203430452093,43.6143216929564,43.6689060376434,43.762895862557,
43.8567591921892,43.9505242749404,44.0442228001483,44.1378874655315,44.2315436525232,
44.3252167284053,44.4189899813687,44.5128181824287,44.6067968301759,44.6613811748626,
44.7664007723502,44.8688416746821,44.9751506197477,45.0814595648132),
 .UNSPECIFIED.);
#1451=B_SPLINE_CURVE_WITH_KNOTS('',3,(#65920,#65921,#65922,#65923,#65924,
#65925,#65926,#65927,#65928,#65929,#65930,#65931,#65932,#65933,#65934,#65935,
#65936,#65937,#65938,#65939,#65940,#65941,#65942,#65943,#65944,#65945,#65946,
#65947,#65948,#65949,#65950,#65951,#65952,#65953,#65954,#65955,#65956,#65957,
#65958,#65959,#65960,#65961,#65962,#65963,#65964,#65965,#65966,#65967,#65968,
#65969,#65970,#65971,#65972,#65973,#65974,#65975,#65976,#65977,#65978,#65979,
#65980,#65981,#65982,#65983,#65984,#65985,#65986,#65987,#65988,#65989,#65990,
#65991,#65992,#65993,#65994,#65995,#65996,#65997,#65998,#65999,#66000,#66001,
#66002,#66003,#66004,#66005,#66006,#66007,#66008,#66009,#66010,#66011,#66012,
#66013,#66014,#66015,#66016,#66017,#66018,#66019,#66020,#66021,#66022,#66023,
#66024,#66025,#66026,#66027,#66028,#66029,#66030,#66031,#66032,#66033,#66034,
#66035,#66036,#66037,#66038,#66039,#66040,#66041,#66042,#66043,#66044,#66045,
#66046,#66047,#66048,#66049,#66050,#66051,#66052,#66053,#66054,#66055,#66056,
#66057,#66058,#66059,#66060,#66061,#66062,#66063,#66064,#66065,#66066,#66067,
#66068,#66069,#66070,#66071,#66072,#66073,#66074,#66075,#66076,#66077,#66078,
#66079,#66080,#66081,#66082,#66083,#66084,#66085,#66086,#66087,#66088,#66089,
#66090,#66091,#66092,#66093,#66094,#66095,#66096,#66097,#66098,#66099,#66100,
#66101,#66102,#66103,#66104,#66105,#66106,#66107,#66108,#66109,#66110,#66111,
#66112,#66113,#66114,#66115,#66116,#66117,#66118,#66119,#66120,#66121,#66122,
#66123,#66124,#66125,#66126,#66127),.UNSPECIFIED.,.F.,.F.,(4,3,3,3,3,3,
3,3,3,3,3,3,3,3,3,3,3,3,3,3,3,3,3,3,3,3,3,3,3,3,3,3,3,3,3,3,3,3,3,3,3,3,
3,3,3,3,3,3,3,3,3,3,3,3,3,3,3,3,3,3,3,3,3,3,3,3,3,3,3,4),(45.081459564983,
45.1769592542972,45.2725075662283,45.3682050177821,45.4639772739664,45.5599488925284,
45.6538563120818,45.7478461369954,45.8417094666272,45.9354745493782,46.0291730745861,
46.1228377399692,46.2164939269609,46.310167002843,46.4039402558063,46.4977684568664,
46.5917471046135,46.6463314493009,46.7403212742146,46.8341846038464,46.9279496865972,
47.0216482118051,47.1153128771883,47.2089690641801,47.3026421400624,47.3964153930259,
47.4902435940862,47.5842222418335,47.6388065865201,47.7327964114337,47.8266597410655,
47.9204248238163,48.0141233490243,48.1077880144075,48.2014442013991,48.2951172772811,
48.3888905302445,48.4827187313046,48.5766973790517,48.6312817237393,48.7252715486528,
48.8191348782849,48.9128999610356,49.0065984862435,49.1002631516265,49.1939193386183,
49.2875924145003,49.3813656674637,49.4751938685238,49.569172516271,49.6237568609584,
49.717746685872,49.811610015504,49.9053750982546,49.9990736234626,50.0927382888457,
50.1863944758373,50.28006755172,50.3738408046834,50.4676690057437,50.5616476534909,
50.6162319981776,50.7097836074257,50.8025276215215,50.8951845324334,50.9877809804665,
51.0819969533905,51.1745774864197,51.2696111792911,51.3646448721626),
 .UNSPECIFIED.);
#1452=B_SPLINE_CURVE_WITH_KNOTS('',3,(#66129,#66130,#66131,#66132,#66133,
#66134,#66135,#66136,#66137,#66138,#66139),.UNSPECIFIED.,.F.,.F.,(4,1,1,
1,1,1,1,1,4),(51.3646459623497,51.6087071353968,52.601182272616,53.5936574098351,
54.5861325470543,55.5786076842735,56.5710828214926,57.5635579587118,57.6478301793422),
 .UNSPECIFIED.);
#1453=B_SPLINE_CURVE_WITH_KNOTS('',3,(#66141,#66142,#66143,#66144,#66145,
#66146,#66147,#66148,#66149,#66150,#66151,#66152,#66153,#66154,#66155,#66156,
#66157,#66158,#66159,#66160,#66161,#66162,#66163,#66164,#66165,#66166,#66167,
#66168,#66169,#66170,#66171,#66172,#66173,#66174,#66175,#66176,#66177,#66178,
#66179,#66180,#66181,#66182,#66183,#66184,#66185,#66186,#66187,#66188,#66189,
#66190,#66191,#66192,#66193,#66194,#66195,#66196,#66197,#66198,#66199,#66200,
#66201,#66202,#66203,#66204,#66205,#66206,#66207,#66208,#66209,#66210,#66211,
#66212,#66213,#66214,#66215,#66216,#66217,#66218,#66219,#66220,#66221,#66222,
#66223,#66224,#66225,#66226,#66227,#66228,#66229,#66230,#66231,#66232,#66233,
#66234,#66235,#66236,#66237,#66238,#66239,#66240,#66241,#66242,#66243,#66244,
#66245,#66246,#66247,#66248,#66249,#66250,#66251,#66252,#66253,#66254,#66255,
#66256,#66257,#66258,#66259,#66260,#66261,#66262,#66263,#66264,#66265,#66266,
#66267,#66268,#66269,#66270,#66271,#66272,#66273,#66274,#66275,#66276,#66277,
#66278,#66279,#66280,#66281,#66282,#66283,#66284,#66285,#66286,#66287,#66288,
#66289,#66290,#66291,#66292,#66293,#66294,#66295,#66296,#66297,#66298,#66299,
#66300,#66301,#66302,#66303,#66304,#66305,#66306,#66307,#66308,#66309,#66310,
#66311,#66312,#66313,#66314,#66315,#66316,#66317,#66318,#66319,#66320,#66321,
#66322,#66323,#66324,#66325,#66326,#66327,#66328,#66329,#66330,#66331,#66332,
#66333,#66334,#66335,#66336,#66337,#66338,#66339,#66340,#66341,#66342,#66343,
#66344,#66345,#66346,#66347,#66348),.UNSPECIFIED.,.F.,.F.,(4,3,3,3,3,3,
3,3,3,3,3,3,3,3,3,3,3,3,3,3,3,3,3,3,3,3,3,3,3,3,3,3,3,3,3,3,3,3,3,3,3,3,
3,3,3,3,3,3,3,3,3,3,3,3,3,3,3,3,3,3,3,3,3,3,3,3,3,3,3,4),(57.6478301793422,
57.7407280669645,57.8335093047544,57.9262007371352,58.0188440325848,58.1114657054143,
58.2040922438032,58.2968090105251,58.3895720306128,58.4824883121618,58.556033095931,
58.6500229208446,58.7438862504766,58.8376513332274,58.9313498584353,59.0250145238185,
59.1186707108101,59.2123437866921,59.3061170396555,59.3999452407157,59.4939238884629,
59.5485082331501,59.6424980580633,59.7363613876947,59.8301264704455,59.9238249956531,
60.017489661036,60.1111458480273,60.2048189239094,60.2985921768725,60.3924203779325,
60.4863990256793,60.5409833703693,60.6349731952839,60.7288365249167,60.8226016076682,
60.9163001328769,61.0099647982609,61.1036209852534,61.1972940611366,61.2910673141008,
61.3848955151621,61.4788741629101,61.5334585075885,61.6274483325016,61.7213116621329,
61.8150767448828,61.9087752700902,62.0024399354729,62.0960961224641,62.1897691983459,
62.2835424513088,62.3773706523686,62.4713493001154,62.5259336448076,62.6199234697194,
62.713786799349,62.8075518820985,62.9012504073045,62.9949150726858,63.0885712596754,
63.1822443355558,63.2760175885173,63.3698457895758,63.4638244373211,63.5184087820268,
63.6215975387392,63.7245199877336,63.8277677370369,63.9310154863402),
 .UNSPECIFIED.);
#1454=B_SPLINE_CURVE_WITH_KNOTS('',3,(#66350,#66351,#66352,#66353,#66354,
#66355,#66356,#66357,#66358,#66359,#66360,#66361,#66362,#66363,#66364,#66365,
#66366,#66367,#66368,#66369,#66370,#66371,#66372,#66373,#66374,#66375,#66376,
#66377,#66378,#66379,#66380,#66381,#66382,#66383,#66384,#66385,#66386,#66387,
#66388,#66389,#66390,#66391,#66392,#66393,#66394,#66395,#66396,#66397,#66398,
#66399,#66400,#66401,#66402,#66403,#66404,#66405,#66406,#66407,#66408,#66409,
#66410,#66411,#66412,#66413,#66414,#66415,#66416,#66417,#66418,#66419,#66420,
#66421,#66422,#66423,#66424,#66425,#66426,#66427,#66428,#66429,#66430,#66431,
#66432,#66433,#66434,#66435,#66436,#66437,#66438,#66439,#66440,#66441,#66442,
#66443,#66444,#66445,#66446,#66447,#66448,#66449,#66450,#66451,#66452,#66453,
#66454,#66455,#66456,#66457,#66458,#66459,#66460,#66461,#66462,#66463,#66464,
#66465,#66466,#66467,#66468,#66469,#66470,#66471,#66472,#66473,#66474,#66475,
#66476,#66477,#66478,#66479,#66480,#66481,#66482,#66483,#66484,#66485,#66486,
#66487,#66488,#66489,#66490,#66491,#66492,#66493,#66494,#66495,#66496,#66497,
#66498,#66499,#66500,#66501,#66502,#66503,#66504,#66505,#66506,#66507,#66508,
#66509,#66510,#66511,#66512,#66513,#66514,#66515,#66516,#66517,#66518,#66519,
#66520,#66521,#66522,#66523,#66524,#66525,#66526,#66527,#66528,#66529,#66530,
#66531,#66532,#66533,#66534,#66535,#66536,#66537,#66538,#66539,#66540,#66541,
#66542,#66543,#66544,#66545,#66546,#66547,#66548,#66549,#66550,#66551,#66552,
#66553,#66554,#66555,#66556,#66557),.UNSPECIFIED.,.F.,.F.,(4,3,3,3,3,3,
3,3,3,3,3,3,3,3,3,3,3,3,3,3,3,3,3,3,3,3,3,3,3,3,3,3,3,3,3,3,3,3,3,3,3,3,
3,3,3,3,3,3,3,3,3,3,3,3,3,3,3,3,3,3,3,3,3,3,3,3,3,3,3,4),(63.9310154865217,
64.0263152239147,64.1216568579874,64.2189636233021,64.3145192288704,64.4127015740582,
64.510883919246,64.6048737441539,64.6987370737801,64.7925021565253,64.8862006817278,
64.9798653471056,65.0735215340919,65.1671946099688,65.260967862927,65.3547960639822,
65.4487747117244,65.5033590564651,65.5973488813674,65.6912122109878,65.7849772937273,
65.8786758189237,65.9723404842952,66.0659966712754,66.1596697471461,66.2534430000979,
66.3472712011466,66.4412498488823,66.4958341936843,66.5898240186435,66.6836873483209,
66.7774524311176,66.8711509563712,66.9648156217999,67.058471808837,67.1521448847643,
67.2459181377723,67.3397463388767,67.4337249866672,67.4883093309035,67.5822991557625,
67.6761624853401,67.7699275680371,67.8636260931917,67.9572907585219,68.0509469454611,
68.1446200212909,68.2383932742035,68.3322214752134,68.4262001229117,68.4807844681226,
68.5747742929777,68.6686376225504,68.7624027052413,68.8561012303887,68.9497658957111,
69.0434220826416,69.1370951584623,69.2308684113642,69.324696612363,69.4186752600488,
69.4732596053418,69.5661785353861,69.65898289471,69.751699366492,69.8443545393512,
69.9370009516695,70.0296366765961,70.1223440423424,70.2142007937013),
 .UNSPECIFIED.);
#1455=B_SPLINE_CURVE_WITH_KNOTS('',3,(#66559,#66560,#66561,#66562,#66563,
#66564,#66565,#66566,#66567,#66568,#66569,#66570,#66571,#66572,#66573,#66574,
#66575,#66576,#66577,#66578,#66579,#66580,#66581,#66582,#66583,#66584,#66585,
#66586,#66587,#66588,#66589,#66590,#66591,#66592,#66593,#66594,#66595,#66596,
#66597,#66598,#66599,#66600,#66601,#66602,#66603,#66604,#66605,#66606,#66607,
#66608,#66609,#66610,#66611,#66612,#66613,#66614,#66615,#66616,#66617,#66618,
#66619,#66620,#66621,#66622,#66623,#66624,#66625,#66626,#66627,#66628,#66629,
#66630,#66631,#66632,#66633,#66634,#66635,#66636,#66637,#66638,#66639,#66640,
#66641,#66642,#66643,#66644,#66645,#66646,#66647,#66648,#66649,#66650,#66651,
#66652,#66653,#66654,#66655,#66656,#66657,#66658,#66659,#66660,#66661,#66662,
#66663,#66664,#66665,#66666,#66667,#66668,#66669,#66670,#66671,#66672,#66673,
#66674,#66675,#66676,#66677,#66678,#66679,#66680,#66681,#66682,#66683,#66684,
#66685,#66686,#66687,#66688,#66689,#66690,#66691,#66692,#66693,#66694,#66695,
#66696,#66697,#66698,#66699,#66700,#66701,#66702,#66703,#66704,#66705,#66706,
#66707,#66708,#66709,#66710,#66711,#66712,#66713,#66714,#66715,#66716,#66717,
#66718,#66719,#66720,#66721,#66722,#66723,#66724,#66725,#66726,#66727,#66728,
#66729,#66730,#66731,#66732,#66733,#66734,#66735,#66736,#66737,#66738,#66739,
#66740,#66741,#66742,#66743,#66744,#66745,#66746,#66747,#66748,#66749,#66750,
#66751,#66752,#66753,#66754,#66755,#66756,#66757,#66758,#66759,#66760,#66761,
#66762,#66763,#66764,#66765,#66766,#66767,#66768,#66769),.UNSPECIFIED.,
 .F.,.F.,(4,3,3,3,3,3,3,3,3,3,3,3,3,3,3,3,3,3,3,3,3,3,3,3,3,3,3,3,3,3,3,
3,3,3,3,3,3,3,3,3,3,3,3,3,3,3,3,3,3,3,3,3,3,3,3,3,3,3,3,3,3,3,3,3,3,3,3,
3,3,3,4),(70.2142007939207,70.3334640590779,70.4552451164889,70.465734742561,
70.5597245669846,70.6535878961274,70.7473529783913,70.8410515031168,70.9347161680207,
71.0283723545367,71.1220454299474,71.2158186824487,71.3096468830513,71.4036255303524,
71.4582098797801,71.552199704465,71.6460630338625,71.7398281163739,71.8335266413357,
71.9271913064686,72.0208474932064,72.1145205688314,72.2082938215339,72.302122022331,
72.3961006698139,72.4506850169993,72.544674844279,72.6385381762844,72.732303261413,
72.826001788995,72.919666456749,73.0133226461056,73.1069957243438,73.2007689796352,
73.2945971830111,73.3885758330317,73.4431601542185,73.5371499749457,73.6310133003967,
73.724778378978,73.8184769000496,73.9121415613188,74.0057977442235,74.0994708160508,
74.1932440650325,74.2870722621464,74.3810509060418,74.4356352914376,74.5296251162456,
74.6234884457315,74.7172535282968,74.8109520532614,74.9046167183659,74.9982729050441,
75.0919459805785,75.1857192331444,75.2795474337786,75.3735260810593,75.4281104286568,
75.5221002698313,75.6159636157889,75.709728714908,75.8034272564792,75.8970919382164,
75.9907481415329,76.0844212336906,76.1781945027555,76.2720227198425,76.366001383341,
76.420585565876,76.4973861008809),.UNSPECIFIED.);
#1456=B_SPLINE_CURVE_WITH_KNOTS('',3,(#66771,#66772,#66773,#66774,#66775,
#66776,#66777,#66778,#66779,#66780),.UNSPECIFIED.,.F.,.F.,(4,1,1,1,1,1,
1,4),(76.4973940480353,77.4130607030951,78.4055358403143,79.3980109775335,
80.3904861147527,81.3829612519718,82.375436389191,82.780565175451),
 .UNSPECIFIED.);
#1457=B_SPLINE_CURVE_WITH_KNOTS('',3,(#66782,#66783,#66784,#66785,#66786,
#66787,#66788,#66789,#66790,#66791,#66792,#66793,#66794,#66795,#66796,#66797,
#66798,#66799,#66800,#66801,#66802,#66803,#66804,#66805,#66806,#66807,#66808,
#66809,#66810,#66811,#66812,#66813,#66814,#66815,#66816,#66817,#66818,#66819,
#66820,#66821,#66822,#66823,#66824,#66825,#66826,#66827,#66828,#66829,#66830,
#66831,#66832,#66833,#66834,#66835,#66836,#66837,#66838,#66839,#66840,#66841,
#66842,#66843,#66844,#66845,#66846,#66847,#66848,#66849,#66850,#66851,#66852,
#66853,#66854,#66855,#66856,#66857,#66858,#66859,#66860,#66861,#66862,#66863,
#66864,#66865,#66866,#66867,#66868,#66869,#66870,#66871,#66872,#66873,#66874,
#66875,#66876,#66877,#66878,#66879,#66880,#66881,#66882,#66883,#66884,#66885,
#66886,#66887,#66888,#66889,#66890,#66891,#66892,#66893,#66894,#66895,#66896,
#66897,#66898,#66899,#66900,#66901,#66902,#66903,#66904,#66905,#66906,#66907,
#66908,#66909,#66910,#66911,#66912,#66913,#66914,#66915,#66916,#66917,#66918,
#66919,#66920,#66921,#66922,#66923,#66924,#66925,#66926,#66927,#66928,#66929,
#66930,#66931,#66932,#66933,#66934,#66935,#66936,#66937,#66938,#66939,#66940,
#66941,#66942,#66943,#66944,#66945,#66946,#66947,#66948,#66949,#66950,#66951,
#66952,#66953,#66954,#66955,#66956,#66957,#66958,#66959,#66960,#66961,#66962,
#66963,#66964,#66965,#66966,#66967,#66968,#66969,#66970,#66971,#66972,#66973,
#66974,#66975,#66976,#66977,#66978,#66979,#66980,#66981,#66982,#66983,#66984,
#66985,#66986,#66987,#66988,#66989,#66990,#66991,#66992),.UNSPECIFIED.,
 .F.,.F.,(4,3,3,3,3,3,3,3,3,3,3,3,3,3,3,3,3,3,3,3,3,3,3,3,3,3,3,3,3,3,3,
3,3,3,3,3,3,3,3,3,3,3,3,3,3,3,3,3,3,3,3,3,3,3,3,3,3,3,3,3,3,3,3,3,3,3,3,
3,3,3,4),(82.7805714080605,82.8756769963287,82.9708180774348,83.0700914396786,
83.165437152978,83.2608693513861,83.3564641921791,83.3679115264102,83.461903274698,
83.5557685153425,83.6495354943892,83.7432358864185,83.8369023997384,83.9305604136443,
84.0242352932622,84.1180103039131,84.211840239249,84.3058205675134,84.3603866636293,
84.4543804594747,84.5482477945329,84.6420169113679,84.7357194963243,84.8293882357292,
84.9230485059173,85.0167256690785,85.110502990458,85.2043352552119,85.2983179190271,
85.3528618008485,85.4468357700119,85.5406832175902,85.6344324134189,85.7281151096413,
85.8217639877295,85.9154044481434,86.0090618772467,86.1028196996842,86.1966325696502,
86.2905961935937,86.3453369380677,86.4393455013607,86.5332274937779,86.6270111399809,
86.720728005926,86.8144108676545,86.9080850852006,87.0017760043043,87.0955667082914,
87.1894121644862,87.28340759052,87.3378120752868,87.4318226025838,87.5257068980905,
87.6194931783374,87.7132131551182,87.806899420454,87.900577328163,87.9942722180067,
88.0880672920136,88.1819173497577,88.2759176933972,88.330287212506,88.4231787283098,
88.515954847165,88.6086422726807,88.701267612456,88.7938817763749,88.8864846860942,
88.9791544786862,89.0637567152401),.UNSPECIFIED.);
#1458=B_SPLINE_CURVE_WITH_KNOTS('',3,(#66994,#66995,#66996,#66997,#66998,
#66999,#67000,#67001,#67002,#67003,#67004,#67005,#67006,#67007,#67008,#67009,
#67010,#67011,#67012,#67013,#67014,#67015,#67016,#67017,#67018,#67019,#67020,
#67021,#67022,#67023,#67024,#67025,#67026,#67027,#67028,#67029,#67030,#67031,
#67032,#67033,#67034,#67035,#67036,#67037,#67038,#67039,#67040,#67041,#67042,
#67043,#67044,#67045,#67046,#67047,#67048,#67049,#67050,#67051,#67052,#67053,
#67054,#67055,#67056,#67057,#67058,#67059,#67060,#67061,#67062,#67063,#67064,
#67065,#67066,#67067,#67068,#67069),.UNSPECIFIED.,.F.,.F.,(4,3,3,3,3,3,
3,3,3,3,3,3,3,3,3,3,3,3,3,3,3,3,3,3,3,4),(89.063756715403,89.1813412978231,
89.3011841336904,89.3227623497252,89.4169215726789,89.5109538690648,89.6048872632074,
89.6987524320014,89.7925826418988,89.8864030729481,89.9802388899363,90.074171613325,
90.1681576637385,90.262290075529,90.3152374869443,90.4088618846611,90.5023619137458,
90.5994770169613,90.6928170034203,90.7861273482923,90.8794338519026,90.9727623043365,
91.0661922230418,91.159682460239,91.253313733231,91.2792827394697),
 .UNSPECIFIED.);
#1459=B_SPLINE_CURVE_WITH_KNOTS('',3,(#67073,#67074,#67075,#67076,#67077),
 .UNSPECIFIED.,.F.,.F.,(4,1,4),(-93.2926628986018,-92.3001877613827,-92.0203418336781),
 .UNSPECIFIED.);
#1460=B_SPLINE_CURVE_WITH_KNOTS('',3,(#67079,#67080,#67081,#67082,#67083,
#67084,#67085,#67086,#67087,#67088),.UNSPECIFIED.,.F.,.F.,(4,1,1,1,1,1,
1,4),(-92.0203418336781,-91.3077126241635,-90.3152374869444,-89.3227623497252,
-88.330287212506,-87.3378120752868,-86.3453369380677,-85.7371565264985),
 .UNSPECIFIED.);
#1461=B_SPLINE_CURVE_WITH_KNOTS('',3,(#67090,#67091,#67092,#67093,#67094,
#67095,#67096,#67097,#67098,#67099,#67100,#67101,#67102,#67103,#67104,#67105,
#67106,#67107,#67108,#67109,#67110,#67111,#67112,#67113,#67114,#67115,#67116,
#67117,#67118,#67119,#67120,#67121,#67122,#67123,#67124,#67125,#67126,#67127,
#67128,#67129,#67130,#67131,#67132,#67133,#67134,#67135,#67136,#67137,#67138,
#67139,#67140,#67141,#67142,#67143,#67144,#67145,#67146,#67147,#67148,#67149,
#67150,#67151,#67152,#67153,#67154,#67155,#67156,#67157,#67158,#67159,#67160,
#67161,#67162,#67163,#67164,#67165,#67166,#67167,#67168,#67169,#67170,#67171,
#67172,#67173,#67174,#67175,#67176,#67177,#67178,#67179,#67180,#67181,#67182,
#67183,#67184,#67185,#67186,#67187,#67188,#67189,#67190,#67191,#67192,#67193,
#67194,#67195,#67196,#67197,#67198,#67199,#67200,#67201,#67202,#67203,#67204,
#67205,#67206,#67207,#67208,#67209,#67210,#67211,#67212,#67213,#67214,#67215,
#67216,#67217,#67218,#67219,#67220,#67221,#67222,#67223,#67224,#67225,#67226,
#67227,#67228,#67229,#67230,#67231,#67232,#67233,#67234,#67235,#67236,#67237,
#67238,#67239,#67240,#67241,#67242,#67243,#67244,#67245,#67246,#67247,#67248,
#67249,#67250,#67251,#67252,#67253,#67254,#67255,#67256,#67257,#67258,#67259,
#67260,#67261,#67262,#67263,#67264,#67265,#67266,#67267,#67268,#67269,#67270,
#67271,#67272,#67273,#67274,#67275,#67276,#67277,#67278,#67279,#67280,#67281,
#67282,#67283,#67284,#67285,#67286,#67287,#67288,#67289,#67290,#67291,#67292,
#67293,#67294,#67295,#67296,#67297),.UNSPECIFIED.,.F.,.F.,(4,3,3,3,3,3,
3,3,3,3,3,3,3,3,3,3,3,3,3,3,3,3,3,3,3,3,3,3,3,3,3,3,3,3,3,3,3,3,3,3,3,3,
3,3,3,3,3,3,3,3,3,3,3,3,3,3,3,3,3,3,3,3,3,3,3,3,3,3,3,4),(-85.7371563039944,
-85.632809300152,-85.5280804819151,-85.4228292623581,-85.3528618008485,
-85.2588679527554,-85.1650005706409,-85.0712314119546,-84.9775287930657,
-84.8838600246363,-84.7901997303596,-84.6965225480777,-84.6027452152697,
-84.5089129434122,-84.4149302793837,-84.3603866636294,-84.2663951665026,
-84.1725301249216,-84.0787632930732,-83.9850629704441,-83.8913964784107,
-83.7977384377239,-83.704063483264,-83.6102883249328,-83.5164582005907,
-83.4224776200041,-83.3679115264102,-83.273923687219,-83.1800623731564,
-83.0862993328493,-82.9926028817128,-82.8989403091757,-82.8052862312469,
-82.7116152780994,-82.6178441559045,-82.5240180932625,-82.430041575035,
-82.375436389191,-82.2814458914497,-82.1875818826862,-82.0938161154856,
-82.0001169007732,-81.9064515430276,-81.8127946616749,-81.7191208902913,
-81.6253469443368,-81.5315180506916,-81.4375387178315,-81.3829612519718,
-81.2889712841214,-81.1951078072733,-81.1013425732528,-81.0076438913324,
-80.9139790659265,-80.8203227157901,-80.7266494738271,-80.6328760512805,
-80.5390476784111,-80.4450688570051,-80.3904861147527,-80.2972774958163,
-80.2041947611772,-80.1104168184663,-80.0174951058634,-79.9246039336365,
-79.8317170561381,-79.7372805969761,-79.6442735644754,-79.5491223919828,
-79.4539712194903),.UNSPECIFIED.);
#1462=B_SPLINE_CURVE_WITH_KNOTS('',3,(#67299,#67300,#67301,#67302,#67303,
#67304,#67305,#67306,#67307,#67308,#67309,#67310,#67311,#67312,#67313,#67314,
#67315,#67316,#67317,#67318,#67319,#67320,#67321,#67322,#67323,#67324,#67325,
#67326,#67327,#67328,#67329,#67330,#67331,#67332,#67333,#67334,#67335,#67336,
#67337,#67338,#67339,#67340,#67341,#67342,#67343,#67344,#67345,#67346,#67347,
#67348,#67349,#67350,#67351,#67352,#67353,#67354,#67355,#67356,#67357,#67358,
#67359,#67360,#67361,#67362,#67363,#67364,#67365,#67366,#67367,#67368,#67369,
#67370,#67371,#67372,#67373,#67374,#67375,#67376,#67377,#67378,#67379,#67380,
#67381,#67382,#67383,#67384,#67385,#67386,#67387,#67388,#67389,#67390,#67391,
#67392,#67393,#67394,#67395,#67396,#67397,#67398,#67399,#67400,#67401,#67402,
#67403,#67404,#67405,#67406,#67407,#67408,#67409,#67410,#67411,#67412,#67413,
#67414,#67415,#67416,#67417,#67418,#67419,#67420,#67421,#67422,#67423,#67424,
#67425,#67426,#67427,#67428,#67429,#67430,#67431,#67432,#67433,#67434,#67435,
#67436,#67437,#67438,#67439,#67440,#67441,#67442,#67443,#67444,#67445,#67446,
#67447,#67448,#67449,#67450,#67451,#67452,#67453,#67454,#67455,#67456,#67457,
#67458,#67459,#67460,#67461,#67462,#67463,#67464,#67465,#67466,#67467,#67468,
#67469,#67470,#67471,#67472,#67473,#67474,#67475,#67476,#67477,#67478,#67479,
#67480,#67481,#67482,#67483,#67484,#67485,#67486,#67487,#67488,#67489,#67490,
#67491,#67492,#67493,#67494,#67495,#67496,#67497,#67498,#67499,#67500,#67501,
#67502,#67503,#67504,#67505,#67506,#67507,#67508,#67509),.UNSPECIFIED.,
 .F.,.F.,(4,3,3,3,3,3,3,3,3,3,3,3,3,3,3,3,3,3,3,3,3,3,3,3,3,3,3,3,3,3,3,
3,3,3,3,3,3,3,3,3,3,3,3,3,3,3,3,3,3,3,3,3,3,3,3,3,3,3,3,3,3,3,3,3,3,3,3,
3,3,3,4),(-79.4539712193189,-79.3980109775335,-79.3040210470638,-79.2101576107371,
-79.1163924203078,-79.0226937864058,-78.9290290117422,-78.835372715019,
-78.7416995290889,-78.6479261662656,-78.5540978552912,-78.4601190986269,
-78.4055358403143,-78.3115460075673,-78.2176826696829,-78.123917578274,
-78.0302190438356,-77.936554368871,-77.8428981719575,-77.7492250858235,
-77.6554518221633,-77.5616236101392,-77.4676449511111,-77.4130607030952,
-77.3190709101445,-77.2252076130074,-77.1314425632348,-77.0377440715906,
-76.9440794401205,-76.85042328735,-76.756750245956,-76.6629770276805,-76.5691488614716,
-76.4751702484923,-76.420585565876,-76.3265957251464,-76.2327323795108,
-76.1389672805919,-76.0452687390383,-75.9516040572061,-75.857947853682,
-75.7642747612044,-75.6705014916504,-75.576673273978,-75.4826946097481,
-75.4281104286568,-75.3341206042293,-75.2402572750495,-75.1464921927161,
-75.0527936678719,-74.959129002819,-74.8654728161236,-74.7717997405032,
-74.6780264877467,-74.5841982868627,-74.4902196392412,-74.4356352914376,
-74.3416454703856,-74.2477821446834,-74.1540170659243,-74.0603185447847,
-73.9666538835156,-73.8729977006788,-73.7793246289871,-73.6855513802437,
-73.5917231834264,-73.4977445399164,-73.4431601542185,-73.325149510274,
-73.2090479125567,-73.1707860257054),.UNSPECIFIED.);
#1463=B_SPLINE_CURVE_WITH_KNOTS('',3,(#67511,#67512,#67513,#67514,#67515,
#67516,#67517,#67518,#67519,#67520),.UNSPECIFIED.,.F.,.F.,(4,1,1,1,1,1,
1,4),(-73.1707859121394,-72.4506850169993,-71.4582098797801,-70.465734742561,
-69.4732596053418,-68.4807844681226,-67.4883093309035,-66.8876006049598),
 .UNSPECIFIED.);
#1464=B_SPLINE_CURVE_WITH_KNOTS('',3,(#67522,#67523,#67524,#67525,#67526,
#67527,#67528,#67529,#67530,#67531,#67532,#67533,#67534,#67535,#67536,#67537,
#67538,#67539,#67540,#67541,#67542,#67543,#67544,#67545,#67546,#67547,#67548,
#67549,#67550,#67551,#67552,#67553,#67554,#67555,#67556,#67557,#67558,#67559,
#67560,#67561,#67562,#67563,#67564,#67565,#67566,#67567,#67568,#67569,#67570,
#67571,#67572,#67573,#67574,#67575,#67576,#67577,#67578,#67579,#67580,#67581,
#67582,#67583,#67584,#67585,#67586,#67587,#67588,#67589,#67590,#67591,#67592,
#67593,#67594,#67595,#67596,#67597,#67598,#67599,#67600,#67601,#67602,#67603,
#67604,#67605,#67606,#67607,#67608,#67609,#67610,#67611,#67612,#67613,#67614,
#67615,#67616,#67617,#67618,#67619,#67620,#67621,#67622,#67623,#67624,#67625,
#67626,#67627,#67628,#67629,#67630,#67631,#67632,#67633,#67634,#67635,#67636,
#67637,#67638,#67639,#67640,#67641,#67642,#67643,#67644,#67645,#67646,#67647,
#67648,#67649,#67650,#67651,#67652,#67653,#67654,#67655,#67656,#67657,#67658,
#67659,#67660,#67661,#67662,#67663,#67664,#67665,#67666,#67667,#67668,#67669,
#67670,#67671,#67672,#67673,#67674,#67675,#67676,#67677,#67678,#67679,#67680,
#67681,#67682,#67683,#67684,#67685,#67686,#67687,#67688,#67689,#67690,#67691,
#67692,#67693,#67694,#67695,#67696,#67697,#67698,#67699,#67700,#67701,#67702,
#67703,#67704,#67705,#67706,#67707,#67708,#67709,#67710,#67711,#67712,#67713,
#67714,#67715,#67716,#67717,#67718,#67719,#67720,#67721,#67722,#67723,#67724,
#67725,#67726,#67727,#67728,#67729),.UNSPECIFIED.,.F.,.F.,(4,3,3,3,3,3,
3,3,3,3,3,3,3,3,3,3,3,3,3,3,3,3,3,3,3,3,3,3,3,3,3,3,3,3,3,3,3,3,3,3,3,3,
3,3,3,3,3,3,3,3,3,3,3,3,3,3,3,3,3,3,3,3,3,3,3,3,3,3,3,4),(-66.8876003895016,
-66.7837700712268,-66.6795867770187,-66.5749020761923,-66.4958341936843,
-66.4018443687823,-66.3079810391619,-66.2142159564225,-66.1205174312264,
-66.0268527658549,-65.933196578875,-65.8395235030045,-65.7457502500528,
-65.6519220490043,-65.5579434012686,-65.5033590564651,-65.4093692315565,
-65.3155059019297,-65.221740819184,-65.1280422939814,-65.0343776286037,
-64.9407214416174,-64.8470483657408,-64.753275112783,-64.6594469117285,
-64.565468263987,-64.510883919246,-64.4168940943267,-64.3230307646889,-64.229265681932,
-64.1355671567181,-64.0419024913288,-63.9482463043309,-63.8545732284425,
-63.7607999754729,-63.6669717744064,-63.572993126653,-63.5184087820268,
-63.4244189571151,-63.3305556274852,-63.2367905447362,-63.1430920195302,
-63.049427354149,-62.9557711671592,-62.862098091279,-62.7683248383175,-62.6744966372593,
-62.580517989514,-62.5259336448076,-62.4319438198945,-62.3380804902631,
-62.2443154075127,-62.1506168823053,-62.0569522169226,-61.9632960299315,
-61.8696229540498,-61.7758497010869,-61.6820215000272,-61.5880428522806,
-61.5334585075885,-61.4403288883763,-61.3473250707808,-61.2544247374575,
-61.1615812526724,-61.0687682618145,-60.9759594442223,-60.8830700660323,
-60.7901426869388,-60.6970626347649,-60.6044152979652),.UNSPECIFIED.);
#1465=B_SPLINE_CURVE_WITH_KNOTS('',3,(#67731,#67732,#67733,#67734,#67735,
#67736,#67737,#67738,#67739,#67740,#67741,#67742,#67743,#67744,#67745,#67746,
#67747,#67748,#67749,#67750,#67751,#67752,#67753,#67754,#67755,#67756,#67757,
#67758,#67759,#67760,#67761,#67762,#67763,#67764,#67765,#67766,#67767,#67768,
#67769,#67770,#67771,#67772,#67773,#67774,#67775,#67776,#67777,#67778,#67779,
#67780,#67781,#67782,#67783,#67784,#67785,#67786,#67787,#67788,#67789,#67790,
#67791,#67792,#67793,#67794,#67795,#67796,#67797,#67798,#67799,#67800,#67801,
#67802,#67803,#67804,#67805,#67806,#67807,#67808,#67809,#67810,#67811,#67812,
#67813,#67814,#67815,#67816,#67817,#67818,#67819,#67820,#67821,#67822,#67823,
#67824,#67825,#67826,#67827,#67828,#67829,#67830,#67831,#67832,#67833,#67834,
#67835,#67836,#67837,#67838,#67839,#67840,#67841,#67842,#67843,#67844,#67845,
#67846,#67847,#67848,#67849,#67850,#67851,#67852,#67853,#67854,#67855,#67856,
#67857,#67858,#67859,#67860,#67861,#67862,#67863,#67864,#67865,#67866,#67867,
#67868,#67869,#67870,#67871,#67872,#67873,#67874,#67875,#67876,#67877,#67878,
#67879,#67880,#67881,#67882,#67883,#67884,#67885,#67886,#67887,#67888,#67889,
#67890,#67891,#67892,#67893,#67894,#67895,#67896,#67897,#67898,#67899,#67900,
#67901,#67902,#67903,#67904,#67905,#67906,#67907,#67908,#67909,#67910,#67911,
#67912,#67913,#67914,#67915,#67916,#67917,#67918,#67919,#67920,#67921,#67922,
#67923,#67924,#67925,#67926,#67927,#67928,#67929,#67930,#67931,#67932,#67933,
#67934,#67935,#67936,#67937,#67938,#67939,#67940,#67941),.UNSPECIFIED.,
 .F.,.F.,(4,3,3,3,3,3,3,3,3,3,3,3,3,3,3,3,3,3,3,3,3,3,3,3,3,3,3,3,3,3,3,
3,3,3,3,3,3,3,3,3,3,3,3,3,3,3,3,3,3,3,3,3,3,3,3,3,3,3,3,3,3,3,3,3,3,3,3,
3,3,3,4),(-60.6044152977802,-60.5409833703693,-60.4469935454563,-60.3531302158249,
-60.2593651330745,-60.1656666078671,-60.0720019424845,-59.9783457554934,
-59.8846726796118,-59.7908994266489,-59.6970712255893,-59.6030925778426,
-59.5485082331501,-59.4545184082364,-59.3606550786044,-59.2668899958533,
-59.1731914706452,-59.0795268052619,-58.98587061827,-58.8921975423876,-58.7984242894241,
-58.7045960883637,-58.6106174406164,-58.556033095931,-58.4620432710174,
-58.3681799413855,-58.2744148586345,-58.1807163334265,-58.0870516680433,
-57.9933954810515,-57.8997224051692,-57.8059491522057,-57.7121209511454,
-57.6181423033982,-57.5635579587118,-57.4695681337982,-57.3757048041664,
-57.2819397214155,-57.1882411962076,-57.0945765308244,-57.0009203438327,
-56.9072472679505,-56.8134740149871,-56.7196458139269,-56.6256671661798,
-56.5710828214926,-56.477092996579,-56.3832296669472,-56.2894645841962,
-56.1957660589883,-56.1021013936051,-56.0084452066135,-55.9147721307313,
-55.8209988777679,-55.7271706767077,-55.6331920289605,-55.5786076842735,
-55.4846178593599,-55.390754529728,-55.2969894469769,-55.203290921769,-55.1096262563858,
-55.0159700693942,-54.9222969935119,-54.8285237405484,-54.7346955394881,
-54.6407168917409,-54.5861325470543,-54.4668321488865,-54.3496326388445,
-54.3212299907803),.UNSPECIFIED.);
#1466=B_SPLINE_CURVE_WITH_KNOTS('',3,(#67943,#67944,#67945,#67946,#67947,
#67948,#67949,#67950,#67951,#67952,#67953,#67954,#67955,#67956,#67957,#67958,
#67959,#67960,#67961,#67962,#67963,#67964,#67965,#67966,#67967,#67968,#67969,
#67970,#67971,#67972,#67973,#67974,#67975,#67976,#67977,#67978,#67979,#67980,
#67981,#67982,#67983,#67984,#67985,#67986,#67987,#67988,#67989,#67990,#67991,
#67992,#67993,#67994,#67995,#67996,#67997,#67998,#67999,#68000,#68001,#68002,
#68003,#68004,#68005,#68006,#68007,#68008,#68009,#68010,#68011,#68012,#68013,
#68014,#68015,#68016,#68017,#68018,#68019,#68020,#68021,#68022,#68023,#68024,
#68025,#68026,#68027,#68028,#68029,#68030,#68031,#68032,#68033,#68034,#68035,
#68036,#68037,#68038,#68039,#68040,#68041,#68042,#68043,#68044,#68045,#68046,
#68047,#68048,#68049,#68050,#68051,#68052,#68053,#68054,#68055,#68056,#68057,
#68058,#68059,#68060,#68061,#68062,#68063,#68064,#68065,#68066,#68067,#68068,
#68069,#68070,#68071,#68072,#68073,#68074,#68075,#68076,#68077,#68078,#68079,
#68080,#68081,#68082,#68083,#68084,#68085,#68086,#68087,#68088,#68089,#68090,
#68091,#68092,#68093,#68094,#68095,#68096,#68097,#68098,#68099,#68100,#68101,
#68102,#68103,#68104,#68105,#68106,#68107,#68108,#68109,#68110,#68111,#68112,
#68113,#68114,#68115,#68116,#68117,#68118,#68119,#68120,#68121,#68122,#68123,
#68124,#68125,#68126,#68127,#68128,#68129,#68130,#68131,#68132,#68133,#68134,
#68135,#68136,#68137,#68138,#68139,#68140,#68141,#68142,#68143,#68144,#68145,
#68146,#68147,#68148,#68149,#68150,#68151,#68152,#68153),.UNSPECIFIED.,
 .F.,.F.,(4,3,3,3,3,3,3,3,3,3,3,3,3,3,3,3,3,3,3,3,3,3,3,3,3,3,3,3,3,3,3,
3,3,3,3,3,3,3,3,3,3,3,3,3,3,3,3,3,3,3,3,3,3,3,3,3,3,3,3,3,3,3,3,3,3,3,3,
3,3,3,4),(-54.3212299906006,-54.2284183110393,-54.1356537708416,-54.0429099834603,
-53.950160587367,-53.8573191213051,-53.7644310102756,-53.6713864992433,
-53.5936574098351,-53.4996675849215,-53.4058042552895,-53.3120391725386,
-53.2183406473307,-53.1246759819475,-53.0310197949558,-52.9373467190735,
-52.8435734661101,-52.7497452650498,-52.6557666173027,-52.601182272616,
-52.5071924477025,-52.4133291180705,-52.3195640353194,-52.2258655101115,
-52.1322008447283,-52.0385446577366,-51.9448715818547,-51.8510983288913,
-51.757270127831,-51.6632914800839,-51.6087071353968,-51.5147173104833,
-51.4208539808515,-51.3270888981007,-51.2333903728928,-51.1397257075096,
-51.0460695205179,-50.9523964446358,-50.8586231916724,-50.764794990612,
-50.6708163428648,-50.6162319981776,-50.522242173264,-50.4283788436319,
-50.334613760881,-50.240915235673,-50.1472505702897,-50.0535943832979,-49.9599213074159,
-49.8661480544523,-49.772319853392,-49.6783412056449,-49.6237568609584,
-49.5297670360449,-49.4359037064131,-49.3421386236626,-49.2484400984547,
-49.1547754330715,-49.0611192460799,-48.9674461701977,-48.8736729172343,
-48.7798447161742,-48.6858660684269,-48.6312817237393,-48.5358676688867,
-48.4405923974443,-48.3454327805398,-48.2503808034438,-48.1553913922474,
-48.060442494842,-48.038044683421),.UNSPECIFIED.);
#1467=B_SPLINE_CURVE_WITH_KNOTS('',3,(#68155,#68156,#68157,#68158,#68159,
#68160,#68161,#68162,#68163,#68164),.UNSPECIFIED.,.F.,.F.,(4,1,1,1,1,1,
1,4),(-48.0380382192525,-47.6388065865201,-46.6463314493009,-45.6538563120818,
-44.6613811748626,-43.6689060376434,-42.6764309004243,-41.7548670354255),
 .UNSPECIFIED.);
#1468=B_SPLINE_CURVE_WITH_KNOTS('',3,(#68166,#68167,#68168,#68169,#68170,
#68171,#68172,#68173,#68174,#68175,#68176,#68177,#68178,#68179,#68180,#68181,
#68182,#68183,#68184,#68185,#68186,#68187,#68188,#68189,#68190,#68191,#68192,
#68193,#68194,#68195,#68196,#68197,#68198,#68199,#68200,#68201,#68202,#68203,
#68204,#68205,#68206,#68207,#68208,#68209,#68210,#68211,#68212,#68213,#68214,
#68215,#68216,#68217,#68218,#68219,#68220,#68221,#68222,#68223,#68224,#68225,
#68226,#68227,#68228,#68229,#68230,#68231,#68232,#68233,#68234,#68235,#68236,
#68237,#68238,#68239,#68240,#68241,#68242,#68243,#68244,#68245,#68246,#68247,
#68248,#68249,#68250,#68251,#68252,#68253,#68254,#68255,#68256,#68257,#68258,
#68259,#68260,#68261,#68262,#68263,#68264,#68265,#68266,#68267,#68268,#68269,
#68270,#68271,#68272,#68273,#68274,#68275,#68276,#68277,#68278,#68279,#68280,
#68281,#68282,#68283,#68284,#68285,#68286,#68287,#68288,#68289,#68290,#68291,
#68292,#68293,#68294,#68295,#68296,#68297,#68298,#68299,#68300,#68301,#68302,
#68303,#68304,#68305,#68306,#68307,#68308,#68309,#68310,#68311,#68312,#68313,
#68314,#68315,#68316,#68317,#68318,#68319,#68320,#68321,#68322,#68323,#68324,
#68325,#68326,#68327,#68328,#68329,#68330,#68331,#68332,#68333,#68334,#68335,
#68336,#68337,#68338,#68339,#68340,#68341,#68342,#68343,#68344,#68345,#68346,
#68347,#68348,#68349,#68350,#68351,#68352,#68353,#68354,#68355,#68356,#68357,
#68358,#68359,#68360,#68361,#68362,#68363,#68364,#68365,#68366,#68367,#68368,
#68369,#68370,#68371,#68372,#68373,#68374,#68375,#68376),.UNSPECIFIED.,
 .F.,.F.,(4,3,3,3,3,3,3,3,3,3,3,3,3,3,3,3,3,3,3,3,3,3,3,3,3,3,3,3,3,3,3,
3,3,3,3,3,3,3,3,3,3,3,3,3,3,3,3,3,3,3,3,3,3,3,3,3,3,3,3,3,3,3,3,3,3,3,3,
3,3,3,4),(-41.7548593762414,-41.6839557632051,-41.5899659382915,-41.4961026086598,
-41.4023375259089,-41.308639000701,-41.2149743353178,-41.1213181483262,
-41.0276450724441,-40.9338718194807,-40.8400436184206,-40.7460649706734,
-40.6914806259859,-40.5974908010722,-40.5036274714403,-40.4098623886892,
-40.3161638634812,-40.222499198098,-40.1288430111062,-40.0351699352239,
-39.9413966822604,-39.8475684812001,-39.7535898334529,-39.6990054887667,
-39.6050156638532,-39.5111523342213,-39.4173872514704,-39.3236887262625,
-39.2300240608794,-39.1363678738877,-39.0426947980056,-38.9489215450422,
-38.855093343982,-38.7611146962348,-38.7065303515476,-38.612540526634,-38.5186771970021,
-38.4249121142512,-38.3312135890432,-38.2375489236601,-38.1438927366683,
-38.0502196607861,-37.9564464078227,-37.8626182067624,-37.7686395590152,
-37.7140552143284,-37.6200653894147,-37.5262020597829,-37.4324369770319,
-37.3387384518239,-37.2450737864407,-37.151417599449,-37.0577445235668,
-36.9639712706034,-36.8701430695431,-36.7761644217959,-36.7215800771092,
-36.6275902521957,-36.5337269225639,-36.439961839813,-36.3462633146052,
-36.2525986492221,-36.1589424622304,-36.0652693863482,-35.9714961333848,
-35.8776679323247,-35.7836892845776,-35.7291049398901,-35.6084268596164,
-35.4900717265883,-35.4716740693444),.UNSPECIFIED.);
#1469=B_SPLINE_CURVE_WITH_KNOTS('',3,(#68378,#68379,#68380,#68381,#68382,
#68383,#68384,#68385,#68386,#68387,#68388,#68389,#68390,#68391,#68392,#68393,
#68394,#68395,#68396,#68397,#68398,#68399,#68400,#68401,#68402,#68403,#68404,
#68405,#68406,#68407,#68408,#68409,#68410,#68411,#68412,#68413,#68414,#68415,
#68416,#68417,#68418,#68419,#68420,#68421,#68422,#68423,#68424,#68425,#68426,
#68427,#68428,#68429,#68430,#68431,#68432,#68433,#68434,#68435,#68436,#68437,
#68438,#68439,#68440,#68441,#68442,#68443,#68444,#68445,#68446,#68447,#68448,
#68449,#68450,#68451,#68452,#68453,#68454,#68455,#68456,#68457,#68458,#68459,
#68460,#68461,#68462,#68463,#68464,#68465,#68466,#68467,#68468,#68469,#68470,
#68471,#68472,#68473,#68474,#68475,#68476,#68477,#68478,#68479,#68480,#68481,
#68482,#68483,#68484,#68485,#68486,#68487,#68488,#68489,#68490,#68491,#68492,
#68493,#68494,#68495,#68496,#68497,#68498,#68499,#68500,#68501,#68502,#68503,
#68504,#68505,#68506,#68507,#68508,#68509,#68510,#68511,#68512,#68513,#68514,
#68515,#68516,#68517,#68518,#68519,#68520,#68521,#68522,#68523,#68524,#68525,
#68526,#68527,#68528,#68529,#68530,#68531,#68532,#68533,#68534,#68535,#68536,
#68537,#68538,#68539,#68540,#68541,#68542,#68543,#68544,#68545,#68546,#68547,
#68548,#68549,#68550,#68551,#68552,#68553,#68554,#68555,#68556,#68557,#68558,
#68559,#68560,#68561,#68562,#68563,#68564,#68565,#68566,#68567,#68568,#68569,
#68570,#68571,#68572,#68573,#68574,#68575,#68576,#68577,#68578,#68579,#68580,
#68581,#68582,#68583,#68584,#68585,#68586,#68587,#68588),.UNSPECIFIED.,
 .F.,.F.,(4,3,3,3,3,3,3,3,3,3,3,3,3,3,3,3,3,3,3,3,3,3,3,3,3,3,3,3,3,3,3,
3,3,3,3,3,3,3,3,3,3,3,3,3,3,3,3,3,3,3,3,3,3,3,3,3,3,3,3,3,3,3,3,3,3,3,3,
3,3,3,4),(-35.4716740690618,-35.3789228982328,-35.2862219687801,-35.1935448239753,
-35.1008650350535,-35.0080954319963,-34.9152817146125,-34.8223097482569,
-34.7366298026709,-34.6426399777574,-34.5487766481253,-34.4550115653746,
-34.3613130401666,-34.2676483747836,-34.173992187792,-34.08031911191,-33.9865458589465,
-33.8927176578865,-33.7987390101393,-33.7441546654517,-33.6501648405385,
-33.556301510907,-33.4625364281562,-33.3688379029486,-33.2751732375657,
-33.1815170505743,-33.0878439746921,-32.994070721729,-32.9002425206692,
-32.8062638729223,-32.7516795282326,-32.6576897033182,-32.5638263736856,
-32.4700612909339,-32.376362765725,-32.2826981003411,-32.1890419133485,
-32.0953688374656,-32.0015955845014,-31.9077673834402,-31.8137887356923,
-31.7592043910134,-31.6652145661003,-31.571351236469,-31.4775861537182,
-31.3838876285108,-31.290222963128,-31.1965667761368,-31.1028937002547,
-31.0091204472917,-30.915292246232,-30.8213135984851,-30.7667292537942,
-30.6727394288825,-30.5788760992527,-30.4851110165036,-30.3914124912977,
-30.2977478259166,-30.2040916389268,-30.110418563047,-30.0166453100855,
-29.9228171090273,-29.8288384612821,-29.7742541165751,-29.6786386681049,
-29.5831643289439,-29.4844954371785,-29.3892549266595,-29.294079326632,
-29.198949630498,-29.1884887618822),.UNSPECIFIED.);
#1470=B_SPLINE_CURVE_WITH_KNOTS('',3,(#68590,#68591,#68592,#68593,#68594,
#68595,#68596,#68597,#68598,#68599),.UNSPECIFIED.,.F.,.F.,(4,1,1,1,1,1,
1,4),(-29.1884825968197,-28.7817789793559,-27.7893038421367,-26.7968287049176,
-25.8043535676984,-24.8118784304792,-23.81940329326,-22.9053114674703),
 .UNSPECIFIED.);
#1471=B_SPLINE_CURVE_WITH_KNOTS('',3,(#68601,#68602,#68603,#68604,#68605,
#68606,#68607,#68608,#68609,#68610,#68611,#68612,#68613,#68614,#68615,#68616,
#68617,#68618,#68619,#68620,#68621,#68622,#68623,#68624,#68625,#68626,#68627,
#68628,#68629,#68630,#68631,#68632,#68633,#68634,#68635,#68636,#68637,#68638,
#68639,#68640,#68641,#68642,#68643,#68644,#68645,#68646,#68647,#68648,#68649,
#68650,#68651,#68652,#68653,#68654,#68655,#68656,#68657,#68658,#68659,#68660,
#68661,#68662,#68663,#68664,#68665,#68666,#68667,#68668,#68669,#68670,#68671,
#68672,#68673,#68674,#68675,#68676,#68677,#68678,#68679,#68680,#68681,#68682,
#68683,#68684,#68685,#68686,#68687,#68688,#68689,#68690,#68691,#68692,#68693,
#68694,#68695,#68696,#68697,#68698,#68699,#68700,#68701,#68702,#68703,#68704,
#68705,#68706,#68707,#68708,#68709,#68710,#68711,#68712,#68713,#68714,#68715,
#68716,#68717,#68718,#68719,#68720,#68721,#68722,#68723,#68724,#68725,#68726,
#68727,#68728,#68729,#68730,#68731,#68732,#68733,#68734,#68735,#68736,#68737,
#68738,#68739,#68740,#68741,#68742,#68743,#68744,#68745,#68746,#68747,#68748,
#68749,#68750,#68751,#68752,#68753,#68754,#68755,#68756,#68757,#68758,#68759,
#68760,#68761,#68762,#68763,#68764,#68765,#68766,#68767,#68768,#68769,#68770,
#68771,#68772,#68773,#68774,#68775,#68776,#68777,#68778,#68779,#68780,#68781,
#68782,#68783,#68784,#68785,#68786,#68787,#68788,#68789,#68790,#68791,#68792,
#68793,#68794,#68795,#68796,#68797,#68798,#68799,#68800,#68801,#68802,#68803,
#68804,#68805,#68806,#68807,#68808),.UNSPECIFIED.,.F.,.F.,(4,3,3,3,3,3,
3,3,3,3,3,3,3,3,3,3,3,3,3,3,3,3,3,3,3,3,3,3,3,3,3,3,3,3,3,3,3,3,3,3,3,3,
3,3,3,3,3,3,3,3,3,3,3,3,3,3,3,3,3,3,3,3,3,3,3,3,3,3,3,4),(-22.9053034547026,
-22.8269281560409,-22.732938331622,-22.6390750024836,-22.5453099202241,
-22.451611395503,-22.3579467306036,-22.2642905440919,-22.1706174686853,
-22.0768442161883,-21.9830160155899,-21.8890373682928,-21.8344530188217,
-21.7404631941409,-21.6465998647475,-21.5528347822404,-21.4591362572829,
-21.3654715921543,-21.2718154054209,-21.1781423298004,-21.0843690771022,
-20.9905408763096,-20.8965622288311,-20.8419778816025,-20.7479880542975,
-20.6541247222668,-20.5603596371129,-20.4666611095056,-20.3729964417263,
-20.2793402523445,-20.1856671740813,-20.0918939187651,-19.9980657153645,
-19.9040870653197,-19.8495027443834,-19.7555129236932,-19.661649598279,
-19.5678845197346,-19.4741859986994,-19.3805213374666,-19.2868651545979,
-19.1931920828063,-19.0994188338597,-19.0055906367805,-18.911611992919,
-18.8570276071642,-18.7630377823695,-18.6691744528973,-18.575409370346,
-18.4817108453957,-18.388046180306,-18.2943899936429,-18.2007169181238,
-18.1069436655733,-18.0131154649549,-17.9191368176901,-17.864552469945,
-17.7705626286161,-17.6766992825034,-17.5829341832289,-17.4892356415025,
-17.3955709596102,-17.3019147561389,-17.2082416638269,-17.1144683946094,
-17.0206401773705,-16.9266615137229,-16.8720773327259,-16.7470977402257,
-16.6221181477255),.UNSPECIFIED.);
#1472=B_SPLINE_CURVE_WITH_KNOTS('',3,(#68810,#68811,#68812,#68813,#68814,
#68815,#68816,#68817,#68818,#68819,#68820,#68821,#68822,#68823,#68824,#68825,
#68826,#68827,#68828,#68829,#68830,#68831,#68832,#68833,#68834,#68835,#68836,
#68837,#68838,#68839,#68840,#68841,#68842,#68843,#68844,#68845,#68846,#68847,
#68848,#68849,#68850,#68851,#68852,#68853,#68854,#68855,#68856,#68857,#68858,
#68859,#68860,#68861,#68862,#68863,#68864,#68865,#68866,#68867,#68868,#68869,
#68870,#68871,#68872,#68873,#68874,#68875,#68876,#68877,#68878,#68879,#68880,
#68881,#68882,#68883,#68884,#68885,#68886,#68887,#68888,#68889,#68890,#68891,
#68892,#68893,#68894,#68895,#68896,#68897,#68898,#68899,#68900,#68901,#68902,
#68903,#68904,#68905,#68906,#68907,#68908,#68909,#68910,#68911,#68912,#68913,
#68914,#68915,#68916,#68917,#68918,#68919,#68920,#68921,#68922,#68923,#68924,
#68925,#68926,#68927,#68928,#68929,#68930,#68931,#68932,#68933,#68934,#68935,
#68936,#68937,#68938,#68939,#68940,#68941,#68942,#68943,#68944,#68945,#68946,
#68947,#68948,#68949,#68950,#68951,#68952,#68953,#68954,#68955,#68956,#68957,
#68958,#68959,#68960,#68961,#68962,#68963,#68964,#68965,#68966,#68967,#68968,
#68969,#68970,#68971,#68972,#68973,#68974,#68975,#68976,#68977,#68978,#68979,
#68980,#68981,#68982,#68983,#68984,#68985,#68986,#68987,#68988,#68989,#68990,
#68991,#68992,#68993,#68994,#68995,#68996,#68997,#68998,#68999,#69000,#69001,
#69002,#69003,#69004,#69005,#69006,#69007,#69008,#69009,#69010,#69011,#69012,
#69013,#69014,#69015,#69016,#69017),.UNSPECIFIED.,.F.,.F.,(4,3,3,3,3,3,
3,3,3,3,3,3,3,3,3,3,3,3,3,3,3,3,3,3,3,3,3,3,3,3,3,3,3,3,3,3,3,3,3,3,3,3,
3,3,3,3,3,3,3,3,3,3,3,3,3,3,3,3,3,3,3,3,3,3,3,3,3,3,3,4),(-16.622118147523,
-16.529303653521,-16.4366606337733,-16.3440443155275,-16.2514282096388,
-16.1584717061058,-16.0657261490512,-15.972664172279,-15.8796021955067,
-15.7856123593066,-15.6917490186731,-15.5979839252156,-15.5042853897803,
-15.4106207144692,-15.3169645178588,-15.2232914326779,-15.1295181709556,
-15.0356899614281,-14.9417113057535,-14.8871270582875,-14.7931371249199,
-14.6992736862861,-14.6055084941381,-14.5118098593999,-14.418145084446,
-14.324488787978,-14.2308156028486,-14.1370422416525,-14.0432139327744,
-13.9492351789253,-13.8946519210684,-13.8006623712746,-13.7067993168445,
-13.6130345090102,-13.5193362571705,-13.4256718640968,-13.3320159480289,
-13.238343141357,-13.1445701533681,-13.0507422152792,-12.9567638247687,
-12.9021767838492,-12.8081867855782,-12.7143232845114,-12.6205580324466,
-12.526859341746,-12.433194513289,-12.3395381658261,-12.2458649322607,-12.1520915267901,
-12.0582631759197,-11.9642843840604,-11.90970164663,-11.8157111396676,-11.7218471235632,
-11.6280813508929,-11.5343821335191,-11.4407167748487,-11.3470598943064,
-11.2533861254682,-11.1596121846898,-11.0657832977134,-10.9718039738099,
-10.9172265094109,-10.8214033407368,-10.7257237751919,-10.6290260414798,
-10.5335869751275,-10.4362599077354,-10.3389328403434),.UNSPECIFIED.);
#1473=B_SPLINE_CURVE_WITH_KNOTS('',3,(#69018,#69019,#69020,#69021,#69022,
#69023,#69024,#69025,#69026,#69027,#69028,#69029,#69030,#69031,#69032,#69033,
#69034,#69035,#69036,#69037,#69038,#69039,#69040,#69041,#69042,#69043,#69044,
#69045,#69046,#69047,#69048,#69049,#69050,#69051,#69052,#69053,#69054,#69055,
#69056,#69057,#69058,#69059,#69060,#69061,#69062,#69063,#69064,#69065,#69066,
#69067,#69068,#69069,#69070,#69071,#69072,#69073,#69074,#69075,#69076,#69077,
#69078,#69079,#69080,#69081,#69082,#69083,#69084,#69085,#69086,#69087,#69088,
#69089,#69090,#69091,#69092,#69093,#69094,#69095,#69096,#69097,#69098,#69099,
#69100,#69101,#69102,#69103,#69104,#69105,#69106,#69107,#69108,#69109,#69110,
#69111,#69112,#69113,#69114,#69115,#69116,#69117,#69118,#69119,#69120,#69121,
#69122,#69123,#69124,#69125,#69126,#69127,#69128,#69129,#69130,#69131,#69132,
#69133,#69134,#69135,#69136,#69137,#69138,#69139,#69140,#69141,#69142,#69143,
#69144,#69145,#69146,#69147,#69148,#69149,#69150,#69151,#69152,#69153,#69154,
#69155,#69156,#69157,#69158,#69159,#69160,#69161,#69162,#69163,#69164,#69165,
#69166,#69167,#69168,#69169,#69170,#69171,#69172,#69173,#69174,#69175,#69176,
#69177,#69178,#69179,#69180,#69181,#69182,#69183,#69184,#69185,#69186,#69187,
#69188,#69189,#69190,#69191,#69192,#69193,#69194,#69195,#69196,#69197,#69198,
#69199,#69200,#69201,#69202,#69203,#69204,#69205,#69206,#69207,#69208,#69209,
#69210,#69211,#69212,#69213,#69214,#69215,#69216,#69217,#69218,#69219,#69220,
#69221,#69222,#69223,#69224,#69225),.UNSPECIFIED.,.F.,.F.,(4,3,3,3,3,3,
3,3,3,3,3,3,3,3,3,3,3,3,3,3,3,3,3,3,3,3,3,3,3,3,3,3,3,3,3,3,3,3,3,3,3,3,
3,3,3,3,3,3,3,3,3,3,3,3,3,3,3,3,3,3,3,3,3,3,3,3,3,3,3,4),(-10.3389328401642,
-10.2353874731711,-10.1327533663568,-10.0287523692743,-9.92475137219169,
-9.83075961919574,-9.73689437390884,-9.64312739029071,-9.54942699381244,
-9.45576047612084,-9.36210245792533,-9.26842757410462,-9.17465255940701,
-9.08082262010667,-8.98684228804526,-8.93227623497251,-8.83828241309624,
-8.74441505185367,-8.6506459087176,-8.55694329739515,-8.46327453159424,
-8.36961423501245,-8.2759370454921,-8.18215969796653,-8.0883274071486,-7.99434471765517,
-7.93980109775335,-7.84582719101489,-7.75197980594718,-7.65823067263216,
-7.56454803867557,-7.47089922267758,-7.37725882410477,-7.28360145651992,
-7.18984369474053,-7.09603088503644,-7.00206732014101,-6.94732596053418,
-6.85331736490599,-6.75943534045618,-6.66565166255936,-6.57193476554713,
-6.47825187314932,-6.38457762536547,-6.29088667648968,-6.19709594361215,
-6.10325045898227,-6.0092550055028,-5.95485082331501,-5.86084016495999,
-5.76695573758775,-5.6731693248544,-5.57944921521557,-5.48576281684318,
-5.39208477608375,-5.29838975334033,-5.2045945474717,-5.11074435826087,
-5.01674388507031,-4.96237568609584,-4.86955617493606,-4.77686249766569,
-4.68427218947732,-4.59173829152433,-4.49923418079547,-4.40673326888904,
-4.31415439096147,-4.22153603551285,-4.12877526983171,-4.05574753337591),
 .UNSPECIFIED.);
#1474=B_SPLINE_CURVE_WITH_KNOTS('',3,(#69228,#69229,#69230,#69231,#69232,
#69233,#69234,#69235,#69236,#69237,#69238,#69239,#69240,#69241,#69242,#69243,
#69244,#69245,#69246,#69247,#69248,#69249,#69250,#69251,#69252,#69253,#69254,
#69255,#69256,#69257,#69258,#69259,#69260,#69261,#69262,#69263,#69264,#69265,
#69266,#69267,#69268,#69269,#69270,#69271,#69272,#69273,#69274,#69275,#69276,
#69277,#69278,#69279,#69280,#69281,#69282,#69283,#69284,#69285,#69286,#69287,
#69288,#69289,#69290,#69291,#69292,#69293,#69294,#69295,#69296,#69297,#69298,
#69299,#69300,#69301,#69302,#69303,#69304,#69305,#69306,#69307,#69308,#69309,
#69310,#69311,#69312,#69313,#69314,#69315,#69316,#69317,#69318,#69319,#69320,
#69321,#69322,#69323,#69324,#69325,#69326,#69327,#69328,#69329,#69330,#69331,
#69332,#69333,#69334,#69335,#69336,#69337,#69338,#69339,#69340,#69341,#69342,
#69343,#69344,#69345,#69346,#69347,#69348,#69349,#69350,#69351,#69352,#69353,
#69354,#69355,#69356,#69357,#69358,#69359,#69360,#69361,#69362,#69363,#69364,
#69365,#69366,#69367,#69368,#69369,#69370,#69371,#69372,#69373,#69374,#69375,
#69376,#69377,#69378,#69379,#69380,#69381,#69382,#69383,#69384,#69385,#69386,
#69387,#69388,#69389,#69390,#69391,#69392,#69393,#69394,#69395,#69396,#69397,
#69398,#69399,#69400,#69401,#69402,#69403,#69404,#69405),.UNSPECIFIED.,
 .F.,.F.,(4,2,2,2,2,2,2,2,2,2,2,2,2,2,2,2,2,2,2,2,2,2,2,2,2,2,2,2,2,2,2,
2,2,2,2,2,2,2,2,2,2,2,2,2,2,2,2,2,2,2,2,2,2,2,2,2,2,2,2,2,2,2,2,2,2,2,2,
2,2,2,2,2,2,2,2,2,2,2,2,2,2,2,2,2,2,2,2,2,4),(-1.42845765518849,-1.42536520723414,
-1.4152106799514,-1.40000645349711,-1.36537780576554,-1.32846426919925,
-1.31882578618782,-1.31264347562592,-1.30673031714364,-1.29849799497411,
-1.27686787775135,-1.24046462295499,-1.20495917778271,-1.19723313512881,
-1.19330464947426,-1.19003138756434,-1.1856591932015,-1.17547759035392,
-1.16021971512157,-1.10340153745338,-1.08502637211127,-1.07781251877794,
-1.07189100828158,-1.06580425026859,-1.05666856388179,-1.02610026476917,
-0.997564570479381,-0.965304109106234,-0.95753238642215,-0.953590449435717,
-0.950306827488488,-0.945920862623889,-0.935712633518282,-0.920403351779626,
-0.885711427188332,-0.849406801774189,-0.839776414519515,-0.833582840866373,
-0.827646045497534,-0.819357871285679,-0.797406078607802,-0.761087574562804,
-0.725841905691213,-0.718105712749734,-0.71417271863651,-0.710913120996444,
-0.706578428912307,-0.696512562638217,-0.68147964072391,-0.620541456282429,
-0.604153436769905,-0.5967882038272,-0.591011115083337,-0.584584856189687,
-0.573644959721232,-0.534751712525508,-0.49107109487792,-0.479935020943087,
-0.475754502458658,-0.472432773967653,-0.468828132279145,-0.462698685853784,
-0.43064954985613,-0.374149053004026,-0.36295465566877,-0.355808816948442,
-0.350000995585055,-0.343211633245007,-0.330703313246897,-0.314581297100423,
-0.280498153286423,-0.245926707479042,-0.238162651384305,-0.234201926234243,
-0.231189491043961,-0.226862069247317,-0.217320989971945,-0.203451483169819,
-0.148879497062157,-0.129098959834247,-0.121687509624381,-0.11620466799479,
-0.110150587183573,-0.101518505191228,-0.0772017292500017,-0.0430984593012172,
-0.0101131422229349,-0.00412518396300005,-0.00334863135138759),
 .UNSPECIFIED.);
#1475=B_SPLINE_CURVE_WITH_KNOTS('',3,(#69409,#69410,#69411,#69412,#69413,
#69414,#69415,#69416,#69417,#69418,#69419,#69420,#69421,#69422,#69423,#69424,
#69425,#69426,#69427,#69428,#69429,#69430,#69431,#69432,#69433,#69434,#69435,
#69436,#69437,#69438,#69439,#69440,#69441,#69442,#69443,#69444,#69445,#69446,
#69447,#69448,#69449,#69450,#69451,#69452,#69453,#69454,#69455,#69456,#69457,
#69458,#69459,#69460,#69461,#69462,#69463,#69464,#69465,#69466,#69467,#69468,
#69469,#69470,#69471,#69472,#69473,#69474,#69475,#69476,#69477,#69478,#69479,
#69480,#69481,#69482,#69483,#69484,#69485,#69486,#69487,#69488,#69489,#69490,
#69491,#69492,#69493,#69494,#69495,#69496,#69497,#69498,#69499,#69500,#69501,
#69502,#69503,#69504,#69505,#69506,#69507,#69508,#69509,#69510,#69511,#69512,
#69513,#69514,#69515,#69516,#69517,#69518,#69519,#69520,#69521,#69522,#69523,
#69524,#69525,#69526,#69527,#69528,#69529,#69530,#69531,#69532,#69533,#69534,
#69535),.UNSPECIFIED.,.F.,.F.,(4,3,3,3,3,3,3,3,3,3,3,3,3,3,3,3,3,3,3,3,
3,3,3,3,3,3,3,3,3,3,3,3,3,3,3,3,3,3,3,3,3,3,4),(97.3893722615554,97.518875078662,
97.6483778957685,97.7487851448158,97.8490491164149,97.9491968996414,98.0492810170443,
98.1493320356798,98.2493804817632,98.3495236236437,98.4497127805419,98.5500755985478,
98.6408530329877,98.7411830318357,98.8413724125209,98.9414499030046,99.0414663731791,
99.1414524608134,99.2414387653865,99.3415245228427,99.4416588133798,99.5419715975158,
99.6333281702069,99.7325582456431,99.8316450817934,99.9309148599975,100.029830533657,
100.128718182013,100.227609766748,100.327158151918,100.42621669172,100.526009999573,
100.625803307426,100.728742075655,100.831518076764,100.934132454852,101.036651773703,
101.139101194609,101.24150579755,101.343920147708,101.446334638376,101.548821984608,
101.618278444645),.UNSPECIFIED.);
#1476=B_SPLINE_CURVE_WITH_KNOTS('',3,(#69536,#69537,#69538,#69539,#69540,
#69541,#69542,#69543,#69544,#69545,#69546,#69547,#69548,#69549,#69550,#69551,
#69552,#69553),.UNSPECIFIED.,.F.,.F.,(4,2,2,2,2,2,2,2,4),(-3.03489337710244,
-2.99899587031306,-2.99021794071613,-2.98407651260254,-2.97800987248344,
-2.97215058911282,-2.96506738697773,-2.94742697701634,-2.94523236784797),
 .UNSPECIFIED.);
#1477=B_SPLINE_CURVE_WITH_KNOTS('',3,(#69558,#69559,#69560,#69561,#69562,
#69563,#69564,#69565,#69566,#69567,#69568,#69569,#69570,#69571,#69572,#69573,
#69574,#69575,#69576,#69577,#69578,#69579,#69580,#69581,#69582,#69583,#69584,
#69585,#69586,#69587,#69588,#69589,#69590,#69591,#69592,#69593,#69594,#69595,
#69596,#69597,#69598,#69599,#69600,#69601,#69602,#69603,#69604,#69605,#69606,
#69607,#69608,#69609,#69610,#69611,#69612,#69613,#69614,#69615,#69616,#69617,
#69618,#69619,#69620,#69621,#69622,#69623,#69624,#69625,#69626,#69627,#69628,
#69629,#69630,#69631,#69632,#69633,#69634,#69635,#69636,#69637,#69638,#69639,
#69640,#69641,#69642,#69643,#69644,#69645,#69646,#69647,#69648,#69649,#69650,
#69651),.UNSPECIFIED.,.F.,.F.,(4,3,3,3,3,3,3,3,3,3,3,3,3,3,3,3,3,3,3,3,
3,3,3,3,3,3,3,3,3,3,3,4),(-0.554646516726398,-0.550740972514746,-0.520307837848763,
-0.493932175372676,-0.486045706929786,-0.47859141274925,-0.448508884890132,
-0.418681489211896,-0.414805187944416,-0.409823971499447,-0.3807253319587,
-0.351958298846651,-0.324015927788516,-0.30764879626434,-0.30203888514984,
-0.297878709519076,-0.270514541794969,-0.258756835329769,-0.230309513510376,
-0.201862191690984,-0.196335053501894,-0.19215012140112,-0.165081508204436,
-0.138209907372373,-0.111603956434757,-0.103486289378542,-0.0966196945845564,
-0.0926311917683891,-0.066934469307677,-0.0416411581672595,-0.0171026713579872,
0.),.UNSPECIFIED.);
#1478=B_SPLINE_CURVE_WITH_KNOTS('',3,(#69653,#69654,#69655,#69656),
 .UNSPECIFIED.,.F.,.F.,(4,4),(0.,0.0117666873624648),.UNSPECIFIED.);
#1479=B_SPLINE_CURVE_WITH_KNOTS('',3,(#69657,#69658,#69659,#69660,#69661,
#69662,#69663,#69664,#69665,#69666,#69667,#69668,#69669,#69670,#69671,#69672,
#69673,#69674,#69675,#69676,#69677,#69678,#69679,#69680,#69681,#69682,#69683,
#69684,#69685,#69686,#69687,#69688,#69689,#69690,#69691,#69692,#69693,#69694,
#69695,#69696,#69697,#69698,#69699,#69700,#69701,#69702,#69703,#69704,#69705,
#69706,#69707,#69708,#69709,#69710,#69711,#69712,#69713,#69714,#69715,#69716,
#69717,#69718,#69719,#69720,#69721,#69722,#69723,#69724,#69725,#69726,#69727,
#69728,#69729,#69730,#69731,#69732,#69733,#69734,#69735,#69736,#69737,#69738,
#69739,#69740,#69741,#69742,#69743,#69744),.UNSPECIFIED.,.F.,.F.,(4,3,3,
3,3,3,3,3,3,3,3,3,3,3,3,3,3,3,3,3,3,3,3,3,3,3,3,3,3,4),(-0.562645757026855,
-0.555701473914062,-0.530900441032168,-0.515098938149575,-0.507065541704813,
-0.499621376006763,-0.473611873388524,-0.45123192600063,-0.444269138995806,
-0.438512576095804,-0.411585781389386,-0.384071987787232,-0.356846623787638,
-0.339848296888339,-0.335818611590039,-0.30730117792828,-0.29482500179958,
-0.2670444715065,-0.23926394121342,-0.231611467000139,-0.227138760951209,
-0.198500238527404,-0.169355291582403,-0.139789787243429,-0.122176108873976,
-0.117677873121744,-0.0872368492236495,-0.0566234034005496,-0.0264688552303108,
0.),.UNSPECIFIED.);
#1480=B_SPLINE_CURVE_WITH_KNOTS('',3,(#70134,#70135,#70136,#70137),
 .UNSPECIFIED.,.F.,.F.,(4,4),(-0.0490568531851087,0.),.UNSPECIFIED.);
#1481=B_SPLINE_CURVE_WITH_KNOTS('',3,(#70138,#70139,#70140,#70141,#70142,
#70143,#70144,#70145,#70146,#70147,#70148,#70149,#70150,#70151,#70152,#70153,
#70154,#70155,#70156,#70157,#70158,#70159,#70160,#70161,#70162,#70163,#70164,
#70165,#70166,#70167,#70168,#70169,#70170,#70171,#70172,#70173,#70174,#70175,
#70176,#70177,#70178,#70179,#70180,#70181,#70182,#70183,#70184,#70185,#70186,
#70187,#70188,#70189,#70190,#70191,#70192,#70193,#70194,#70195,#70196,#70197,
#70198,#70199,#70200,#70201,#70202,#70203,#70204,#70205,#70206,#70207,#70208,
#70209,#70210,#70211,#70212,#70213,#70214,#70215,#70216,#70217,#70218,#70219,
#70220,#70221,#70222,#70223,#70224,#70225),.UNSPECIFIED.,.F.,.F.,(4,3,3,
3,3,3,3,3,3,3,3,3,3,3,3,3,3,3,3,3,3,3,3,3,3,3,3,3,3,4),(-0.56264575702688,
-0.555701473914083,-0.531007418756454,-0.515098938720501,-0.507065529682846,
-0.499621375158853,-0.473611844527599,-0.451231901960729,-0.44426920356528,
-0.438512593706661,-0.411476852815532,-0.384052718111971,-0.356621494830653,
-0.339848281411137,-0.335818576668947,-0.307301144235682,-0.294825001799607,
-0.267044458395629,-0.23926391499165,-0.231611325020553,-0.227138740775428,
-0.198500204394852,-0.169355239834281,-0.139789729029255,-0.122176056932312,
-0.117677830115777,-0.0872367918330862,-0.0566233467844078,-0.0264688402299216,
-1.07255465021213E-14),.UNSPECIFIED.);
#1482=B_SPLINE_CURVE_WITH_KNOTS('',3,(#70230,#70231,#70232,#70233,#70234,
#70235,#70236,#70237,#70238,#70239,#70240,#70241,#70242,#70243,#70244,#70245,
#70246,#70247,#70248,#70249,#70250,#70251,#70252,#70253,#70254,#70255,#70256,
#70257,#70258,#70259,#70260,#70261,#70262,#70263,#70264,#70265,#70266,#70267,
#70268,#70269,#70270,#70271,#70272,#70273,#70274,#70275,#70276,#70277,#70278,
#70279,#70280,#70281,#70282,#70283,#70284,#70285,#70286,#70287,#70288,#70289,
#70290,#70291,#70292,#70293,#70294,#70295,#70296,#70297,#70298,#70299,#70300,
#70301,#70302,#70303,#70304,#70305,#70306,#70307,#70308,#70309,#70310,#70311,
#70312,#70313,#70314,#70315,#70316,#70317,#70318,#70319,#70320),
 .UNSPECIFIED.,.F.,.F.,(4,3,3,3,3,3,3,3,3,3,3,3,3,3,3,3,3,3,3,3,3,3,3,3,
3,3,3,3,3,3,4),(-0.554646384615711,-0.550740972514731,-0.520102356322042,
-0.489576564448263,-0.481306012005539,-0.451226840594297,-0.427170533611444,
-0.414805205120169,-0.409823976078728,-0.380725346809426,-0.351958339265775,
-0.32401601607743,-0.307648859480877,-0.302038780735922,-0.297878690081443,
-0.270514560405435,-0.258756835329743,-0.23030952069742,-0.201862206065096,
-0.196335035864416,-0.192150115673263,-0.165068640371989,-0.138040782233652,
-0.11155197104457,-0.103486161100401,-0.0966193329184451,-0.092630885380201,
-0.0669341287282739,-0.0416407713559216,-0.0171022276675499,0.),
 .UNSPECIFIED.);
#1483=B_SPLINE_CURVE_WITH_KNOTS('',3,(#70710,#70711,#70712,#70713),
 .UNSPECIFIED.,.F.,.F.,(4,4),(-0.0490579837509845,0.),.UNSPECIFIED.);
#1563=FACE_BOUND('',#3276,.T.);
#1564=FACE_BOUND('',#3390,.T.);
#1902=PLANE('',#14631);
#1903=PLANE('',#14634);
#1904=PLANE('',#14640);
#1905=PLANE('',#14644);
#1906=PLANE('',#14645);
#1907=PLANE('',#14646);
#1908=PLANE('',#14647);
#1909=PLANE('',#14687);
#1910=PLANE('',#14688);
#1911=PLANE('',#14689);
#1912=PLANE('',#14691);
#1913=PLANE('',#14692);
#1914=PLANE('',#14693);
#1915=PLANE('',#14695);
#1916=PLANE('',#14696);
#1917=PLANE('',#14697);
#1918=PLANE('',#14699);
#1919=PLANE('',#14700);
#1920=PLANE('',#14701);
#1921=PLANE('',#14703);
#1922=PLANE('',#14704);
#1923=PLANE('',#14705);
#1924=PLANE('',#14707);
#1925=PLANE('',#14708);
#1926=PLANE('',#14709);
#1927=PLANE('',#14711);
#1928=PLANE('',#14712);
#1929=PLANE('',#14713);
#1930=PLANE('',#14715);
#1931=PLANE('',#14716);
#1932=PLANE('',#14717);
#1933=PLANE('',#14719);
#1934=PLANE('',#14720);
#1935=PLANE('',#14721);
#1936=PLANE('',#14723);
#1937=PLANE('',#14724);
#1938=PLANE('',#14725);
#1939=PLANE('',#14727);
#1940=PLANE('',#14728);
#1941=PLANE('',#14729);
#1942=PLANE('',#14731);
#1943=PLANE('',#14732);
#1944=PLANE('',#14733);
#1945=PLANE('',#14735);
#1946=PLANE('',#14736);
#1947=PLANE('',#14737);
#1948=PLANE('',#14739);
#1949=PLANE('',#14740);
#1950=PLANE('',#14741);
#1951=PLANE('',#14743);
#1952=PLANE('',#14744);
#1953=PLANE('',#14745);
#1954=PLANE('',#14747);
#1955=PLANE('',#14748);
#1956=PLANE('',#14749);
#1957=PLANE('',#14751);
#1958=PLANE('',#14752);
#1959=PLANE('',#14753);
#1960=PLANE('',#14756);
#1961=PLANE('',#14757);
#1962=PLANE('',#14758);
#1963=PLANE('',#14760);
#1964=PLANE('',#14761);
#1965=PLANE('',#14762);
#1966=PLANE('',#14764);
#1967=PLANE('',#14765);
#1968=PLANE('',#14766);
#1969=PLANE('',#14768);
#1970=PLANE('',#14769);
#1971=PLANE('',#14770);
#1972=PLANE('',#14772);
#1973=PLANE('',#14773);
#1974=PLANE('',#14774);
#1975=PLANE('',#14776);
#1976=PLANE('',#14777);
#1977=PLANE('',#14778);
#1978=PLANE('',#14780);
#1979=PLANE('',#14781);
#1980=PLANE('',#14782);
#1981=PLANE('',#14784);
#1982=PLANE('',#14785);
#1983=PLANE('',#14786);
#1984=PLANE('',#14788);
#1985=PLANE('',#14789);
#1986=PLANE('',#14790);
#1987=PLANE('',#14792);
#1988=PLANE('',#14793);
#1989=PLANE('',#14794);
#1990=PLANE('',#14796);
#1991=PLANE('',#14797);
#1992=PLANE('',#14798);
#1993=PLANE('',#14800);
#1994=PLANE('',#14801);
#1995=PLANE('',#14802);
#1996=PLANE('',#14804);
#1997=PLANE('',#14805);
#1998=PLANE('',#14806);
#1999=PLANE('',#14808);
#2000=PLANE('',#14809);
#2001=PLANE('',#14810);
#2002=PLANE('',#14812);
#2003=PLANE('',#14813);
#2004=PLANE('',#14814);
#2005=PLANE('',#14816);
#2006=PLANE('',#14817);
#2007=PLANE('',#14818);
#2008=PLANE('',#14820);
#2009=PLANE('',#14821);
#2010=PLANE('',#14822);
#2011=PLANE('',#14824);
#2012=PLANE('',#14825);
#2013=PLANE('',#14826);
#2014=PLANE('',#14829);
#2015=PLANE('',#14830);
#2016=PLANE('',#14832);
#2017=PLANE('',#14834);
#2018=PLANE('',#14836);
#2019=PLANE('',#14838);
#2020=PLANE('',#14840);
#2021=PLANE('',#14843);
#2022=PLANE('',#14844);
#2023=PLANE('',#14845);
#2024=PLANE('',#14846);
#2025=PLANE('',#14847);
#2026=PLANE('',#14848);
#2527=FACE_OUTER_BOUND('',#3254,.T.);
#2528=FACE_OUTER_BOUND('',#3255,.T.);
#2529=FACE_OUTER_BOUND('',#3256,.T.);
#2530=FACE_OUTER_BOUND('',#3257,.T.);
#2531=FACE_OUTER_BOUND('',#3258,.T.);
#2532=FACE_OUTER_BOUND('',#3259,.T.);
#2533=FACE_OUTER_BOUND('',#3260,.T.);
#2534=FACE_OUTER_BOUND('',#3261,.T.);
#2535=FACE_OUTER_BOUND('',#3262,.T.);
#2536=FACE_OUTER_BOUND('',#3263,.T.);
#2537=FACE_OUTER_BOUND('',#3264,.T.);
#2538=FACE_OUTER_BOUND('',#3265,.T.);
#2539=FACE_OUTER_BOUND('',#3266,.T.);
#2540=FACE_OUTER_BOUND('',#3267,.T.);
#2541=FACE_OUTER_BOUND('',#3268,.T.);
#2542=FACE_OUTER_BOUND('',#3269,.T.);
#2543=FACE_OUTER_BOUND('',#3270,.T.);
#2544=FACE_OUTER_BOUND('',#3271,.T.);
#2545=FACE_OUTER_BOUND('',#3272,.T.);
#2546=FACE_OUTER_BOUND('',#3273,.T.);
#2547=FACE_OUTER_BOUND('',#3274,.T.);
#2548=FACE_OUTER_BOUND('',#3275,.T.);
#2549=FACE_OUTER_BOUND('',#3277,.T.);
#2550=FACE_OUTER_BOUND('',#3278,.T.);
#2551=FACE_OUTER_BOUND('',#3279,.T.);
#2552=FACE_OUTER_BOUND('',#3280,.T.);
#2553=FACE_OUTER_BOUND('',#3281,.T.);
#2554=FACE_OUTER_BOUND('',#3282,.T.);
#2555=FACE_OUTER_BOUND('',#3283,.T.);
#2556=FACE_OUTER_BOUND('',#3284,.T.);
#2557=FACE_OUTER_BOUND('',#3285,.T.);
#2558=FACE_OUTER_BOUND('',#3286,.T.);
#2559=FACE_OUTER_BOUND('',#3287,.T.);
#2560=FACE_OUTER_BOUND('',#3288,.T.);
#2561=FACE_OUTER_BOUND('',#3289,.T.);
#2562=FACE_OUTER_BOUND('',#3290,.T.);
#2563=FACE_OUTER_BOUND('',#3291,.T.);
#2564=FACE_OUTER_BOUND('',#3292,.T.);
#2565=FACE_OUTER_BOUND('',#3293,.T.);
#2566=FACE_OUTER_BOUND('',#3294,.T.);
#2567=FACE_OUTER_BOUND('',#3295,.T.);
#2568=FACE_OUTER_BOUND('',#3296,.T.);
#2569=FACE_OUTER_BOUND('',#3297,.T.);
#2570=FACE_OUTER_BOUND('',#3298,.T.);
#2571=FACE_OUTER_BOUND('',#3299,.T.);
#2572=FACE_OUTER_BOUND('',#3300,.T.);
#2573=FACE_OUTER_BOUND('',#3301,.T.);
#2574=FACE_OUTER_BOUND('',#3302,.T.);
#2575=FACE_OUTER_BOUND('',#3303,.T.);
#2576=FACE_OUTER_BOUND('',#3304,.T.);
#2577=FACE_OUTER_BOUND('',#3305,.T.);
#2578=FACE_OUTER_BOUND('',#3306,.T.);
#2579=FACE_OUTER_BOUND('',#3307,.T.);
#2580=FACE_OUTER_BOUND('',#3308,.T.);
#2581=FACE_OUTER_BOUND('',#3309,.T.);
#2582=FACE_OUTER_BOUND('',#3310,.T.);
#2583=FACE_OUTER_BOUND('',#3311,.T.);
#2584=FACE_OUTER_BOUND('',#3312,.T.);
#2585=FACE_OUTER_BOUND('',#3313,.T.);
#2586=FACE_OUTER_BOUND('',#3314,.T.);
#2587=FACE_OUTER_BOUND('',#3315,.T.);
#2588=FACE_OUTER_BOUND('',#3316,.T.);
#2589=FACE_OUTER_BOUND('',#3317,.T.);
#2590=FACE_OUTER_BOUND('',#3318,.T.);
#2591=FACE_OUTER_BOUND('',#3319,.T.);
#2592=FACE_OUTER_BOUND('',#3320,.T.);
#2593=FACE_OUTER_BOUND('',#3321,.T.);
#2594=FACE_OUTER_BOUND('',#3322,.T.);
#2595=FACE_OUTER_BOUND('',#3323,.T.);
#2596=FACE_OUTER_BOUND('',#3324,.T.);
#2597=FACE_OUTER_BOUND('',#3325,.T.);
#2598=FACE_OUTER_BOUND('',#3326,.T.);
#2599=FACE_OUTER_BOUND('',#3327,.T.);
#2600=FACE_OUTER_BOUND('',#3328,.T.);
#2601=FACE_OUTER_BOUND('',#3329,.T.);
#2602=FACE_OUTER_BOUND('',#3330,.T.);
#2603=FACE_OUTER_BOUND('',#3331,.T.);
#2604=FACE_OUTER_BOUND('',#3332,.T.);
#2605=FACE_OUTER_BOUND('',#3333,.T.);
#2606=FACE_OUTER_BOUND('',#3334,.T.);
#2607=FACE_OUTER_BOUND('',#3335,.T.);
#2608=FACE_OUTER_BOUND('',#3336,.T.);
#2609=FACE_OUTER_BOUND('',#3337,.T.);
#2610=FACE_OUTER_BOUND('',#3338,.T.);
#2611=FACE_OUTER_BOUND('',#3339,.T.);
#2612=FACE_OUTER_BOUND('',#3340,.T.);
#2613=FACE_OUTER_BOUND('',#3341,.T.);
#2614=FACE_OUTER_BOUND('',#3342,.T.);
#2615=FACE_OUTER_BOUND('',#3343,.T.);
#2616=FACE_OUTER_BOUND('',#3344,.T.);
#2617=FACE_OUTER_BOUND('',#3345,.T.);
#2618=FACE_OUTER_BOUND('',#3346,.T.);
#2619=FACE_OUTER_BOUND('',#3347,.T.);
#2620=FACE_OUTER_BOUND('',#3348,.T.);
#2621=FACE_OUTER_BOUND('',#3349,.T.);
#2622=FACE_OUTER_BOUND('',#3350,.T.);
#2623=FACE_OUTER_BOUND('',#3351,.T.);
#2624=FACE_OUTER_BOUND('',#3352,.T.);
#2625=FACE_OUTER_BOUND('',#3353,.T.);
#2626=FACE_OUTER_BOUND('',#3354,.T.);
#2627=FACE_OUTER_BOUND('',#3355,.T.);
#2628=FACE_OUTER_BOUND('',#3356,.T.);
#2629=FACE_OUTER_BOUND('',#3357,.T.);
#2630=FACE_OUTER_BOUND('',#3358,.T.);
#2631=FACE_OUTER_BOUND('',#3359,.T.);
#2632=FACE_OUTER_BOUND('',#3360,.T.);
#2633=FACE_OUTER_BOUND('',#3361,.T.);
#2634=FACE_OUTER_BOUND('',#3362,.T.);
#2635=FACE_OUTER_BOUND('',#3363,.T.);
#2636=FACE_OUTER_BOUND('',#3364,.T.);
#2637=FACE_OUTER_BOUND('',#3365,.T.);
#2638=FACE_OUTER_BOUND('',#3366,.T.);
#2639=FACE_OUTER_BOUND('',#3367,.T.);
#2640=FACE_OUTER_BOUND('',#3368,.T.);
#2641=FACE_OUTER_BOUND('',#3369,.T.);
#2642=FACE_OUTER_BOUND('',#3370,.T.);
#2643=FACE_OUTER_BOUND('',#3371,.T.);
#2644=FACE_OUTER_BOUND('',#3372,.T.);
#2645=FACE_OUTER_BOUND('',#3373,.T.);
#2646=FACE_OUTER_BOUND('',#3374,.T.);
#2647=FACE_OUTER_BOUND('',#3375,.T.);
#2648=FACE_OUTER_BOUND('',#3376,.T.);
#2649=FACE_OUTER_BOUND('',#3377,.T.);
#2650=FACE_OUTER_BOUND('',#3378,.T.);
#2651=FACE_OUTER_BOUND('',#3379,.T.);
#2652=FACE_OUTER_BOUND('',#3380,.T.);
#2653=FACE_OUTER_BOUND('',#3381,.T.);
#2654=FACE_OUTER_BOUND('',#3382,.T.);
#2655=FACE_OUTER_BOUND('',#3383,.T.);
#2656=FACE_OUTER_BOUND('',#3384,.T.);
#2657=FACE_OUTER_BOUND('',#3385,.T.);
#2658=FACE_OUTER_BOUND('',#3386,.T.);
#2659=FACE_OUTER_BOUND('',#3387,.T.);
#2660=FACE_OUTER_BOUND('',#3388,.T.);
#2661=FACE_OUTER_BOUND('',#3389,.T.);
#2662=FACE_OUTER_BOUND('',#3391,.T.);
#2663=FACE_OUTER_BOUND('',#3392,.T.);
#2664=FACE_OUTER_BOUND('',#3393,.T.);
#2665=FACE_OUTER_BOUND('',#3394,.T.);
#2666=FACE_OUTER_BOUND('',#3395,.T.);
#2667=FACE_OUTER_BOUND('',#3396,.T.);
#2668=FACE_OUTER_BOUND('',#3397,.T.);
#2669=FACE_OUTER_BOUND('',#3398,.T.);
#2670=FACE_OUTER_BOUND('',#3399,.T.);
#2671=FACE_OUTER_BOUND('',#3400,.T.);
#2672=FACE_OUTER_BOUND('',#3401,.T.);
#2673=FACE_OUTER_BOUND('',#3402,.T.);
#2674=FACE_OUTER_BOUND('',#3403,.T.);
#3254=EDGE_LOOP('',(#11931,#11932,#11933,#11934));
#3255=EDGE_LOOP('',(#11935,#11936,#11937,#11938,#11939,#11940));
#3256=EDGE_LOOP('',(#11941,#11942,#11943,#11944,#11945));
#3257=EDGE_LOOP('',(#11946,#11947,#11948,#11949,#11950,#11951));
#3258=EDGE_LOOP('',(#11952,#11953,#11954,#11955,#11956));
#3259=EDGE_LOOP('',(#11957,#11958,#11959,#11960,#11961));
#3260=EDGE_LOOP('',(#11962,#11963,#11964,#11965,#11966));
#3261=EDGE_LOOP('',(#11967,#11968,#11969,#11970,#11971));
#3262=EDGE_LOOP('',(#11972,#11973,#11974,#11975,#11976));
#3263=EDGE_LOOP('',(#11977,#11978,#11979,#11980,#11981));
#3264=EDGE_LOOP('',(#11982,#11983,#11984,#11985,#11986,#11987));
#3265=EDGE_LOOP('',(#11988,#11989,#11990,#11991,#11992));
#3266=EDGE_LOOP('',(#11993,#11994,#11995,#11996,#11997));
#3267=EDGE_LOOP('',(#11998,#11999,#12000,#12001));
#3268=EDGE_LOOP('',(#12002,#12003,#12004,#12005,#12006,#12007,#12008,#12009,
#12010,#12011,#12012,#12013,#12014,#12015,#12016,#12017,#12018,#12019,#12020,
#12021,#12022,#12023,#12024,#12025,#12026,#12027,#12028,#12029,#12030,#12031,
#12032,#12033,#12034,#12035));
#3269=EDGE_LOOP('',(#12036,#12037,#12038,#12039,#12040));
#3270=EDGE_LOOP('',(#12041,#12042,#12043,#12044,#12045,#12046));
#3271=EDGE_LOOP('',(#12047,#12048,#12049,#12050,#12051,#12052,#12053,#12054,
#12055,#12056,#12057,#12058,#12059,#12060,#12061,#12062,#12063,#12064,#12065,
#12066,#12067,#12068,#12069,#12070,#12071,#12072,#12073,#12074,#12075,#12076,
#12077,#12078,#12079,#12080,#12081,#12082,#12083,#12084,#12085,#12086,#12087,
#12088,#12089));
#3272=EDGE_LOOP('',(#12090,#12091,#12092,#12093,#12094));
#3273=EDGE_LOOP('',(#12095,#12096,#12097,#12098,#12099,#12100,#12101,#12102,
#12103,#12104,#12105,#12106,#12107,#12108,#12109,#12110,#12111,#12112,#12113,
#12114,#12115,#12116,#12117,#12118,#12119,#12120,#12121,#12122,#12123,#12124,
#12125,#12126,#12127,#12128,#12129,#12130,#12131,#12132,#12133,#12134,#12135,
#12136));
#3274=EDGE_LOOP('',(#12137,#12138,#12139,#12140,#12141,#12142,#12143));
#3275=EDGE_LOOP('',(#12144));
#3276=EDGE_LOOP('',(#12145));
#3277=EDGE_LOOP('',(#12146,#12147,#12148,#12149,#12150,#12151,#12152));
#3278=EDGE_LOOP('',(#12153));
#3279=EDGE_LOOP('',(#12154,#12155,#12156,#12157));
#3280=EDGE_LOOP('',(#12158,#12159,#12160,#12161));
#3281=EDGE_LOOP('',(#12162,#12163,#12164));
#3282=EDGE_LOOP('',(#12165,#12166,#12167,#12168,#12169,#12170,#12171,#12172,
#12173,#12174,#12175,#12176,#12177,#12178,#12179,#12180,#12181,#12182,#12183,
#12184,#12185,#12186,#12187,#12188,#12189,#12190,#12191,#12192,#12193,#12194,
#12195,#12196,#12197,#12198,#12199,#12200,#12201,#12202,#12203,#12204,#12205,
#12206,#12207,#12208,#12209,#12210,#12211,#12212,#12213,#12214,#12215,#12216,
#12217,#12218,#12219,#12220,#12221,#12222,#12223,#12224,#12225,#12226,#12227,
#12228,#12229,#12230,#12231,#12232,#12233,#12234,#12235,#12236,#12237,#12238,
#12239,#12240,#12241,#12242,#12243,#12244,#12245,#12246,#12247,#12248,#12249,
#12250,#12251,#12252,#12253,#12254,#12255,#12256,#12257,#12258,#12259,#12260,
#12261,#12262,#12263,#12264,#12265,#12266,#12267,#12268,#12269,#12270,#12271,
#12272,#12273,#12274,#12275));
#3283=EDGE_LOOP('',(#12276,#12277,#12278,#12279));
#3284=EDGE_LOOP('',(#12280,#12281,#12282,#12283));
#3285=EDGE_LOOP('',(#12284,#12285,#12286));
#3286=EDGE_LOOP('',(#12287,#12288,#12289,#12290));
#3287=EDGE_LOOP('',(#12291,#12292,#12293,#12294));
#3288=EDGE_LOOP('',(#12295,#12296,#12297));
#3289=EDGE_LOOP('',(#12298,#12299,#12300,#12301));
#3290=EDGE_LOOP('',(#12302,#12303,#12304,#12305));
#3291=EDGE_LOOP('',(#12306,#12307,#12308));
#3292=EDGE_LOOP('',(#12309,#12310,#12311,#12312));
#3293=EDGE_LOOP('',(#12313,#12314,#12315,#12316));
#3294=EDGE_LOOP('',(#12317,#12318,#12319));
#3295=EDGE_LOOP('',(#12320,#12321,#12322,#12323));
#3296=EDGE_LOOP('',(#12324,#12325,#12326,#12327));
#3297=EDGE_LOOP('',(#12328,#12329,#12330));
#3298=EDGE_LOOP('',(#12331,#12332,#12333,#12334));
#3299=EDGE_LOOP('',(#12335,#12336,#12337,#12338));
#3300=EDGE_LOOP('',(#12339,#12340,#12341));
#3301=EDGE_LOOP('',(#12342,#12343,#12344,#12345));
#3302=EDGE_LOOP('',(#12346,#12347,#12348,#12349));
#3303=EDGE_LOOP('',(#12350,#12351,#12352));
#3304=EDGE_LOOP('',(#12353,#12354,#12355,#12356));
#3305=EDGE_LOOP('',(#12357,#12358,#12359,#12360));
#3306=EDGE_LOOP('',(#12361,#12362,#12363));
#3307=EDGE_LOOP('',(#12364,#12365,#12366,#12367));
#3308=EDGE_LOOP('',(#12368,#12369,#12370,#12371));
#3309=EDGE_LOOP('',(#12372,#12373,#12374));
#3310=EDGE_LOOP('',(#12375,#12376,#12377,#12378));
#3311=EDGE_LOOP('',(#12379,#12380,#12381,#12382));
#3312=EDGE_LOOP('',(#12383,#12384,#12385));
#3313=EDGE_LOOP('',(#12386,#12387,#12388,#12389));
#3314=EDGE_LOOP('',(#12390,#12391,#12392,#12393));
#3315=EDGE_LOOP('',(#12394,#12395,#12396));
#3316=EDGE_LOOP('',(#12397,#12398,#12399,#12400));
#3317=EDGE_LOOP('',(#12401,#12402,#12403,#12404));
#3318=EDGE_LOOP('',(#12405,#12406,#12407));
#3319=EDGE_LOOP('',(#12408,#12409,#12410,#12411));
#3320=EDGE_LOOP('',(#12412,#12413,#12414,#12415));
#3321=EDGE_LOOP('',(#12416,#12417,#12418));
#3322=EDGE_LOOP('',(#12419,#12420,#12421,#12422));
#3323=EDGE_LOOP('',(#12423,#12424,#12425,#12426));
#3324=EDGE_LOOP('',(#12427,#12428,#12429));
#3325=EDGE_LOOP('',(#12430,#12431,#12432,#12433));
#3326=EDGE_LOOP('',(#12434,#12435,#12436,#12437));
#3327=EDGE_LOOP('',(#12438,#12439,#12440));
#3328=EDGE_LOOP('',(#12441,#12442,#12443,#12444));
#3329=EDGE_LOOP('',(#12445,#12446,#12447,#12448));
#3330=EDGE_LOOP('',(#12449,#12450,#12451));
#3331=EDGE_LOOP('',(#12452,#12453,#12454,#12455));
#3332=EDGE_LOOP('',(#12456,#12457,#12458,#12459));
#3333=EDGE_LOOP('',(#12460,#12461,#12462,#12463));
#3334=EDGE_LOOP('',(#12464,#12465,#12466,#12467));
#3335=EDGE_LOOP('',(#12468,#12469,#12470,#12471));
#3336=EDGE_LOOP('',(#12472,#12473,#12474));
#3337=EDGE_LOOP('',(#12475,#12476,#12477,#12478));
#3338=EDGE_LOOP('',(#12479,#12480,#12481,#12482));
#3339=EDGE_LOOP('',(#12483,#12484,#12485));
#3340=EDGE_LOOP('',(#12486,#12487,#12488,#12489));
#3341=EDGE_LOOP('',(#12490,#12491,#12492,#12493));
#3342=EDGE_LOOP('',(#12494,#12495,#12496));
#3343=EDGE_LOOP('',(#12497,#12498,#12499,#12500));
#3344=EDGE_LOOP('',(#12501,#12502,#12503,#12504));
#3345=EDGE_LOOP('',(#12505,#12506,#12507));
#3346=EDGE_LOOP('',(#12508,#12509,#12510,#12511));
#3347=EDGE_LOOP('',(#12512,#12513,#12514,#12515));
#3348=EDGE_LOOP('',(#12516,#12517,#12518));
#3349=EDGE_LOOP('',(#12519,#12520,#12521,#12522));
#3350=EDGE_LOOP('',(#12523,#12524,#12525,#12526));
#3351=EDGE_LOOP('',(#12527,#12528,#12529));
#3352=EDGE_LOOP('',(#12530,#12531,#12532,#12533));
#3353=EDGE_LOOP('',(#12534,#12535,#12536,#12537));
#3354=EDGE_LOOP('',(#12538,#12539,#12540));
#3355=EDGE_LOOP('',(#12541,#12542,#12543,#12544));
#3356=EDGE_LOOP('',(#12545,#12546,#12547,#12548));
#3357=EDGE_LOOP('',(#12549,#12550,#12551));
#3358=EDGE_LOOP('',(#12552,#12553,#12554,#12555));
#3359=EDGE_LOOP('',(#12556,#12557,#12558,#12559));
#3360=EDGE_LOOP('',(#12560,#12561,#12562));
#3361=EDGE_LOOP('',(#12563,#12564,#12565,#12566));
#3362=EDGE_LOOP('',(#12567,#12568,#12569,#12570));
#3363=EDGE_LOOP('',(#12571,#12572,#12573));
#3364=EDGE_LOOP('',(#12574,#12575,#12576,#12577));
#3365=EDGE_LOOP('',(#12578,#12579,#12580,#12581));
#3366=EDGE_LOOP('',(#12582,#12583,#12584));
#3367=EDGE_LOOP('',(#12585,#12586,#12587,#12588));
#3368=EDGE_LOOP('',(#12589,#12590,#12591,#12592));
#3369=EDGE_LOOP('',(#12593,#12594,#12595));
#3370=EDGE_LOOP('',(#12596,#12597,#12598,#12599));
#3371=EDGE_LOOP('',(#12600,#12601,#12602,#12603));
#3372=EDGE_LOOP('',(#12604,#12605,#12606));
#3373=EDGE_LOOP('',(#12607,#12608,#12609,#12610));
#3374=EDGE_LOOP('',(#12611,#12612,#12613,#12614));
#3375=EDGE_LOOP('',(#12615,#12616,#12617));
#3376=EDGE_LOOP('',(#12618,#12619,#12620,#12621));
#3377=EDGE_LOOP('',(#12622,#12623,#12624,#12625));
#3378=EDGE_LOOP('',(#12626,#12627,#12628));
#3379=EDGE_LOOP('',(#12629,#12630,#12631,#12632));
#3380=EDGE_LOOP('',(#12633,#12634,#12635,#12636));
#3381=EDGE_LOOP('',(#12637,#12638,#12639));
#3382=EDGE_LOOP('',(#12640,#12641,#12642,#12643));
#3383=EDGE_LOOP('',(#12644,#12645,#12646,#12647));
#3384=EDGE_LOOP('',(#12648,#12649,#12650));
#3385=EDGE_LOOP('',(#12651,#12652,#12653,#12654));
#3386=EDGE_LOOP('',(#12655,#12656,#12657,#12658));
#3387=EDGE_LOOP('',(#12659,#12660,#12661));
#3388=EDGE_LOOP('',(#12662,#12663,#12664,#12665,#12666,#12667,#12668,#12669,
#12670,#12671,#12672,#12673,#12674,#12675,#12676,#12677,#12678,#12679,#12680,
#12681,#12682,#12683,#12684,#12685,#12686,#12687,#12688,#12689,#12690,#12691,
#12692,#12693,#12694,#12695,#12696,#12697,#12698,#12699,#12700,#12701,#12702,
#12703,#12704,#12705,#12706,#12707,#12708,#12709,#12710,#12711,#12712,#12713,
#12714,#12715,#12716,#12717,#12718,#12719,#12720,#12721,#12722,#12723,#12724,
#12725,#12726,#12727,#12728,#12729,#12730,#12731,#12732,#12733,#12734,#12735,
#12736,#12737,#12738,#12739,#12740,#12741,#12742,#12743,#12744,#12745,#12746,
#12747,#12748,#12749,#12750,#12751,#12752,#12753,#12754,#12755,#12756,#12757,
#12758,#12759,#12760,#12761,#12762,#12763,#12764,#12765,#12766,#12767,#12768,
#12769,#12770,#12771,#12772,#12773,#12774,#12775,#12776,#12777,#12778,#12779,
#12780,#12781,#12782,#12783,#12784,#12785,#12786,#12787,#12788,#12789,#12790,
#12791,#12792,#12793,#12794,#12795,#12796,#12797,#12798,#12799,#12800,#12801,
#12802,#12803,#12804,#12805,#12806,#12807,#12808,#12809));
#3389=EDGE_LOOP('',(#12810));
#3390=EDGE_LOOP('',(#12811,#12812,#12813,#12814,#12815,#12816));
#3391=EDGE_LOOP('',(#12817,#12818));
#3392=EDGE_LOOP('',(#12819,#12820));
#3393=EDGE_LOOP('',(#12821,#12822));
#3394=EDGE_LOOP('',(#12823,#12824));
#3395=EDGE_LOOP('',(#12825,#12826));
#3396=EDGE_LOOP('',(#12827,#12828));
#3397=EDGE_LOOP('',(#12829,#12830,#12831,#12832,#12833,#12834,#12835,#12836));
#3398=EDGE_LOOP('',(#12837,#12838,#12839,#12840));
#3399=EDGE_LOOP('',(#12841,#12842,#12843,#12844));
#3400=EDGE_LOOP('',(#12845,#12846,#12847,#12848));
#3401=EDGE_LOOP('',(#12849,#12850,#12851,#12852));
#3402=EDGE_LOOP('',(#12853,#12854,#12855,#12856));
#3403=EDGE_LOOP('',(#12857,#12858,#12859,#12860));
#3746=CIRCLE('',#14612,2.40538);
#3747=CIRCLE('',#14627,3.11023);
#3748=CIRCLE('',#14628,3.11023);
#3749=CIRCLE('',#14630,2.40538);
#3750=CIRCLE('',#14632,3.11023);
#3751=CIRCLE('',#14633,3.11023);
#3752=CIRCLE('',#14635,3.11023);
#3753=CIRCLE('',#14636,3.11023);
#3754=CIRCLE('',#14638,3.31023);
#3755=CIRCLE('',#14639,0.2);
#3756=CIRCLE('',#14641,4.7625);
#3757=CIRCLE('',#14643,2.71023);
#3758=CIRCLE('',#14648,4.7625);
#3759=CIRCLE('',#14650,4.7625);
#3760=CIRCLE('',#14651,4.7625);
#3761=CIRCLE('',#14652,4.7625);
#3762=CIRCLE('',#14653,4.7625);
#3763=CIRCLE('',#14654,4.7625);
#3764=CIRCLE('',#14655,4.7625);
#3765=CIRCLE('',#14656,4.7625);
#3766=CIRCLE('',#14657,4.7625);
#3767=CIRCLE('',#14658,4.7625);
#3768=CIRCLE('',#14659,4.7625);
#3769=CIRCLE('',#14660,4.7625);
#3770=CIRCLE('',#14661,4.7625);
#3771=CIRCLE('',#14662,4.7625);
#3772=CIRCLE('',#14663,4.7625);
#3773=CIRCLE('',#14664,4.7625);
#3774=CIRCLE('',#14665,4.7625);
#3775=CIRCLE('',#14666,4.7625);
#3776=CIRCLE('',#14667,4.7625);
#3777=CIRCLE('',#14668,4.7625);
#3778=CIRCLE('',#14669,4.7625);
#3779=CIRCLE('',#14670,4.7625);
#3780=CIRCLE('',#14671,4.7625);
#3781=CIRCLE('',#14672,4.7625);
#3782=CIRCLE('',#14673,4.7625);
#3783=CIRCLE('',#14674,4.7625);
#3784=CIRCLE('',#14675,4.7625);
#3785=CIRCLE('',#14676,4.7625);
#3786=CIRCLE('',#14677,4.7625);
#3787=CIRCLE('',#14678,4.7625);
#3788=CIRCLE('',#14679,4.7625);
#3789=CIRCLE('',#14680,4.7625);
#3790=CIRCLE('',#14681,4.7625);
#3791=CIRCLE('',#14682,4.7625);
#3792=CIRCLE('',#14683,4.7625);
#3793=CIRCLE('',#14684,4.7625);
#3794=CIRCLE('',#14685,4.7625);
#3795=CIRCLE('',#14686,4.3625);
#3796=CIRCLE('',#14690,4.7625);
#3797=CIRCLE('',#14694,4.7625);
#3798=CIRCLE('',#14698,4.7625);
#3799=CIRCLE('',#14702,4.7625);
#3800=CIRCLE('',#14706,4.7625);
#3801=CIRCLE('',#14710,4.7625);
#3802=CIRCLE('',#14714,4.7625);
#3803=CIRCLE('',#14718,4.7625);
#3804=CIRCLE('',#14722,4.7625);
#3805=CIRCLE('',#14726,4.7625);
#3806=CIRCLE('',#14730,4.7625);
#3807=CIRCLE('',#14734,4.7625);
#3808=CIRCLE('',#14738,4.7625);
#3809=CIRCLE('',#14742,4.7625);
#3810=CIRCLE('',#14746,4.7625);
#3811=CIRCLE('',#14750,4.7625);
#3812=CIRCLE('',#14754,4.7625);
#3813=CIRCLE('',#14755,4.7625);
#3814=CIRCLE('',#14759,4.7625);
#3815=CIRCLE('',#14763,4.7625);
#3816=CIRCLE('',#14767,4.7625);
#3817=CIRCLE('',#14771,4.7625);
#3818=CIRCLE('',#14775,4.7625);
#3819=CIRCLE('',#14779,4.7625);
#3820=CIRCLE('',#14783,4.7625);
#3821=CIRCLE('',#14787,4.7625);
#3822=CIRCLE('',#14791,4.7625);
#3823=CIRCLE('',#14795,4.7625);
#3824=CIRCLE('',#14799,4.7625);
#3825=CIRCLE('',#14803,4.7625);
#3826=CIRCLE('',#14807,4.7625);
#3827=CIRCLE('',#14811,4.7625);
#3828=CIRCLE('',#14815,4.7625);
#3829=CIRCLE('',#14819,4.7625);
#3830=CIRCLE('',#14823,4.7625);
#3831=CIRCLE('',#14827,4.7625);
#3832=CIRCLE('',#14831,2.74963065701559);
#3833=CIRCLE('',#14833,2.74963065701559);
#3834=CIRCLE('',#14835,2.74963065701559);
#3835=CIRCLE('',#14837,2.74963065701559);
#3836=CIRCLE('',#14839,2.74963065701559);
#3837=CIRCLE('',#14841,2.74963065701559);
#4533=LINE('',#59761,#5444);
#4534=LINE('',#60034,#5445);
#4535=LINE('',#60434,#5446);
#4536=LINE('',#60650,#5447);
#4537=LINE('',#60872,#5448);
#4538=LINE('',#61255,#5449);
#4539=LINE('',#61640,#5450);
#4540=LINE('',#62097,#5451);
#4541=LINE('',#62580,#5452);
#4542=LINE('',#63075,#5453);
#4543=LINE('',#63306,#5454);
#4544=LINE('',#63543,#5455);
#4545=LINE('',#63914,#5456);
#4546=LINE('',#64382,#5457);
#4547=LINE('',#70723,#5458);
#4548=LINE('',#70729,#5459);
#4549=LINE('',#70731,#5460);
#4550=LINE('',#70733,#5461);
#4551=LINE('',#70740,#5462);
#4552=LINE('',#70744,#5463);
#4553=LINE('',#71100,#5464);
#4554=LINE('',#71104,#5465);
#4555=LINE('',#71106,#5466);
#4556=LINE('',#71107,#5467);
#4557=LINE('',#71110,#5468);
#4558=LINE('',#71111,#5469);
#4559=LINE('',#71116,#5470);
#4560=LINE('',#71118,#5471);
#4561=LINE('',#71119,#5472);
#4562=LINE('',#71122,#5473);
#4563=LINE('',#71123,#5474);
#4564=LINE('',#71128,#5475);
#4565=LINE('',#71130,#5476);
#4566=LINE('',#71131,#5477);
#4567=LINE('',#71134,#5478);
#4568=LINE('',#71135,#5479);
#4569=LINE('',#71140,#5480);
#4570=LINE('',#71142,#5481);
#4571=LINE('',#71143,#5482);
#4572=LINE('',#71146,#5483);
#4573=LINE('',#71147,#5484);
#4574=LINE('',#71152,#5485);
#4575=LINE('',#71154,#5486);
#4576=LINE('',#71155,#5487);
#4577=LINE('',#71158,#5488);
#4578=LINE('',#71159,#5489);
#4579=LINE('',#71164,#5490);
#4580=LINE('',#71166,#5491);
#4581=LINE('',#71167,#5492);
#4582=LINE('',#71170,#5493);
#4583=LINE('',#71171,#5494);
#4584=LINE('',#71176,#5495);
#4585=LINE('',#71178,#5496);
#4586=LINE('',#71179,#5497);
#4587=LINE('',#71182,#5498);
#4588=LINE('',#71183,#5499);
#4589=LINE('',#71188,#5500);
#4590=LINE('',#71190,#5501);
#4591=LINE('',#71191,#5502);
#4592=LINE('',#71194,#5503);
#4593=LINE('',#71195,#5504);
#4594=LINE('',#71200,#5505);
#4595=LINE('',#71202,#5506);
#4596=LINE('',#71203,#5507);
#4597=LINE('',#71206,#5508);
#4598=LINE('',#71207,#5509);
#4599=LINE('',#71212,#5510);
#4600=LINE('',#71214,#5511);
#4601=LINE('',#71215,#5512);
#4602=LINE('',#71218,#5513);
#4603=LINE('',#71219,#5514);
#4604=LINE('',#71224,#5515);
#4605=LINE('',#71226,#5516);
#4606=LINE('',#71227,#5517);
#4607=LINE('',#71230,#5518);
#4608=LINE('',#71231,#5519);
#4609=LINE('',#71236,#5520);
#4610=LINE('',#71238,#5521);
#4611=LINE('',#71239,#5522);
#4612=LINE('',#71242,#5523);
#4613=LINE('',#71243,#5524);
#4614=LINE('',#71248,#5525);
#4615=LINE('',#71250,#5526);
#4616=LINE('',#71251,#5527);
#4617=LINE('',#71254,#5528);
#4618=LINE('',#71255,#5529);
#4619=LINE('',#71260,#5530);
#4620=LINE('',#71262,#5531);
#4621=LINE('',#71263,#5532);
#4622=LINE('',#71266,#5533);
#4623=LINE('',#71267,#5534);
#4624=LINE('',#71272,#5535);
#4625=LINE('',#71274,#5536);
#4626=LINE('',#71275,#5537);
#4627=LINE('',#71278,#5538);
#4628=LINE('',#71279,#5539);
#4629=LINE('',#71284,#5540);
#4630=LINE('',#71286,#5541);
#4631=LINE('',#71287,#5542);
#4632=LINE('',#71290,#5543);
#4633=LINE('',#71291,#5544);
#4634=LINE('',#71296,#5545);
#4635=LINE('',#71298,#5546);
#4636=LINE('',#71299,#5547);
#4637=LINE('',#71302,#5548);
#4638=LINE('',#71303,#5549);
#4639=LINE('',#71310,#5550);
#4640=LINE('',#71312,#5551);
#4641=LINE('',#71313,#5552);
#4642=LINE('',#71316,#5553);
#4643=LINE('',#71317,#5554);
#4644=LINE('',#71322,#5555);
#4645=LINE('',#71324,#5556);
#4646=LINE('',#71325,#5557);
#4647=LINE('',#71328,#5558);
#4648=LINE('',#71329,#5559);
#4649=LINE('',#71334,#5560);
#4650=LINE('',#71336,#5561);
#4651=LINE('',#71337,#5562);
#4652=LINE('',#71340,#5563);
#4653=LINE('',#71341,#5564);
#4654=LINE('',#71346,#5565);
#4655=LINE('',#71348,#5566);
#4656=LINE('',#71349,#5567);
#4657=LINE('',#71352,#5568);
#4658=LINE('',#71353,#5569);
#4659=LINE('',#71358,#5570);
#4660=LINE('',#71360,#5571);
#4661=LINE('',#71361,#5572);
#4662=LINE('',#71364,#5573);
#4663=LINE('',#71365,#5574);
#4664=LINE('',#71370,#5575);
#4665=LINE('',#71372,#5576);
#4666=LINE('',#71373,#5577);
#4667=LINE('',#71376,#5578);
#4668=LINE('',#71377,#5579);
#4669=LINE('',#71382,#5580);
#4670=LINE('',#71384,#5581);
#4671=LINE('',#71385,#5582);
#4672=LINE('',#71388,#5583);
#4673=LINE('',#71389,#5584);
#4674=LINE('',#71394,#5585);
#4675=LINE('',#71396,#5586);
#4676=LINE('',#71397,#5587);
#4677=LINE('',#71400,#5588);
#4678=LINE('',#71401,#5589);
#4679=LINE('',#71406,#5590);
#4680=LINE('',#71408,#5591);
#4681=LINE('',#71409,#5592);
#4682=LINE('',#71412,#5593);
#4683=LINE('',#71413,#5594);
#4684=LINE('',#71418,#5595);
#4685=LINE('',#71420,#5596);
#4686=LINE('',#71421,#5597);
#4687=LINE('',#71424,#5598);
#4688=LINE('',#71425,#5599);
#4689=LINE('',#71430,#5600);
#4690=LINE('',#71432,#5601);
#4691=LINE('',#71433,#5602);
#4692=LINE('',#71436,#5603);
#4693=LINE('',#71437,#5604);
#4694=LINE('',#71442,#5605);
#4695=LINE('',#71444,#5606);
#4696=LINE('',#71445,#5607);
#4697=LINE('',#71448,#5608);
#4698=LINE('',#71449,#5609);
#4699=LINE('',#71454,#5610);
#4700=LINE('',#71456,#5611);
#4701=LINE('',#71457,#5612);
#4702=LINE('',#71460,#5613);
#4703=LINE('',#71461,#5614);
#4704=LINE('',#71466,#5615);
#4705=LINE('',#71468,#5616);
#4706=LINE('',#71469,#5617);
#4707=LINE('',#71472,#5618);
#4708=LINE('',#71473,#5619);
#4709=LINE('',#71478,#5620);
#4710=LINE('',#71480,#5621);
#4711=LINE('',#71481,#5622);
#4712=LINE('',#71484,#5623);
#4713=LINE('',#71485,#5624);
#4714=LINE('',#71490,#5625);
#4715=LINE('',#71492,#5626);
#4716=LINE('',#71493,#5627);
#4717=LINE('',#71496,#5628);
#4718=LINE('',#71497,#5629);
#4719=LINE('',#71502,#5630);
#4720=LINE('',#71504,#5631);
#4721=LINE('',#71505,#5632);
#4722=LINE('',#71508,#5633);
#4723=LINE('',#71509,#5634);
#4724=LINE('',#71514,#5635);
#4725=LINE('',#71516,#5636);
#4726=LINE('',#71517,#5637);
#4727=LINE('',#71520,#5638);
#4728=LINE('',#71521,#5639);
#4729=LINE('',#71525,#5640);
#4730=LINE('',#71529,#5641);
#4731=LINE('',#71531,#5642);
#4732=LINE('',#71533,#5643);
#4733=LINE('',#71535,#5644);
#4734=LINE('',#71537,#5645);
#4735=LINE('',#71538,#5646);
#4736=LINE('',#71542,#5647);
#4737=LINE('',#71546,#5648);
#4738=LINE('',#71550,#5649);
#4739=LINE('',#71554,#5650);
#4740=LINE('',#71558,#5651);
#4741=LINE('',#71561,#5652);
#4742=LINE('',#71565,#5653);
#4743=LINE('',#71567,#5654);
#4744=LINE('',#71568,#5655);
#4745=LINE('',#71570,#5656);
#4746=LINE('',#71572,#5657);
#4747=LINE('',#71574,#5658);
#4748=LINE('',#71576,#5659);
#5444=VECTOR('',#17450,2.40538);
#5445=VECTOR('',#17455,2.40538);
#5446=VECTOR('',#17458,2.40538);
#5447=VECTOR('',#17461,2.40538);
#5448=VECTOR('',#17464,2.40538);
#5449=VECTOR('',#17467,2.40538);
#5450=VECTOR('',#17470,2.40538);
#5451=VECTOR('',#17473,2.40538);
#5452=VECTOR('',#17476,2.40538);
#5453=VECTOR('',#17479,2.40538);
#5454=VECTOR('',#17482,2.40538);
#5455=VECTOR('',#17485,2.40538);
#5456=VECTOR('',#17488,2.40538);
#5457=VECTOR('',#17491,2.40538);
#5458=VECTOR('',#17526,2.91023);
#5459=VECTOR('',#17533,10.);
#5460=VECTOR('',#17534,10.);
#5461=VECTOR('',#17535,10.);
#5462=VECTOR('',#17538,10.);
#5463=VECTOR('',#17539,10.);
#5464=VECTOR('',#17618,4.5625);
#5465=VECTOR('',#17623,10.);
#5466=VECTOR('',#17624,10.);
#5467=VECTOR('',#17625,10.);
#5468=VECTOR('',#17628,10.);
#5469=VECTOR('',#17629,10.);
#5470=VECTOR('',#17636,10.);
#5471=VECTOR('',#17637,10.);
#5472=VECTOR('',#17638,10.);
#5473=VECTOR('',#17641,10.);
#5474=VECTOR('',#17642,10.);
#5475=VECTOR('',#17649,10.);
#5476=VECTOR('',#17650,10.);
#5477=VECTOR('',#17651,10.);
#5478=VECTOR('',#17654,10.);
#5479=VECTOR('',#17655,10.);
#5480=VECTOR('',#17662,10.);
#5481=VECTOR('',#17663,10.);
#5482=VECTOR('',#17664,10.);
#5483=VECTOR('',#17667,10.);
#5484=VECTOR('',#17668,10.);
#5485=VECTOR('',#17675,10.);
#5486=VECTOR('',#17676,10.);
#5487=VECTOR('',#17677,10.);
#5488=VECTOR('',#17680,10.);
#5489=VECTOR('',#17681,10.);
#5490=VECTOR('',#17688,10.);
#5491=VECTOR('',#17689,10.);
#5492=VECTOR('',#17690,10.);
#5493=VECTOR('',#17693,10.);
#5494=VECTOR('',#17694,10.);
#5495=VECTOR('',#17701,10.);
#5496=VECTOR('',#17702,10.);
#5497=VECTOR('',#17703,10.);
#5498=VECTOR('',#17706,10.);
#5499=VECTOR('',#17707,10.);
#5500=VECTOR('',#17714,10.);
#5501=VECTOR('',#17715,10.);
#5502=VECTOR('',#17716,10.);
#5503=VECTOR('',#17719,10.);
#5504=VECTOR('',#17720,10.);
#5505=VECTOR('',#17727,10.);
#5506=VECTOR('',#17728,10.);
#5507=VECTOR('',#17729,10.);
#5508=VECTOR('',#17732,10.);
#5509=VECTOR('',#17733,10.);
#5510=VECTOR('',#17740,10.);
#5511=VECTOR('',#17741,10.);
#5512=VECTOR('',#17742,10.);
#5513=VECTOR('',#17745,10.);
#5514=VECTOR('',#17746,10.);
#5515=VECTOR('',#17753,10.);
#5516=VECTOR('',#17754,10.);
#5517=VECTOR('',#17755,10.);
#5518=VECTOR('',#17758,10.);
#5519=VECTOR('',#17759,10.);
#5520=VECTOR('',#17766,10.);
#5521=VECTOR('',#17767,10.);
#5522=VECTOR('',#17768,10.);
#5523=VECTOR('',#17771,10.);
#5524=VECTOR('',#17772,10.);
#5525=VECTOR('',#17779,10.);
#5526=VECTOR('',#17780,10.);
#5527=VECTOR('',#17781,10.);
#5528=VECTOR('',#17784,10.);
#5529=VECTOR('',#17785,10.);
#5530=VECTOR('',#17792,10.);
#5531=VECTOR('',#17793,10.);
#5532=VECTOR('',#17794,10.);
#5533=VECTOR('',#17797,10.);
#5534=VECTOR('',#17798,10.);
#5535=VECTOR('',#17805,10.);
#5536=VECTOR('',#17806,10.);
#5537=VECTOR('',#17807,10.);
#5538=VECTOR('',#17810,10.);
#5539=VECTOR('',#17811,10.);
#5540=VECTOR('',#17818,10.);
#5541=VECTOR('',#17819,10.);
#5542=VECTOR('',#17820,10.);
#5543=VECTOR('',#17823,10.);
#5544=VECTOR('',#17824,10.);
#5545=VECTOR('',#17831,10.);
#5546=VECTOR('',#17832,10.);
#5547=VECTOR('',#17833,10.);
#5548=VECTOR('',#17836,10.);
#5549=VECTOR('',#17837,10.);
#5550=VECTOR('',#17846,10.);
#5551=VECTOR('',#17847,10.);
#5552=VECTOR('',#17848,10.);
#5553=VECTOR('',#17851,10.);
#5554=VECTOR('',#17852,10.);
#5555=VECTOR('',#17859,10.);
#5556=VECTOR('',#17860,10.);
#5557=VECTOR('',#17861,10.);
#5558=VECTOR('',#17864,10.);
#5559=VECTOR('',#17865,10.);
#5560=VECTOR('',#17872,10.);
#5561=VECTOR('',#17873,10.);
#5562=VECTOR('',#17874,10.);
#5563=VECTOR('',#17877,10.);
#5564=VECTOR('',#17878,10.);
#5565=VECTOR('',#17885,10.);
#5566=VECTOR('',#17886,10.);
#5567=VECTOR('',#17887,10.);
#5568=VECTOR('',#17890,10.);
#5569=VECTOR('',#17891,10.);
#5570=VECTOR('',#17898,10.);
#5571=VECTOR('',#17899,10.);
#5572=VECTOR('',#17900,10.);
#5573=VECTOR('',#17903,10.);
#5574=VECTOR('',#17904,10.);
#5575=VECTOR('',#17911,10.);
#5576=VECTOR('',#17912,10.);
#5577=VECTOR('',#17913,10.);
#5578=VECTOR('',#17916,10.);
#5579=VECTOR('',#17917,10.);
#5580=VECTOR('',#17924,10.);
#5581=VECTOR('',#17925,10.);
#5582=VECTOR('',#17926,10.);
#5583=VECTOR('',#17929,10.);
#5584=VECTOR('',#17930,9.99999999999999);
#5585=VECTOR('',#17937,10.);
#5586=VECTOR('',#17938,10.);
#5587=VECTOR('',#17939,10.);
#5588=VECTOR('',#17942,10.);
#5589=VECTOR('',#17943,10.);
#5590=VECTOR('',#17950,10.);
#5591=VECTOR('',#17951,10.);
#5592=VECTOR('',#17952,10.);
#5593=VECTOR('',#17955,10.);
#5594=VECTOR('',#17956,10.);
#5595=VECTOR('',#17963,10.);
#5596=VECTOR('',#17964,10.);
#5597=VECTOR('',#17965,10.);
#5598=VECTOR('',#17968,10.);
#5599=VECTOR('',#17969,10.);
#5600=VECTOR('',#17976,10.);
#5601=VECTOR('',#17977,10.);
#5602=VECTOR('',#17978,10.);
#5603=VECTOR('',#17981,10.);
#5604=VECTOR('',#17982,10.);
#5605=VECTOR('',#17989,10.);
#5606=VECTOR('',#17990,10.);
#5607=VECTOR('',#17991,10.);
#5608=VECTOR('',#17994,10.);
#5609=VECTOR('',#17995,9.99999999999999);
#5610=VECTOR('',#18002,10.);
#5611=VECTOR('',#18003,10.);
#5612=VECTOR('',#18004,10.);
#5613=VECTOR('',#18007,10.);
#5614=VECTOR('',#18008,10.);
#5615=VECTOR('',#18015,10.);
#5616=VECTOR('',#18016,10.);
#5617=VECTOR('',#18017,10.);
#5618=VECTOR('',#18020,10.);
#5619=VECTOR('',#18021,10.);
#5620=VECTOR('',#18028,10.);
#5621=VECTOR('',#18029,10.);
#5622=VECTOR('',#18030,10.);
#5623=VECTOR('',#18033,10.);
#5624=VECTOR('',#18034,10.);
#5625=VECTOR('',#18041,10.);
#5626=VECTOR('',#18042,10.);
#5627=VECTOR('',#18043,10.);
#5628=VECTOR('',#18046,10.);
#5629=VECTOR('',#18047,10.);
#5630=VECTOR('',#18054,10.);
#5631=VECTOR('',#18055,10.);
#5632=VECTOR('',#18056,10.);
#5633=VECTOR('',#18059,10.);
#5634=VECTOR('',#18060,10.);
#5635=VECTOR('',#18067,10.);
#5636=VECTOR('',#18068,10.);
#5637=VECTOR('',#18069,10.);
#5638=VECTOR('',#18072,10.);
#5639=VECTOR('',#18073,10.);
#5640=VECTOR('',#18080,4.7625);
#5641=VECTOR('',#18083,10.);
#5642=VECTOR('',#18084,10.);
#5643=VECTOR('',#18085,9.99999999999999);
#5644=VECTOR('',#18086,10.);
#5645=VECTOR('',#18087,10.);
#5646=VECTOR('',#18088,10.);
#5647=VECTOR('',#18091,10.);
#5648=VECTOR('',#18096,10.);
#5649=VECTOR('',#18101,9.99999999999999);
#5650=VECTOR('',#18106,10.);
#5651=VECTOR('',#18111,10.);
#5652=VECTOR('',#18116,10.);
#5653=VECTOR('',#18121,2.74963065701559);
#5654=VECTOR('',#18124,10.);
#5655=VECTOR('',#18125,10.);
#5656=VECTOR('',#18128,10.);
#5657=VECTOR('',#18131,10.);
#5658=VECTOR('',#18134,10.);
#5659=VECTOR('',#18137,10.);
#6696=VERTEX_POINT('',#59759);
#6697=VERTEX_POINT('',#59760);
#6698=VERTEX_POINT('',#59762);
#6699=VERTEX_POINT('',#59917);
#6700=VERTEX_POINT('',#60032);
#6701=VERTEX_POINT('',#60033);
#6702=VERTEX_POINT('',#60035);
#6703=VERTEX_POINT('',#60233);
#6704=VERTEX_POINT('',#60432);
#6705=VERTEX_POINT('',#60433);
#6706=VERTEX_POINT('',#60623);
#6707=VERTEX_POINT('',#60648);
#6708=VERTEX_POINT('',#60649);
#6709=VERTEX_POINT('',#60651);
#6710=VERTEX_POINT('',#60680);
#6711=VERTEX_POINT('',#60870);
#6712=VERTEX_POINT('',#60871);
#6713=VERTEX_POINT('',#60873);
#6714=VERTEX_POINT('',#61253);
#6715=VERTEX_POINT('',#61254);
#6716=VERTEX_POINT('',#61450);
#6717=VERTEX_POINT('',#61638);
#6718=VERTEX_POINT('',#61639);
#6719=VERTEX_POINT('',#61641);
#6720=VERTEX_POINT('',#62095);
#6721=VERTEX_POINT('',#62096);
#6722=VERTEX_POINT('',#62370);
#6723=VERTEX_POINT('',#62578);
#6724=VERTEX_POINT('',#62579);
#6725=VERTEX_POINT('',#62581);
#6726=VERTEX_POINT('',#63073);
#6727=VERTEX_POINT('',#63074);
#6728=VERTEX_POINT('',#63274);
#6729=VERTEX_POINT('',#63304);
#6730=VERTEX_POINT('',#63305);
#6731=VERTEX_POINT('',#63307);
#6732=VERTEX_POINT('',#63326);
#6733=VERTEX_POINT('',#63541);
#6734=VERTEX_POINT('',#63542);
#6735=VERTEX_POINT('',#63544);
#6736=VERTEX_POINT('',#63912);
#6737=VERTEX_POINT('',#63913);
#6738=VERTEX_POINT('',#63915);
#6739=VERTEX_POINT('',#64380);
#6740=VERTEX_POINT('',#64381);
#6741=VERTEX_POINT('',#64762);
#6742=VERTEX_POINT('',#64763);
#6743=VERTEX_POINT('',#64834);
#6744=VERTEX_POINT('',#64836);
#6745=VERTEX_POINT('',#64842);
#6746=VERTEX_POINT('',#65054);
#6747=VERTEX_POINT('',#65065);
#6748=VERTEX_POINT('',#65274);
#6749=VERTEX_POINT('',#65486);
#6750=VERTEX_POINT('',#65698);
#6751=VERTEX_POINT('',#65710);
#6752=VERTEX_POINT('',#65919);
#6753=VERTEX_POINT('',#66128);
#6754=VERTEX_POINT('',#66140);
#6755=VERTEX_POINT('',#66349);
#6756=VERTEX_POINT('',#66558);
#6757=VERTEX_POINT('',#66770);
#6758=VERTEX_POINT('',#66781);
#6759=VERTEX_POINT('',#66993);
#6760=VERTEX_POINT('',#67070);
#6761=VERTEX_POINT('',#67072);
#6762=VERTEX_POINT('',#67078);
#6763=VERTEX_POINT('',#67089);
#6764=VERTEX_POINT('',#67298);
#6765=VERTEX_POINT('',#67510);
#6766=VERTEX_POINT('',#67521);
#6767=VERTEX_POINT('',#67730);
#6768=VERTEX_POINT('',#67942);
#6769=VERTEX_POINT('',#68154);
#6770=VERTEX_POINT('',#68165);
#6771=VERTEX_POINT('',#68377);
#6772=VERTEX_POINT('',#68589);
#6773=VERTEX_POINT('',#68600);
#6774=VERTEX_POINT('',#68809);
#6775=VERTEX_POINT('',#69227);
#6776=VERTEX_POINT('',#69406);
#6777=VERTEX_POINT('',#69408);
#6778=VERTEX_POINT('',#69555);
#6779=VERTEX_POINT('',#69556);
#6780=VERTEX_POINT('',#69652);
#6781=VERTEX_POINT('',#70227);
#6782=VERTEX_POINT('',#70228);
#6783=VERTEX_POINT('',#70715);
#6784=VERTEX_POINT('',#70719);
#6785=VERTEX_POINT('',#70722);
#6786=VERTEX_POINT('',#70727);
#6787=VERTEX_POINT('',#70728);
#6788=VERTEX_POINT('',#70730);
#6789=VERTEX_POINT('',#70732);
#6790=VERTEX_POINT('',#70738);
#6791=VERTEX_POINT('',#70739);
#6792=VERTEX_POINT('',#70748);
#6793=VERTEX_POINT('',#70749);
#6794=VERTEX_POINT('',#70753);
#6795=VERTEX_POINT('',#70755);
#6796=VERTEX_POINT('',#70759);
#6797=VERTEX_POINT('',#70763);
#6798=VERTEX_POINT('',#70765);
#6799=VERTEX_POINT('',#70769);
#6800=VERTEX_POINT('',#70773);
#6801=VERTEX_POINT('',#70775);
#6802=VERTEX_POINT('',#70779);
#6803=VERTEX_POINT('',#70783);
#6804=VERTEX_POINT('',#70785);
#6805=VERTEX_POINT('',#70789);
#6806=VERTEX_POINT('',#70793);
#6807=VERTEX_POINT('',#70795);
#6808=VERTEX_POINT('',#70799);
#6809=VERTEX_POINT('',#70803);
#6810=VERTEX_POINT('',#70805);
#6811=VERTEX_POINT('',#70809);
#6812=VERTEX_POINT('',#70813);
#6813=VERTEX_POINT('',#70815);
#6814=VERTEX_POINT('',#70819);
#6815=VERTEX_POINT('',#70823);
#6816=VERTEX_POINT('',#70825);
#6817=VERTEX_POINT('',#70829);
#6818=VERTEX_POINT('',#70833);
#6819=VERTEX_POINT('',#70835);
#6820=VERTEX_POINT('',#70839);
#6821=VERTEX_POINT('',#70843);
#6822=VERTEX_POINT('',#70845);
#6823=VERTEX_POINT('',#70849);
#6824=VERTEX_POINT('',#70853);
#6825=VERTEX_POINT('',#70855);
#6826=VERTEX_POINT('',#70859);
#6827=VERTEX_POINT('',#70863);
#6828=VERTEX_POINT('',#70865);
#6829=VERTEX_POINT('',#70869);
#6830=VERTEX_POINT('',#70873);
#6831=VERTEX_POINT('',#70875);
#6832=VERTEX_POINT('',#70879);
#6833=VERTEX_POINT('',#70883);
#6834=VERTEX_POINT('',#70885);
#6835=VERTEX_POINT('',#70889);
#6836=VERTEX_POINT('',#70893);
#6837=VERTEX_POINT('',#70895);
#6838=VERTEX_POINT('',#70899);
#6839=VERTEX_POINT('',#70903);
#6840=VERTEX_POINT('',#70905);
#6841=VERTEX_POINT('',#70909);
#6842=VERTEX_POINT('',#70913);
#6843=VERTEX_POINT('',#70915);
#6844=VERTEX_POINT('',#70919);
#6845=VERTEX_POINT('',#70923);
#6846=VERTEX_POINT('',#70925);
#6847=VERTEX_POINT('',#70929);
#6848=VERTEX_POINT('',#70934);
#6849=VERTEX_POINT('',#70936);
#6850=VERTEX_POINT('',#70940);
#6851=VERTEX_POINT('',#70944);
#6852=VERTEX_POINT('',#70946);
#6853=VERTEX_POINT('',#70950);
#6854=VERTEX_POINT('',#70954);
#6855=VERTEX_POINT('',#70956);
#6856=VERTEX_POINT('',#70960);
#6857=VERTEX_POINT('',#70964);
#6858=VERTEX_POINT('',#70966);
#6859=VERTEX_POINT('',#70970);
#6860=VERTEX_POINT('',#70974);
#6861=VERTEX_POINT('',#70976);
#6862=VERTEX_POINT('',#70980);
#6863=VERTEX_POINT('',#70984);
#6864=VERTEX_POINT('',#70986);
#6865=VERTEX_POINT('',#70990);
#6866=VERTEX_POINT('',#70994);
#6867=VERTEX_POINT('',#70996);
#6868=VERTEX_POINT('',#71000);
#6869=VERTEX_POINT('',#71004);
#6870=VERTEX_POINT('',#71006);
#6871=VERTEX_POINT('',#71010);
#6872=VERTEX_POINT('',#71014);
#6873=VERTEX_POINT('',#71016);
#6874=VERTEX_POINT('',#71020);
#6875=VERTEX_POINT('',#71024);
#6876=VERTEX_POINT('',#71026);
#6877=VERTEX_POINT('',#71030);
#6878=VERTEX_POINT('',#71034);
#6879=VERTEX_POINT('',#71036);
#6880=VERTEX_POINT('',#71040);
#6881=VERTEX_POINT('',#71044);
#6882=VERTEX_POINT('',#71046);
#6883=VERTEX_POINT('',#71050);
#6884=VERTEX_POINT('',#71054);
#6885=VERTEX_POINT('',#71056);
#6886=VERTEX_POINT('',#71060);
#6887=VERTEX_POINT('',#71064);
#6888=VERTEX_POINT('',#71066);
#6889=VERTEX_POINT('',#71070);
#6890=VERTEX_POINT('',#71074);
#6891=VERTEX_POINT('',#71076);
#6892=VERTEX_POINT('',#71080);
#6893=VERTEX_POINT('',#71084);
#6894=VERTEX_POINT('',#71086);
#6895=VERTEX_POINT('',#71090);
#6896=VERTEX_POINT('',#71094);
#6897=VERTEX_POINT('',#71099);
#6898=VERTEX_POINT('',#71103);
#6899=VERTEX_POINT('',#71105);
#6900=VERTEX_POINT('',#71109);
#6901=VERTEX_POINT('',#71115);
#6902=VERTEX_POINT('',#71117);
#6903=VERTEX_POINT('',#71121);
#6904=VERTEX_POINT('',#71127);
#6905=VERTEX_POINT('',#71129);
#6906=VERTEX_POINT('',#71133);
#6907=VERTEX_POINT('',#71139);
#6908=VERTEX_POINT('',#71141);
#6909=VERTEX_POINT('',#71145);
#6910=VERTEX_POINT('',#71151);
#6911=VERTEX_POINT('',#71153);
#6912=VERTEX_POINT('',#71157);
#6913=VERTEX_POINT('',#71163);
#6914=VERTEX_POINT('',#71165);
#6915=VERTEX_POINT('',#71169);
#6916=VERTEX_POINT('',#71175);
#6917=VERTEX_POINT('',#71177);
#6918=VERTEX_POINT('',#71181);
#6919=VERTEX_POINT('',#71187);
#6920=VERTEX_POINT('',#71189);
#6921=VERTEX_POINT('',#71193);
#6922=VERTEX_POINT('',#71199);
#6923=VERTEX_POINT('',#71201);
#6924=VERTEX_POINT('',#71205);
#6925=VERTEX_POINT('',#71211);
#6926=VERTEX_POINT('',#71213);
#6927=VERTEX_POINT('',#71217);
#6928=VERTEX_POINT('',#71223);
#6929=VERTEX_POINT('',#71225);
#6930=VERTEX_POINT('',#71229);
#6931=VERTEX_POINT('',#71235);
#6932=VERTEX_POINT('',#71237);
#6933=VERTEX_POINT('',#71241);
#6934=VERTEX_POINT('',#71247);
#6935=VERTEX_POINT('',#71249);
#6936=VERTEX_POINT('',#71253);
#6937=VERTEX_POINT('',#71259);
#6938=VERTEX_POINT('',#71261);
#6939=VERTEX_POINT('',#71265);
#6940=VERTEX_POINT('',#71271);
#6941=VERTEX_POINT('',#71273);
#6942=VERTEX_POINT('',#71277);
#6943=VERTEX_POINT('',#71283);
#6944=VERTEX_POINT('',#71285);
#6945=VERTEX_POINT('',#71289);
#6946=VERTEX_POINT('',#71295);
#6947=VERTEX_POINT('',#71297);
#6948=VERTEX_POINT('',#71301);
#6949=VERTEX_POINT('',#71305);
#6950=VERTEX_POINT('',#71309);
#6951=VERTEX_POINT('',#71311);
#6952=VERTEX_POINT('',#71315);
#6953=VERTEX_POINT('',#71321);
#6954=VERTEX_POINT('',#71323);
#6955=VERTEX_POINT('',#71327);
#6956=VERTEX_POINT('',#71333);
#6957=VERTEX_POINT('',#71335);
#6958=VERTEX_POINT('',#71339);
#6959=VERTEX_POINT('',#71345);
#6960=VERTEX_POINT('',#71347);
#6961=VERTEX_POINT('',#71351);
#6962=VERTEX_POINT('',#71357);
#6963=VERTEX_POINT('',#71359);
#6964=VERTEX_POINT('',#71363);
#6965=VERTEX_POINT('',#71369);
#6966=VERTEX_POINT('',#71371);
#6967=VERTEX_POINT('',#71375);
#6968=VERTEX_POINT('',#71381);
#6969=VERTEX_POINT('',#71383);
#6970=VERTEX_POINT('',#71387);
#6971=VERTEX_POINT('',#71393);
#6972=VERTEX_POINT('',#71395);
#6973=VERTEX_POINT('',#71399);
#6974=VERTEX_POINT('',#71405);
#6975=VERTEX_POINT('',#71407);
#6976=VERTEX_POINT('',#71411);
#6977=VERTEX_POINT('',#71417);
#6978=VERTEX_POINT('',#71419);
#6979=VERTEX_POINT('',#71423);
#6980=VERTEX_POINT('',#71429);
#6981=VERTEX_POINT('',#71431);
#6982=VERTEX_POINT('',#71435);
#6983=VERTEX_POINT('',#71441);
#6984=VERTEX_POINT('',#71443);
#6985=VERTEX_POINT('',#71447);
#6986=VERTEX_POINT('',#71453);
#6987=VERTEX_POINT('',#71455);
#6988=VERTEX_POINT('',#71459);
#6989=VERTEX_POINT('',#71465);
#6990=VERTEX_POINT('',#71467);
#6991=VERTEX_POINT('',#71471);
#6992=VERTEX_POINT('',#71477);
#6993=VERTEX_POINT('',#71479);
#6994=VERTEX_POINT('',#71483);
#6995=VERTEX_POINT('',#71489);
#6996=VERTEX_POINT('',#71491);
#6997=VERTEX_POINT('',#71495);
#6998=VERTEX_POINT('',#71501);
#6999=VERTEX_POINT('',#71503);
#7000=VERTEX_POINT('',#71507);
#7001=VERTEX_POINT('',#71513);
#7002=VERTEX_POINT('',#71515);
#7003=VERTEX_POINT('',#71519);
#7004=VERTEX_POINT('',#71527);
#7005=VERTEX_POINT('',#71528);
#7006=VERTEX_POINT('',#71530);
#7007=VERTEX_POINT('',#71532);
#7008=VERTEX_POINT('',#71534);
#7009=VERTEX_POINT('',#71536);
#7010=VERTEX_POINT('',#71540);
#7011=VERTEX_POINT('',#71541);
#7012=VERTEX_POINT('',#71545);
#7013=VERTEX_POINT('',#71549);
#7014=VERTEX_POINT('',#71553);
#7015=VERTEX_POINT('',#71557);
#7016=VERTEX_POINT('',#71564);
#8500=EDGE_CURVE('',#6696,#6697,#4533,.T.);
#8501=EDGE_CURVE('',#6698,#6696,#1399,.T.);
#8502=EDGE_CURVE('',#6699,#6698,#3746,.T.);
#8503=EDGE_CURVE('',#6699,#6697,#1400,.T.);
#8504=EDGE_CURVE('',#6700,#6701,#4534,.T.);
#8505=EDGE_CURVE('',#6702,#6700,#1401,.F.);
#8506=EDGE_CURVE('',#6696,#6702,#1402,.T.);
#8507=EDGE_CURVE('',#6697,#6703,#1403,.T.);
#8508=EDGE_CURVE('',#6703,#6701,#1404,.T.);
#8509=EDGE_CURVE('',#6704,#6705,#4535,.T.);
#8510=EDGE_CURVE('',#6700,#6704,#1405,.F.);
#8511=EDGE_CURVE('',#6701,#6706,#1406,.T.);
#8512=EDGE_CURVE('',#6706,#6705,#1407,.T.);
#8513=EDGE_CURVE('',#6707,#6708,#4536,.T.);
#8514=EDGE_CURVE('',#6709,#6707,#1408,.T.);
#8515=EDGE_CURVE('',#6704,#6709,#1409,.F.);
#8516=EDGE_CURVE('',#6705,#6710,#1410,.T.);
#8517=EDGE_CURVE('',#6710,#6708,#1411,.T.);
#8518=EDGE_CURVE('',#6711,#6712,#4537,.T.);
#8519=EDGE_CURVE('',#6713,#6711,#1412,.F.);
#8520=EDGE_CURVE('',#6707,#6713,#1413,.T.);
#8521=EDGE_CURVE('',#6708,#6712,#1414,.T.);
#8522=EDGE_CURVE('',#6714,#6715,#4538,.T.);
#8523=EDGE_CURVE('',#6711,#6714,#1415,.F.);
#8524=EDGE_CURVE('',#6712,#6716,#1416,.T.);
#8525=EDGE_CURVE('',#6716,#6715,#1417,.T.);
#8526=EDGE_CURVE('',#6717,#6718,#4539,.T.);
#8527=EDGE_CURVE('',#6719,#6717,#1418,.F.);
#8528=EDGE_CURVE('',#6714,#6719,#1419,.F.);
#8529=EDGE_CURVE('',#6715,#6718,#1420,.T.);
#8530=EDGE_CURVE('',#6720,#6721,#4540,.T.);
#8531=EDGE_CURVE('',#6717,#6720,#1421,.F.);
#8532=EDGE_CURVE('',#6718,#6722,#1422,.T.);
#8533=EDGE_CURVE('',#6722,#6721,#1423,.T.);
#8534=EDGE_CURVE('',#6723,#6724,#4541,.T.);
#8535=EDGE_CURVE('',#6725,#6723,#1424,.F.);
#8536=EDGE_CURVE('',#6720,#6725,#1425,.F.);
#8537=EDGE_CURVE('',#6721,#6724,#1426,.T.);
#8538=EDGE_CURVE('',#6726,#6727,#4542,.T.);
#8539=EDGE_CURVE('',#6723,#6726,#1427,.F.);
#8540=EDGE_CURVE('',#6724,#6728,#1428,.T.);
#8541=EDGE_CURVE('',#6728,#6727,#1429,.T.);
#8542=EDGE_CURVE('',#6729,#6730,#4543,.T.);
#8543=EDGE_CURVE('',#6731,#6729,#1430,.T.);
#8544=EDGE_CURVE('',#6726,#6731,#1431,.F.);
#8545=EDGE_CURVE('',#6727,#6732,#1432,.T.);
#8546=EDGE_CURVE('',#6732,#6730,#1433,.T.);
#8547=EDGE_CURVE('',#6733,#6734,#4544,.T.);
#8548=EDGE_CURVE('',#6735,#6733,#1434,.T.);
#8549=EDGE_CURVE('',#6729,#6735,#1435,.T.);
#8550=EDGE_CURVE('',#6730,#6734,#1436,.T.);
#8551=EDGE_CURVE('',#6736,#6737,#4545,.T.);
#8552=EDGE_CURVE('',#6738,#6736,#1437,.F.);
#8553=EDGE_CURVE('',#6733,#6738,#1438,.T.);
#8554=EDGE_CURVE('',#6734,#6737,#1439,.T.);
#8555=EDGE_CURVE('',#6739,#6740,#4546,.T.);
#8556=EDGE_CURVE('',#6736,#6739,#1440,.F.);
#8557=EDGE_CURVE('',#6737,#6740,#1441,.T.);
#8558=EDGE_CURVE('',#6741,#6742,#1442,.T.);
#8559=EDGE_CURVE('',#6743,#6742,#3747,.T.);
#8560=EDGE_CURVE('',#6743,#6744,#1443,.T.);
#8561=EDGE_CURVE('',#6744,#6745,#1444,.T.);
#8562=EDGE_CURVE('',#6745,#6746,#1445,.T.);
#8563=EDGE_CURVE('',#6746,#6747,#1446,.T.);
#8564=EDGE_CURVE('',#6747,#6748,#1447,.T.);
#8565=EDGE_CURVE('',#6748,#6749,#1448,.T.);
#8566=EDGE_CURVE('',#6749,#6750,#1449,.T.);
#8567=EDGE_CURVE('',#6750,#6751,#1450,.T.);
#8568=EDGE_CURVE('',#6751,#6752,#1451,.T.);
#8569=EDGE_CURVE('',#6752,#6753,#1452,.T.);
#8570=EDGE_CURVE('',#6753,#6754,#1453,.T.);
#8571=EDGE_CURVE('',#6754,#6755,#1454,.T.);
#8572=EDGE_CURVE('',#6755,#6756,#1455,.T.);
#8573=EDGE_CURVE('',#6756,#6757,#1456,.T.);
#8574=EDGE_CURVE('',#6757,#6758,#1457,.T.);
#8575=EDGE_CURVE('',#6758,#6759,#1458,.T.);
#8576=EDGE_CURVE('',#6760,#6759,#3748,.T.);
#8577=EDGE_CURVE('',#6760,#6761,#1459,.T.);
#8578=EDGE_CURVE('',#6761,#6762,#1460,.T.);
#8579=EDGE_CURVE('',#6762,#6763,#1461,.T.);
#8580=EDGE_CURVE('',#6763,#6764,#1462,.T.);
#8581=EDGE_CURVE('',#6764,#6765,#1463,.T.);
#8582=EDGE_CURVE('',#6765,#6766,#1464,.T.);
#8583=EDGE_CURVE('',#6766,#6767,#1465,.T.);
#8584=EDGE_CURVE('',#6767,#6768,#1466,.T.);
#8585=EDGE_CURVE('',#6768,#6769,#1467,.T.);
#8586=EDGE_CURVE('',#6769,#6770,#1468,.T.);
#8587=EDGE_CURVE('',#6770,#6771,#1469,.T.);
#8588=EDGE_CURVE('',#6771,#6772,#1470,.T.);
#8589=EDGE_CURVE('',#6772,#6773,#1471,.T.);
#8590=EDGE_CURVE('',#6773,#6774,#1472,.T.);
#8591=EDGE_CURVE('',#6774,#6741,#1473,.T.);
#8592=EDGE_CURVE('',#6740,#6775,#1474,.T.);
#8593=EDGE_CURVE('',#6776,#6775,#3749,.T.);
#8594=EDGE_CURVE('',#6777,#6776,#1475,.T.);
#8595=EDGE_CURVE('',#6739,#6777,#1476,.F.);
#8596=EDGE_CURVE('',#6778,#6779,#3750,.T.);
#8597=EDGE_CURVE('',#6778,#6776,#1477,.T.);
#8598=EDGE_CURVE('',#6775,#6780,#1478,.T.);
#8599=EDGE_CURVE('',#6780,#6760,#1479,.T.);
#8600=EDGE_CURVE('',#6779,#6760,#3751,.T.);
#8601=EDGE_CURVE('',#6759,#6778,#1480,.T.);
#8602=EDGE_CURVE('',#6698,#6743,#1481,.T.);
#8603=EDGE_CURVE('',#6781,#6782,#3752,.T.);
#8604=EDGE_CURVE('',#6781,#6699,#1482,.T.);
#8605=EDGE_CURVE('',#6782,#6743,#3753,.T.);
#8606=EDGE_CURVE('',#6742,#6781,#1483,.T.);
#8607=EDGE_CURVE('',#6783,#6783,#3754,.T.);
#8608=EDGE_CURVE('',#6783,#6782,#3755,.T.);
#8609=EDGE_CURVE('',#6784,#6784,#3756,.T.);
#8610=EDGE_CURVE('',#6779,#6785,#4547,.T.);
#8611=EDGE_CURVE('',#6785,#6785,#3757,.T.);
#8612=EDGE_CURVE('',#6786,#6787,#4548,.T.);
#8613=EDGE_CURVE('',#6786,#6788,#4549,.T.);
#8614=EDGE_CURVE('',#6789,#6788,#4550,.T.);
#8615=EDGE_CURVE('',#6787,#6789,#931,.T.);
#8616=EDGE_CURVE('',#6790,#6791,#4551,.T.);
#8617=EDGE_CURVE('',#6789,#6790,#932,.T.);
#8618=EDGE_CURVE('',#6788,#6791,#4552,.T.);
#8619=EDGE_CURVE('',#6791,#6786,#3758,.T.);
#8620=EDGE_CURVE('',#6792,#6793,#933,.T.);
#8621=EDGE_CURVE('',#6793,#6794,#3759,.T.);
#8622=EDGE_CURVE('',#6794,#6795,#934,.T.);
#8623=EDGE_CURVE('',#6795,#6796,#935,.T.);
#8624=EDGE_CURVE('',#6796,#6797,#3760,.T.);
#8625=EDGE_CURVE('',#6797,#6798,#936,.T.);
#8626=EDGE_CURVE('',#6798,#6799,#937,.T.);
#8627=EDGE_CURVE('',#6799,#6800,#3761,.T.);
#8628=EDGE_CURVE('',#6800,#6801,#938,.T.);
#8629=EDGE_CURVE('',#6801,#6802,#939,.T.);
#8630=EDGE_CURVE('',#6802,#6803,#3762,.T.);
#8631=EDGE_CURVE('',#6803,#6804,#940,.T.);
#8632=EDGE_CURVE('',#6804,#6805,#941,.T.);
#8633=EDGE_CURVE('',#6805,#6806,#3763,.T.);
#8634=EDGE_CURVE('',#6806,#6807,#942,.T.);
#8635=EDGE_CURVE('',#6807,#6808,#943,.T.);
#8636=EDGE_CURVE('',#6808,#6809,#3764,.T.);
#8637=EDGE_CURVE('',#6809,#6810,#944,.T.);
#8638=EDGE_CURVE('',#6810,#6811,#945,.T.);
#8639=EDGE_CURVE('',#6811,#6812,#3765,.T.);
#8640=EDGE_CURVE('',#6812,#6813,#946,.T.);
#8641=EDGE_CURVE('',#6813,#6814,#947,.T.);
#8642=EDGE_CURVE('',#6814,#6815,#3766,.T.);
#8643=EDGE_CURVE('',#6815,#6816,#948,.T.);
#8644=EDGE_CURVE('',#6816,#6817,#949,.T.);
#8645=EDGE_CURVE('',#6817,#6818,#3767,.T.);
#8646=EDGE_CURVE('',#6818,#6819,#950,.T.);
#8647=EDGE_CURVE('',#6819,#6820,#951,.T.);
#8648=EDGE_CURVE('',#6820,#6821,#3768,.T.);
#8649=EDGE_CURVE('',#6821,#6822,#952,.T.);
#8650=EDGE_CURVE('',#6822,#6823,#953,.T.);
#8651=EDGE_CURVE('',#6823,#6824,#3769,.T.);
#8652=EDGE_CURVE('',#6824,#6825,#954,.T.);
#8653=EDGE_CURVE('',#6825,#6826,#955,.T.);
#8654=EDGE_CURVE('',#6826,#6827,#3770,.T.);
#8655=EDGE_CURVE('',#6827,#6828,#956,.T.);
#8656=EDGE_CURVE('',#6828,#6829,#957,.T.);
#8657=EDGE_CURVE('',#6829,#6830,#3771,.T.);
#8658=EDGE_CURVE('',#6830,#6831,#958,.T.);
#8659=EDGE_CURVE('',#6831,#6832,#959,.T.);
#8660=EDGE_CURVE('',#6832,#6833,#3772,.T.);
#8661=EDGE_CURVE('',#6833,#6834,#960,.T.);
#8662=EDGE_CURVE('',#6834,#6835,#961,.T.);
#8663=EDGE_CURVE('',#6835,#6836,#3773,.T.);
#8664=EDGE_CURVE('',#6836,#6837,#962,.T.);
#8665=EDGE_CURVE('',#6837,#6838,#963,.T.);
#8666=EDGE_CURVE('',#6838,#6839,#3774,.T.);
#8667=EDGE_CURVE('',#6839,#6840,#964,.T.);
#8668=EDGE_CURVE('',#6840,#6841,#965,.T.);
#8669=EDGE_CURVE('',#6841,#6842,#3775,.T.);
#8670=EDGE_CURVE('',#6842,#6843,#966,.T.);
#8671=EDGE_CURVE('',#6843,#6844,#967,.T.);
#8672=EDGE_CURVE('',#6844,#6845,#3776,.T.);
#8673=EDGE_CURVE('',#6845,#6846,#968,.T.);
#8674=EDGE_CURVE('',#6846,#6847,#969,.T.);
#8675=EDGE_CURVE('',#6847,#6787,#3777,.T.);
#8676=EDGE_CURVE('',#6790,#6848,#3778,.T.);
#8677=EDGE_CURVE('',#6848,#6849,#970,.T.);
#8678=EDGE_CURVE('',#6849,#6850,#971,.T.);
#8679=EDGE_CURVE('',#6850,#6851,#3779,.T.);
#8680=EDGE_CURVE('',#6851,#6852,#972,.T.);
#8681=EDGE_CURVE('',#6852,#6853,#973,.T.);
#8682=EDGE_CURVE('',#6853,#6854,#3780,.T.);
#8683=EDGE_CURVE('',#6854,#6855,#974,.T.);
#8684=EDGE_CURVE('',#6855,#6856,#975,.T.);
#8685=EDGE_CURVE('',#6856,#6857,#3781,.T.);
#8686=EDGE_CURVE('',#6857,#6858,#976,.T.);
#8687=EDGE_CURVE('',#6858,#6859,#977,.T.);
#8688=EDGE_CURVE('',#6859,#6860,#3782,.T.);
#8689=EDGE_CURVE('',#6860,#6861,#978,.T.);
#8690=EDGE_CURVE('',#6861,#6862,#979,.T.);
#8691=EDGE_CURVE('',#6862,#6863,#3783,.T.);
#8692=EDGE_CURVE('',#6863,#6864,#980,.T.);
#8693=EDGE_CURVE('',#6864,#6865,#981,.T.);
#8694=EDGE_CURVE('',#6865,#6866,#3784,.T.);
#8695=EDGE_CURVE('',#6866,#6867,#982,.T.);
#8696=EDGE_CURVE('',#6867,#6868,#983,.T.);
#8697=EDGE_CURVE('',#6868,#6869,#3785,.T.);
#8698=EDGE_CURVE('',#6869,#6870,#984,.T.);
#8699=EDGE_CURVE('',#6870,#6871,#985,.T.);
#8700=EDGE_CURVE('',#6871,#6872,#3786,.T.);
#8701=EDGE_CURVE('',#6872,#6873,#986,.T.);
#8702=EDGE_CURVE('',#6873,#6874,#987,.T.);
#8703=EDGE_CURVE('',#6874,#6875,#3787,.T.);
#8704=EDGE_CURVE('',#6875,#6876,#988,.T.);
#8705=EDGE_CURVE('',#6876,#6877,#989,.T.);
#8706=EDGE_CURVE('',#6877,#6878,#3788,.T.);
#8707=EDGE_CURVE('',#6878,#6879,#990,.T.);
#8708=EDGE_CURVE('',#6879,#6880,#991,.T.);
#8709=EDGE_CURVE('',#6880,#6881,#3789,.T.);
#8710=EDGE_CURVE('',#6881,#6882,#992,.T.);
#8711=EDGE_CURVE('',#6882,#6883,#993,.T.);
#8712=EDGE_CURVE('',#6883,#6884,#3790,.T.);
#8713=EDGE_CURVE('',#6884,#6885,#994,.T.);
#8714=EDGE_CURVE('',#6885,#6886,#995,.T.);
#8715=EDGE_CURVE('',#6886,#6887,#3791,.T.);
#8716=EDGE_CURVE('',#6887,#6888,#996,.T.);
#8717=EDGE_CURVE('',#6888,#6889,#997,.T.);
#8718=EDGE_CURVE('',#6889,#6890,#3792,.T.);
#8719=EDGE_CURVE('',#6890,#6891,#998,.T.);
#8720=EDGE_CURVE('',#6891,#6892,#999,.T.);
#8721=EDGE_CURVE('',#6892,#6893,#3793,.T.);
#8722=EDGE_CURVE('',#6893,#6894,#1000,.T.);
#8723=EDGE_CURVE('',#6894,#6895,#1001,.T.);
#8724=EDGE_CURVE('',#6895,#6896,#3794,.T.);
#8725=EDGE_CURVE('',#6896,#6792,#1002,.T.);
#8726=EDGE_CURVE('',#6792,#6897,#4553,.T.);
#8727=EDGE_CURVE('',#6897,#6897,#3795,.T.);
#8728=EDGE_CURVE('',#6898,#6848,#4554,.T.);
#8729=EDGE_CURVE('',#6898,#6899,#4555,.T.);
#8730=EDGE_CURVE('',#6849,#6899,#4556,.T.);
#8731=EDGE_CURVE('',#6850,#6900,#4557,.T.);
#8732=EDGE_CURVE('',#6899,#6900,#4558,.T.);
#8733=EDGE_CURVE('',#6900,#6898,#3796,.T.);
#8734=EDGE_CURVE('',#6901,#6851,#4559,.T.);
#8735=EDGE_CURVE('',#6901,#6902,#4560,.T.);
#8736=EDGE_CURVE('',#6852,#6902,#4561,.T.);
#8737=EDGE_CURVE('',#6853,#6903,#4562,.T.);
#8738=EDGE_CURVE('',#6902,#6903,#4563,.T.);
#8739=EDGE_CURVE('',#6903,#6901,#3797,.T.);
#8740=EDGE_CURVE('',#6904,#6854,#4564,.T.);
#8741=EDGE_CURVE('',#6904,#6905,#4565,.T.);
#8742=EDGE_CURVE('',#6855,#6905,#4566,.T.);
#8743=EDGE_CURVE('',#6856,#6906,#4567,.T.);
#8744=EDGE_CURVE('',#6905,#6906,#4568,.T.);
#8745=EDGE_CURVE('',#6906,#6904,#3798,.T.);
#8746=EDGE_CURVE('',#6907,#6857,#4569,.T.);
#8747=EDGE_CURVE('',#6907,#6908,#4570,.T.);
#8748=EDGE_CURVE('',#6858,#6908,#4571,.T.);
#8749=EDGE_CURVE('',#6859,#6909,#4572,.T.);
#8750=EDGE_CURVE('',#6908,#6909,#4573,.T.);
#8751=EDGE_CURVE('',#6909,#6907,#3799,.T.);
#8752=EDGE_CURVE('',#6910,#6860,#4574,.T.);
#8753=EDGE_CURVE('',#6910,#6911,#4575,.T.);
#8754=EDGE_CURVE('',#6861,#6911,#4576,.T.);
#8755=EDGE_CURVE('',#6862,#6912,#4577,.T.);
#8756=EDGE_CURVE('',#6911,#6912,#4578,.T.);
#8757=EDGE_CURVE('',#6912,#6910,#3800,.T.);
#8758=EDGE_CURVE('',#6913,#6863,#4579,.T.);
#8759=EDGE_CURVE('',#6913,#6914,#4580,.T.);
#8760=EDGE_CURVE('',#6864,#6914,#4581,.T.);
#8761=EDGE_CURVE('',#6865,#6915,#4582,.T.);
#8762=EDGE_CURVE('',#6914,#6915,#4583,.T.);
#8763=EDGE_CURVE('',#6915,#6913,#3801,.T.);
#8764=EDGE_CURVE('',#6916,#6866,#4584,.T.);
#8765=EDGE_CURVE('',#6916,#6917,#4585,.T.);
#8766=EDGE_CURVE('',#6867,#6917,#4586,.T.);
#8767=EDGE_CURVE('',#6868,#6918,#4587,.T.);
#8768=EDGE_CURVE('',#6917,#6918,#4588,.T.);
#8769=EDGE_CURVE('',#6918,#6916,#3802,.T.);
#8770=EDGE_CURVE('',#6919,#6869,#4589,.T.);
#8771=EDGE_CURVE('',#6919,#6920,#4590,.T.);
#8772=EDGE_CURVE('',#6870,#6920,#4591,.T.);
#8773=EDGE_CURVE('',#6871,#6921,#4592,.T.);
#8774=EDGE_CURVE('',#6920,#6921,#4593,.T.);
#8775=EDGE_CURVE('',#6921,#6919,#3803,.T.);
#8776=EDGE_CURVE('',#6922,#6872,#4594,.T.);
#8777=EDGE_CURVE('',#6922,#6923,#4595,.T.);
#8778=EDGE_CURVE('',#6873,#6923,#4596,.T.);
#8779=EDGE_CURVE('',#6874,#6924,#4597,.T.);
#8780=EDGE_CURVE('',#6923,#6924,#4598,.T.);
#8781=EDGE_CURVE('',#6924,#6922,#3804,.T.);
#8782=EDGE_CURVE('',#6925,#6875,#4599,.T.);
#8783=EDGE_CURVE('',#6925,#6926,#4600,.T.);
#8784=EDGE_CURVE('',#6876,#6926,#4601,.T.);
#8785=EDGE_CURVE('',#6877,#6927,#4602,.T.);
#8786=EDGE_CURVE('',#6926,#6927,#4603,.T.);
#8787=EDGE_CURVE('',#6927,#6925,#3805,.T.);
#8788=EDGE_CURVE('',#6928,#6878,#4604,.T.);
#8789=EDGE_CURVE('',#6928,#6929,#4605,.T.);
#8790=EDGE_CURVE('',#6879,#6929,#4606,.T.);
#8791=EDGE_CURVE('',#6880,#6930,#4607,.T.);
#8792=EDGE_CURVE('',#6929,#6930,#4608,.T.);
#8793=EDGE_CURVE('',#6930,#6928,#3806,.T.);
#8794=EDGE_CURVE('',#6931,#6881,#4609,.T.);
#8795=EDGE_CURVE('',#6931,#6932,#4610,.T.);
#8796=EDGE_CURVE('',#6882,#6932,#4611,.T.);
#8797=EDGE_CURVE('',#6883,#6933,#4612,.T.);
#8798=EDGE_CURVE('',#6932,#6933,#4613,.T.);
#8799=EDGE_CURVE('',#6933,#6931,#3807,.T.);
#8800=EDGE_CURVE('',#6934,#6884,#4614,.T.);
#8801=EDGE_CURVE('',#6934,#6935,#4615,.T.);
#8802=EDGE_CURVE('',#6885,#6935,#4616,.T.);
#8803=EDGE_CURVE('',#6886,#6936,#4617,.T.);
#8804=EDGE_CURVE('',#6935,#6936,#4618,.T.);
#8805=EDGE_CURVE('',#6936,#6934,#3808,.T.);
#8806=EDGE_CURVE('',#6937,#6887,#4619,.T.);
#8807=EDGE_CURVE('',#6937,#6938,#4620,.T.);
#8808=EDGE_CURVE('',#6888,#6938,#4621,.T.);
#8809=EDGE_CURVE('',#6889,#6939,#4622,.T.);
#8810=EDGE_CURVE('',#6938,#6939,#4623,.T.);
#8811=EDGE_CURVE('',#6939,#6937,#3809,.T.);
#8812=EDGE_CURVE('',#6940,#6890,#4624,.T.);
#8813=EDGE_CURVE('',#6940,#6941,#4625,.T.);
#8814=EDGE_CURVE('',#6891,#6941,#4626,.T.);
#8815=EDGE_CURVE('',#6892,#6942,#4627,.T.);
#8816=EDGE_CURVE('',#6941,#6942,#4628,.T.);
#8817=EDGE_CURVE('',#6942,#6940,#3810,.T.);
#8818=EDGE_CURVE('',#6943,#6893,#4629,.T.);
#8819=EDGE_CURVE('',#6943,#6944,#4630,.T.);
#8820=EDGE_CURVE('',#6894,#6944,#4631,.T.);
#8821=EDGE_CURVE('',#6895,#6945,#4632,.T.);
#8822=EDGE_CURVE('',#6944,#6945,#4633,.T.);
#8823=EDGE_CURVE('',#6945,#6943,#3811,.T.);
#8824=EDGE_CURVE('',#6946,#6896,#4634,.T.);
#8825=EDGE_CURVE('',#6946,#6947,#4635,.T.);
#8826=EDGE_CURVE('',#6792,#6947,#4636,.T.);
#8827=EDGE_CURVE('',#6793,#6948,#4637,.T.);
#8828=EDGE_CURVE('',#6947,#6948,#4638,.T.);
#8829=EDGE_CURVE('',#6948,#6949,#3812,.T.);
#8830=EDGE_CURVE('',#6949,#6946,#3813,.T.);
#8831=EDGE_CURVE('',#6950,#6794,#4639,.T.);
#8832=EDGE_CURVE('',#6950,#6951,#4640,.T.);
#8833=EDGE_CURVE('',#6795,#6951,#4641,.T.);
#8834=EDGE_CURVE('',#6796,#6952,#4642,.T.);
#8835=EDGE_CURVE('',#6951,#6952,#4643,.T.);
#8836=EDGE_CURVE('',#6952,#6950,#3814,.T.);
#8837=EDGE_CURVE('',#6953,#6797,#4644,.T.);
#8838=EDGE_CURVE('',#6953,#6954,#4645,.T.);
#8839=EDGE_CURVE('',#6798,#6954,#4646,.T.);
#8840=EDGE_CURVE('',#6799,#6955,#4647,.T.);
#8841=EDGE_CURVE('',#6954,#6955,#4648,.T.);
#8842=EDGE_CURVE('',#6955,#6953,#3815,.T.);
#8843=EDGE_CURVE('',#6956,#6800,#4649,.T.);
#8844=EDGE_CURVE('',#6956,#6957,#4650,.T.);
#8845=EDGE_CURVE('',#6801,#6957,#4651,.T.);
#8846=EDGE_CURVE('',#6802,#6958,#4652,.T.);
#8847=EDGE_CURVE('',#6957,#6958,#4653,.T.);
#8848=EDGE_CURVE('',#6958,#6956,#3816,.T.);
#8849=EDGE_CURVE('',#6959,#6803,#4654,.T.);
#8850=EDGE_CURVE('',#6959,#6960,#4655,.T.);
#8851=EDGE_CURVE('',#6804,#6960,#4656,.T.);
#8852=EDGE_CURVE('',#6805,#6961,#4657,.T.);
#8853=EDGE_CURVE('',#6960,#6961,#4658,.T.);
#8854=EDGE_CURVE('',#6961,#6959,#3817,.T.);
#8855=EDGE_CURVE('',#6962,#6806,#4659,.T.);
#8856=EDGE_CURVE('',#6962,#6963,#4660,.T.);
#8857=EDGE_CURVE('',#6807,#6963,#4661,.T.);
#8858=EDGE_CURVE('',#6808,#6964,#4662,.T.);
#8859=EDGE_CURVE('',#6963,#6964,#4663,.T.);
#8860=EDGE_CURVE('',#6964,#6962,#3818,.T.);
#8861=EDGE_CURVE('',#6965,#6809,#4664,.T.);
#8862=EDGE_CURVE('',#6965,#6966,#4665,.T.);
#8863=EDGE_CURVE('',#6810,#6966,#4666,.T.);
#8864=EDGE_CURVE('',#6811,#6967,#4667,.T.);
#8865=EDGE_CURVE('',#6966,#6967,#4668,.T.);
#8866=EDGE_CURVE('',#6967,#6965,#3819,.T.);
#8867=EDGE_CURVE('',#6968,#6812,#4669,.T.);
#8868=EDGE_CURVE('',#6968,#6969,#4670,.T.);
#8869=EDGE_CURVE('',#6813,#6969,#4671,.T.);
#8870=EDGE_CURVE('',#6814,#6970,#4672,.T.);
#8871=EDGE_CURVE('',#6969,#6970,#4673,.T.);
#8872=EDGE_CURVE('',#6970,#6968,#3820,.T.);
#8873=EDGE_CURVE('',#6971,#6815,#4674,.T.);
#8874=EDGE_CURVE('',#6971,#6972,#4675,.T.);
#8875=EDGE_CURVE('',#6816,#6972,#4676,.T.);
#8876=EDGE_CURVE('',#6817,#6973,#4677,.T.);
#8877=EDGE_CURVE('',#6972,#6973,#4678,.T.);
#8878=EDGE_CURVE('',#6973,#6971,#3821,.T.);
#8879=EDGE_CURVE('',#6974,#6818,#4679,.T.);
#8880=EDGE_CURVE('',#6974,#6975,#4680,.T.);
#8881=EDGE_CURVE('',#6819,#6975,#4681,.T.);
#8882=EDGE_CURVE('',#6820,#6976,#4682,.T.);
#8883=EDGE_CURVE('',#6975,#6976,#4683,.T.);
#8884=EDGE_CURVE('',#6976,#6974,#3822,.T.);
#8885=EDGE_CURVE('',#6977,#6821,#4684,.T.);
#8886=EDGE_CURVE('',#6977,#6978,#4685,.T.);
#8887=EDGE_CURVE('',#6822,#6978,#4686,.T.);
#8888=EDGE_CURVE('',#6823,#6979,#4687,.T.);
#8889=EDGE_CURVE('',#6978,#6979,#4688,.T.);
#8890=EDGE_CURVE('',#6979,#6977,#3823,.T.);
#8891=EDGE_CURVE('',#6980,#6824,#4689,.T.);
#8892=EDGE_CURVE('',#6980,#6981,#4690,.T.);
#8893=EDGE_CURVE('',#6825,#6981,#4691,.T.);
#8894=EDGE_CURVE('',#6826,#6982,#4692,.T.);
#8895=EDGE_CURVE('',#6981,#6982,#4693,.T.);
#8896=EDGE_CURVE('',#6982,#6980,#3824,.T.);
#8897=EDGE_CURVE('',#6983,#6827,#4694,.T.);
#8898=EDGE_CURVE('',#6983,#6984,#4695,.T.);
#8899=EDGE_CURVE('',#6828,#6984,#4696,.T.);
#8900=EDGE_CURVE('',#6829,#6985,#4697,.T.);
#8901=EDGE_CURVE('',#6984,#6985,#4698,.T.);
#8902=EDGE_CURVE('',#6985,#6983,#3825,.T.);
#8903=EDGE_CURVE('',#6986,#6830,#4699,.T.);
#8904=EDGE_CURVE('',#6986,#6987,#4700,.T.);
#8905=EDGE_CURVE('',#6831,#6987,#4701,.T.);
#8906=EDGE_CURVE('',#6832,#6988,#4702,.T.);
#8907=EDGE_CURVE('',#6987,#6988,#4703,.T.);
#8908=EDGE_CURVE('',#6988,#6986,#3826,.T.);
#8909=EDGE_CURVE('',#6989,#6833,#4704,.T.);
#8910=EDGE_CURVE('',#6989,#6990,#4705,.T.);
#8911=EDGE_CURVE('',#6834,#6990,#4706,.T.);
#8912=EDGE_CURVE('',#6835,#6991,#4707,.T.);
#8913=EDGE_CURVE('',#6990,#6991,#4708,.T.);
#8914=EDGE_CURVE('',#6991,#6989,#3827,.T.);
#8915=EDGE_CURVE('',#6992,#6836,#4709,.T.);
#8916=EDGE_CURVE('',#6992,#6993,#4710,.T.);
#8917=EDGE_CURVE('',#6837,#6993,#4711,.T.);
#8918=EDGE_CURVE('',#6838,#6994,#4712,.T.);
#8919=EDGE_CURVE('',#6993,#6994,#4713,.T.);
#8920=EDGE_CURVE('',#6994,#6992,#3828,.T.);
#8921=EDGE_CURVE('',#6995,#6839,#4714,.T.);
#8922=EDGE_CURVE('',#6995,#6996,#4715,.T.);
#8923=EDGE_CURVE('',#6840,#6996,#4716,.T.);
#8924=EDGE_CURVE('',#6841,#6997,#4717,.T.);
#8925=EDGE_CURVE('',#6996,#6997,#4718,.T.);
#8926=EDGE_CURVE('',#6997,#6995,#3829,.T.);
#8927=EDGE_CURVE('',#6998,#6842,#4719,.T.);
#8928=EDGE_CURVE('',#6998,#6999,#4720,.T.);
#8929=EDGE_CURVE('',#6843,#6999,#4721,.T.);
#8930=EDGE_CURVE('',#6844,#7000,#4722,.T.);
#8931=EDGE_CURVE('',#6999,#7000,#4723,.T.);
#8932=EDGE_CURVE('',#7000,#6998,#3830,.T.);
#8933=EDGE_CURVE('',#7001,#6845,#4724,.T.);
#8934=EDGE_CURVE('',#7001,#7002,#4725,.T.);
#8935=EDGE_CURVE('',#6846,#7002,#4726,.T.);
#8936=EDGE_CURVE('',#6847,#7003,#4727,.T.);
#8937=EDGE_CURVE('',#7002,#7003,#4728,.T.);
#8938=EDGE_CURVE('',#7003,#7001,#3831,.T.);
#8939=EDGE_CURVE('',#6949,#6784,#4729,.T.);
#8940=EDGE_CURVE('',#7004,#7005,#4730,.T.);
#8941=EDGE_CURVE('',#7005,#7006,#4731,.T.);
#8942=EDGE_CURVE('',#7006,#7007,#4732,.T.);
#8943=EDGE_CURVE('',#7007,#7008,#4733,.T.);
#8944=EDGE_CURVE('',#7008,#7009,#4734,.T.);
#8945=EDGE_CURVE('',#7009,#7004,#4735,.T.);
#8946=EDGE_CURVE('',#7010,#7011,#4736,.T.);
#8947=EDGE_CURVE('',#7010,#7011,#3832,.T.);
#8948=EDGE_CURVE('',#7011,#7012,#4737,.T.);
#8949=EDGE_CURVE('',#7011,#7012,#3833,.T.);
#8950=EDGE_CURVE('',#7012,#7013,#4738,.T.);
#8951=EDGE_CURVE('',#7012,#7013,#3834,.T.);
#8952=EDGE_CURVE('',#7013,#7014,#4739,.T.);
#8953=EDGE_CURVE('',#7013,#7014,#3835,.T.);
#8954=EDGE_CURVE('',#7014,#7015,#4740,.T.);
#8955=EDGE_CURVE('',#7014,#7015,#3836,.T.);
#8956=EDGE_CURVE('',#7015,#7010,#4741,.T.);
#8957=EDGE_CURVE('',#7015,#7010,#3837,.T.);
#8958=EDGE_CURVE('',#7016,#7010,#4742,.T.);
#8959=EDGE_CURVE('',#7004,#7010,#4743,.T.);
#8960=EDGE_CURVE('',#7005,#7011,#4744,.T.);
#8961=EDGE_CURVE('',#7009,#7015,#4745,.T.);
#8962=EDGE_CURVE('',#7008,#7014,#4746,.T.);
#8963=EDGE_CURVE('',#7007,#7013,#4747,.T.);
#8964=EDGE_CURVE('',#7006,#7012,#4748,.T.);
#11931=ORIENTED_EDGE('',*,*,#8500,.F.);
#11932=ORIENTED_EDGE('',*,*,#8501,.F.);
#11933=ORIENTED_EDGE('',*,*,#8502,.F.);
#11934=ORIENTED_EDGE('',*,*,#8503,.T.);
#11935=ORIENTED_EDGE('',*,*,#8504,.F.);
#11936=ORIENTED_EDGE('',*,*,#8505,.F.);
#11937=ORIENTED_EDGE('',*,*,#8506,.F.);
#11938=ORIENTED_EDGE('',*,*,#8500,.T.);
#11939=ORIENTED_EDGE('',*,*,#8507,.T.);
#11940=ORIENTED_EDGE('',*,*,#8508,.T.);
#11941=ORIENTED_EDGE('',*,*,#8509,.F.);
#11942=ORIENTED_EDGE('',*,*,#8510,.F.);
#11943=ORIENTED_EDGE('',*,*,#8504,.T.);
#11944=ORIENTED_EDGE('',*,*,#8511,.T.);
#11945=ORIENTED_EDGE('',*,*,#8512,.T.);
#11946=ORIENTED_EDGE('',*,*,#8513,.F.);
#11947=ORIENTED_EDGE('',*,*,#8514,.F.);
#11948=ORIENTED_EDGE('',*,*,#8515,.F.);
#11949=ORIENTED_EDGE('',*,*,#8509,.T.);
#11950=ORIENTED_EDGE('',*,*,#8516,.T.);
#11951=ORIENTED_EDGE('',*,*,#8517,.T.);
#11952=ORIENTED_EDGE('',*,*,#8518,.F.);
#11953=ORIENTED_EDGE('',*,*,#8519,.F.);
#11954=ORIENTED_EDGE('',*,*,#8520,.F.);
#11955=ORIENTED_EDGE('',*,*,#8513,.T.);
#11956=ORIENTED_EDGE('',*,*,#8521,.T.);
#11957=ORIENTED_EDGE('',*,*,#8522,.F.);
#11958=ORIENTED_EDGE('',*,*,#8523,.F.);
#11959=ORIENTED_EDGE('',*,*,#8518,.T.);
#11960=ORIENTED_EDGE('',*,*,#8524,.T.);
#11961=ORIENTED_EDGE('',*,*,#8525,.T.);
#11962=ORIENTED_EDGE('',*,*,#8526,.F.);
#11963=ORIENTED_EDGE('',*,*,#8527,.F.);
#11964=ORIENTED_EDGE('',*,*,#8528,.F.);
#11965=ORIENTED_EDGE('',*,*,#8522,.T.);
#11966=ORIENTED_EDGE('',*,*,#8529,.T.);
#11967=ORIENTED_EDGE('',*,*,#8530,.F.);
#11968=ORIENTED_EDGE('',*,*,#8531,.F.);
#11969=ORIENTED_EDGE('',*,*,#8526,.T.);
#11970=ORIENTED_EDGE('',*,*,#8532,.T.);
#11971=ORIENTED_EDGE('',*,*,#8533,.T.);
#11972=ORIENTED_EDGE('',*,*,#8534,.F.);
#11973=ORIENTED_EDGE('',*,*,#8535,.F.);
#11974=ORIENTED_EDGE('',*,*,#8536,.F.);
#11975=ORIENTED_EDGE('',*,*,#8530,.T.);
#11976=ORIENTED_EDGE('',*,*,#8537,.T.);
#11977=ORIENTED_EDGE('',*,*,#8538,.F.);
#11978=ORIENTED_EDGE('',*,*,#8539,.F.);
#11979=ORIENTED_EDGE('',*,*,#8534,.T.);
#11980=ORIENTED_EDGE('',*,*,#8540,.T.);
#11981=ORIENTED_EDGE('',*,*,#8541,.T.);
#11982=ORIENTED_EDGE('',*,*,#8542,.F.);
#11983=ORIENTED_EDGE('',*,*,#8543,.F.);
#11984=ORIENTED_EDGE('',*,*,#8544,.F.);
#11985=ORIENTED_EDGE('',*,*,#8538,.T.);
#11986=ORIENTED_EDGE('',*,*,#8545,.T.);
#11987=ORIENTED_EDGE('',*,*,#8546,.T.);
#11988=ORIENTED_EDGE('',*,*,#8547,.F.);
#11989=ORIENTED_EDGE('',*,*,#8548,.F.);
#11990=ORIENTED_EDGE('',*,*,#8549,.F.);
#11991=ORIENTED_EDGE('',*,*,#8542,.T.);
#11992=ORIENTED_EDGE('',*,*,#8550,.T.);
#11993=ORIENTED_EDGE('',*,*,#8551,.F.);
#11994=ORIENTED_EDGE('',*,*,#8552,.F.);
#11995=ORIENTED_EDGE('',*,*,#8553,.F.);
#11996=ORIENTED_EDGE('',*,*,#8547,.T.);
#11997=ORIENTED_EDGE('',*,*,#8554,.T.);
#11998=ORIENTED_EDGE('',*,*,#8555,.F.);
#11999=ORIENTED_EDGE('',*,*,#8556,.F.);
#12000=ORIENTED_EDGE('',*,*,#8551,.T.);
#12001=ORIENTED_EDGE('',*,*,#8557,.T.);
#12002=ORIENTED_EDGE('',*,*,#8558,.T.);
#12003=ORIENTED_EDGE('',*,*,#8559,.F.);
#12004=ORIENTED_EDGE('',*,*,#8560,.T.);
#12005=ORIENTED_EDGE('',*,*,#8561,.T.);
#12006=ORIENTED_EDGE('',*,*,#8562,.T.);
#12007=ORIENTED_EDGE('',*,*,#8563,.T.);
#12008=ORIENTED_EDGE('',*,*,#8564,.T.);
#12009=ORIENTED_EDGE('',*,*,#8565,.T.);
#12010=ORIENTED_EDGE('',*,*,#8566,.T.);
#12011=ORIENTED_EDGE('',*,*,#8567,.T.);
#12012=ORIENTED_EDGE('',*,*,#8568,.T.);
#12013=ORIENTED_EDGE('',*,*,#8569,.T.);
#12014=ORIENTED_EDGE('',*,*,#8570,.T.);
#12015=ORIENTED_EDGE('',*,*,#8571,.T.);
#12016=ORIENTED_EDGE('',*,*,#8572,.T.);
#12017=ORIENTED_EDGE('',*,*,#8573,.T.);
#12018=ORIENTED_EDGE('',*,*,#8574,.T.);
#12019=ORIENTED_EDGE('',*,*,#8575,.T.);
#12020=ORIENTED_EDGE('',*,*,#8576,.F.);
#12021=ORIENTED_EDGE('',*,*,#8577,.T.);
#12022=ORIENTED_EDGE('',*,*,#8578,.T.);
#12023=ORIENTED_EDGE('',*,*,#8579,.T.);
#12024=ORIENTED_EDGE('',*,*,#8580,.T.);
#12025=ORIENTED_EDGE('',*,*,#8581,.T.);
#12026=ORIENTED_EDGE('',*,*,#8582,.T.);
#12027=ORIENTED_EDGE('',*,*,#8583,.T.);
#12028=ORIENTED_EDGE('',*,*,#8584,.T.);
#12029=ORIENTED_EDGE('',*,*,#8585,.T.);
#12030=ORIENTED_EDGE('',*,*,#8586,.T.);
#12031=ORIENTED_EDGE('',*,*,#8587,.T.);
#12032=ORIENTED_EDGE('',*,*,#8588,.T.);
#12033=ORIENTED_EDGE('',*,*,#8589,.T.);
#12034=ORIENTED_EDGE('',*,*,#8590,.T.);
#12035=ORIENTED_EDGE('',*,*,#8591,.T.);
#12036=ORIENTED_EDGE('',*,*,#8555,.T.);
#12037=ORIENTED_EDGE('',*,*,#8592,.T.);
#12038=ORIENTED_EDGE('',*,*,#8593,.F.);
#12039=ORIENTED_EDGE('',*,*,#8594,.F.);
#12040=ORIENTED_EDGE('',*,*,#8595,.F.);
#12041=ORIENTED_EDGE('',*,*,#8596,.F.);
#12042=ORIENTED_EDGE('',*,*,#8597,.T.);
#12043=ORIENTED_EDGE('',*,*,#8593,.T.);
#12044=ORIENTED_EDGE('',*,*,#8598,.T.);
#12045=ORIENTED_EDGE('',*,*,#8599,.T.);
#12046=ORIENTED_EDGE('',*,*,#8600,.F.);
#12047=ORIENTED_EDGE('',*,*,#8597,.F.);
#12048=ORIENTED_EDGE('',*,*,#8601,.F.);
#12049=ORIENTED_EDGE('',*,*,#8575,.F.);
#12050=ORIENTED_EDGE('',*,*,#8574,.F.);
#12051=ORIENTED_EDGE('',*,*,#8573,.F.);
#12052=ORIENTED_EDGE('',*,*,#8572,.F.);
#12053=ORIENTED_EDGE('',*,*,#8571,.F.);
#12054=ORIENTED_EDGE('',*,*,#8570,.F.);
#12055=ORIENTED_EDGE('',*,*,#8569,.F.);
#12056=ORIENTED_EDGE('',*,*,#8568,.F.);
#12057=ORIENTED_EDGE('',*,*,#8567,.F.);
#12058=ORIENTED_EDGE('',*,*,#8566,.F.);
#12059=ORIENTED_EDGE('',*,*,#8565,.F.);
#12060=ORIENTED_EDGE('',*,*,#8564,.F.);
#12061=ORIENTED_EDGE('',*,*,#8563,.F.);
#12062=ORIENTED_EDGE('',*,*,#8562,.F.);
#12063=ORIENTED_EDGE('',*,*,#8561,.F.);
#12064=ORIENTED_EDGE('',*,*,#8560,.F.);
#12065=ORIENTED_EDGE('',*,*,#8602,.F.);
#12066=ORIENTED_EDGE('',*,*,#8501,.T.);
#12067=ORIENTED_EDGE('',*,*,#8506,.T.);
#12068=ORIENTED_EDGE('',*,*,#8505,.T.);
#12069=ORIENTED_EDGE('',*,*,#8510,.T.);
#12070=ORIENTED_EDGE('',*,*,#8515,.T.);
#12071=ORIENTED_EDGE('',*,*,#8514,.T.);
#12072=ORIENTED_EDGE('',*,*,#8520,.T.);
#12073=ORIENTED_EDGE('',*,*,#8519,.T.);
#12074=ORIENTED_EDGE('',*,*,#8523,.T.);
#12075=ORIENTED_EDGE('',*,*,#8528,.T.);
#12076=ORIENTED_EDGE('',*,*,#8527,.T.);
#12077=ORIENTED_EDGE('',*,*,#8531,.T.);
#12078=ORIENTED_EDGE('',*,*,#8536,.T.);
#12079=ORIENTED_EDGE('',*,*,#8535,.T.);
#12080=ORIENTED_EDGE('',*,*,#8539,.T.);
#12081=ORIENTED_EDGE('',*,*,#8544,.T.);
#12082=ORIENTED_EDGE('',*,*,#8543,.T.);
#12083=ORIENTED_EDGE('',*,*,#8549,.T.);
#12084=ORIENTED_EDGE('',*,*,#8548,.T.);
#12085=ORIENTED_EDGE('',*,*,#8553,.T.);
#12086=ORIENTED_EDGE('',*,*,#8552,.T.);
#12087=ORIENTED_EDGE('',*,*,#8556,.T.);
#12088=ORIENTED_EDGE('',*,*,#8595,.T.);
#12089=ORIENTED_EDGE('',*,*,#8594,.T.);
#12090=ORIENTED_EDGE('',*,*,#8603,.F.);
#12091=ORIENTED_EDGE('',*,*,#8604,.T.);
#12092=ORIENTED_EDGE('',*,*,#8502,.T.);
#12093=ORIENTED_EDGE('',*,*,#8602,.T.);
#12094=ORIENTED_EDGE('',*,*,#8605,.F.);
#12095=ORIENTED_EDGE('',*,*,#8599,.F.);
#12096=ORIENTED_EDGE('',*,*,#8598,.F.);
#12097=ORIENTED_EDGE('',*,*,#8592,.F.);
#12098=ORIENTED_EDGE('',*,*,#8557,.F.);
#12099=ORIENTED_EDGE('',*,*,#8554,.F.);
#12100=ORIENTED_EDGE('',*,*,#8550,.F.);
#12101=ORIENTED_EDGE('',*,*,#8546,.F.);
#12102=ORIENTED_EDGE('',*,*,#8545,.F.);
#12103=ORIENTED_EDGE('',*,*,#8541,.F.);
#12104=ORIENTED_EDGE('',*,*,#8540,.F.);
#12105=ORIENTED_EDGE('',*,*,#8537,.F.);
#12106=ORIENTED_EDGE('',*,*,#8533,.F.);
#12107=ORIENTED_EDGE('',*,*,#8532,.F.);
#12108=ORIENTED_EDGE('',*,*,#8529,.F.);
#12109=ORIENTED_EDGE('',*,*,#8525,.F.);
#12110=ORIENTED_EDGE('',*,*,#8524,.F.);
#12111=ORIENTED_EDGE('',*,*,#8521,.F.);
#12112=ORIENTED_EDGE('',*,*,#8517,.F.);
#12113=ORIENTED_EDGE('',*,*,#8516,.F.);
#12114=ORIENTED_EDGE('',*,*,#8512,.F.);
#12115=ORIENTED_EDGE('',*,*,#8511,.F.);
#12116=ORIENTED_EDGE('',*,*,#8508,.F.);
#12117=ORIENTED_EDGE('',*,*,#8507,.F.);
#12118=ORIENTED_EDGE('',*,*,#8503,.F.);
#12119=ORIENTED_EDGE('',*,*,#8604,.F.);
#12120=ORIENTED_EDGE('',*,*,#8606,.F.);
#12121=ORIENTED_EDGE('',*,*,#8558,.F.);
#12122=ORIENTED_EDGE('',*,*,#8591,.F.);
#12123=ORIENTED_EDGE('',*,*,#8590,.F.);
#12124=ORIENTED_EDGE('',*,*,#8589,.F.);
#12125=ORIENTED_EDGE('',*,*,#8588,.F.);
#12126=ORIENTED_EDGE('',*,*,#8587,.F.);
#12127=ORIENTED_EDGE('',*,*,#8586,.F.);
#12128=ORIENTED_EDGE('',*,*,#8585,.F.);
#12129=ORIENTED_EDGE('',*,*,#8584,.F.);
#12130=ORIENTED_EDGE('',*,*,#8583,.F.);
#12131=ORIENTED_EDGE('',*,*,#8582,.F.);
#12132=ORIENTED_EDGE('',*,*,#8581,.F.);
#12133=ORIENTED_EDGE('',*,*,#8580,.F.);
#12134=ORIENTED_EDGE('',*,*,#8579,.F.);
#12135=ORIENTED_EDGE('',*,*,#8578,.F.);
#12136=ORIENTED_EDGE('',*,*,#8577,.F.);
#12137=ORIENTED_EDGE('',*,*,#8607,.T.);
#12138=ORIENTED_EDGE('',*,*,#8608,.T.);
#12139=ORIENTED_EDGE('',*,*,#8605,.T.);
#12140=ORIENTED_EDGE('',*,*,#8559,.T.);
#12141=ORIENTED_EDGE('',*,*,#8606,.T.);
#12142=ORIENTED_EDGE('',*,*,#8603,.T.);
#12143=ORIENTED_EDGE('',*,*,#8608,.F.);
#12144=ORIENTED_EDGE('',*,*,#8609,.F.);
#12145=ORIENTED_EDGE('',*,*,#8607,.F.);
#12146=ORIENTED_EDGE('',*,*,#8596,.T.);
#12147=ORIENTED_EDGE('',*,*,#8610,.T.);
#12148=ORIENTED_EDGE('',*,*,#8611,.T.);
#12149=ORIENTED_EDGE('',*,*,#8610,.F.);
#12150=ORIENTED_EDGE('',*,*,#8600,.T.);
#12151=ORIENTED_EDGE('',*,*,#8576,.T.);
#12152=ORIENTED_EDGE('',*,*,#8601,.T.);
#12153=ORIENTED_EDGE('',*,*,#8611,.F.);
#12154=ORIENTED_EDGE('',*,*,#8612,.F.);
#12155=ORIENTED_EDGE('',*,*,#8613,.T.);
#12156=ORIENTED_EDGE('',*,*,#8614,.F.);
#12157=ORIENTED_EDGE('',*,*,#8615,.F.);
#12158=ORIENTED_EDGE('',*,*,#8616,.F.);
#12159=ORIENTED_EDGE('',*,*,#8617,.F.);
#12160=ORIENTED_EDGE('',*,*,#8614,.T.);
#12161=ORIENTED_EDGE('',*,*,#8618,.T.);
#12162=ORIENTED_EDGE('',*,*,#8619,.F.);
#12163=ORIENTED_EDGE('',*,*,#8618,.F.);
#12164=ORIENTED_EDGE('',*,*,#8613,.F.);
#12165=ORIENTED_EDGE('',*,*,#8620,.T.);
#12166=ORIENTED_EDGE('',*,*,#8621,.T.);
#12167=ORIENTED_EDGE('',*,*,#8622,.T.);
#12168=ORIENTED_EDGE('',*,*,#8623,.T.);
#12169=ORIENTED_EDGE('',*,*,#8624,.T.);
#12170=ORIENTED_EDGE('',*,*,#8625,.T.);
#12171=ORIENTED_EDGE('',*,*,#8626,.T.);
#12172=ORIENTED_EDGE('',*,*,#8627,.T.);
#12173=ORIENTED_EDGE('',*,*,#8628,.T.);
#12174=ORIENTED_EDGE('',*,*,#8629,.T.);
#12175=ORIENTED_EDGE('',*,*,#8630,.T.);
#12176=ORIENTED_EDGE('',*,*,#8631,.T.);
#12177=ORIENTED_EDGE('',*,*,#8632,.T.);
#12178=ORIENTED_EDGE('',*,*,#8633,.T.);
#12179=ORIENTED_EDGE('',*,*,#8634,.T.);
#12180=ORIENTED_EDGE('',*,*,#8635,.T.);
#12181=ORIENTED_EDGE('',*,*,#8636,.T.);
#12182=ORIENTED_EDGE('',*,*,#8637,.T.);
#12183=ORIENTED_EDGE('',*,*,#8638,.T.);
#12184=ORIENTED_EDGE('',*,*,#8639,.T.);
#12185=ORIENTED_EDGE('',*,*,#8640,.T.);
#12186=ORIENTED_EDGE('',*,*,#8641,.T.);
#12187=ORIENTED_EDGE('',*,*,#8642,.T.);
#12188=ORIENTED_EDGE('',*,*,#8643,.T.);
#12189=ORIENTED_EDGE('',*,*,#8644,.T.);
#12190=ORIENTED_EDGE('',*,*,#8645,.T.);
#12191=ORIENTED_EDGE('',*,*,#8646,.T.);
#12192=ORIENTED_EDGE('',*,*,#8647,.T.);
#12193=ORIENTED_EDGE('',*,*,#8648,.T.);
#12194=ORIENTED_EDGE('',*,*,#8649,.T.);
#12195=ORIENTED_EDGE('',*,*,#8650,.T.);
#12196=ORIENTED_EDGE('',*,*,#8651,.T.);
#12197=ORIENTED_EDGE('',*,*,#8652,.T.);
#12198=ORIENTED_EDGE('',*,*,#8653,.T.);
#12199=ORIENTED_EDGE('',*,*,#8654,.T.);
#12200=ORIENTED_EDGE('',*,*,#8655,.T.);
#12201=ORIENTED_EDGE('',*,*,#8656,.T.);
#12202=ORIENTED_EDGE('',*,*,#8657,.T.);
#12203=ORIENTED_EDGE('',*,*,#8658,.T.);
#12204=ORIENTED_EDGE('',*,*,#8659,.T.);
#12205=ORIENTED_EDGE('',*,*,#8660,.T.);
#12206=ORIENTED_EDGE('',*,*,#8661,.T.);
#12207=ORIENTED_EDGE('',*,*,#8662,.T.);
#12208=ORIENTED_EDGE('',*,*,#8663,.T.);
#12209=ORIENTED_EDGE('',*,*,#8664,.T.);
#12210=ORIENTED_EDGE('',*,*,#8665,.T.);
#12211=ORIENTED_EDGE('',*,*,#8666,.T.);
#12212=ORIENTED_EDGE('',*,*,#8667,.T.);
#12213=ORIENTED_EDGE('',*,*,#8668,.T.);
#12214=ORIENTED_EDGE('',*,*,#8669,.T.);
#12215=ORIENTED_EDGE('',*,*,#8670,.T.);
#12216=ORIENTED_EDGE('',*,*,#8671,.T.);
#12217=ORIENTED_EDGE('',*,*,#8672,.T.);
#12218=ORIENTED_EDGE('',*,*,#8673,.T.);
#12219=ORIENTED_EDGE('',*,*,#8674,.T.);
#12220=ORIENTED_EDGE('',*,*,#8675,.T.);
#12221=ORIENTED_EDGE('',*,*,#8615,.T.);
#12222=ORIENTED_EDGE('',*,*,#8617,.T.);
#12223=ORIENTED_EDGE('',*,*,#8676,.T.);
#12224=ORIENTED_EDGE('',*,*,#8677,.T.);
#12225=ORIENTED_EDGE('',*,*,#8678,.T.);
#12226=ORIENTED_EDGE('',*,*,#8679,.T.);
#12227=ORIENTED_EDGE('',*,*,#8680,.T.);
#12228=ORIENTED_EDGE('',*,*,#8681,.T.);
#12229=ORIENTED_EDGE('',*,*,#8682,.T.);
#12230=ORIENTED_EDGE('',*,*,#8683,.T.);
#12231=ORIENTED_EDGE('',*,*,#8684,.T.);
#12232=ORIENTED_EDGE('',*,*,#8685,.T.);
#12233=ORIENTED_EDGE('',*,*,#8686,.T.);
#12234=ORIENTED_EDGE('',*,*,#8687,.T.);
#12235=ORIENTED_EDGE('',*,*,#8688,.T.);
#12236=ORIENTED_EDGE('',*,*,#8689,.T.);
#12237=ORIENTED_EDGE('',*,*,#8690,.T.);
#12238=ORIENTED_EDGE('',*,*,#8691,.T.);
#12239=ORIENTED_EDGE('',*,*,#8692,.T.);
#12240=ORIENTED_EDGE('',*,*,#8693,.T.);
#12241=ORIENTED_EDGE('',*,*,#8694,.T.);
#12242=ORIENTED_EDGE('',*,*,#8695,.T.);
#12243=ORIENTED_EDGE('',*,*,#8696,.T.);
#12244=ORIENTED_EDGE('',*,*,#8697,.T.);
#12245=ORIENTED_EDGE('',*,*,#8698,.T.);
#12246=ORIENTED_EDGE('',*,*,#8699,.T.);
#12247=ORIENTED_EDGE('',*,*,#8700,.T.);
#12248=ORIENTED_EDGE('',*,*,#8701,.T.);
#12249=ORIENTED_EDGE('',*,*,#8702,.T.);
#12250=ORIENTED_EDGE('',*,*,#8703,.T.);
#12251=ORIENTED_EDGE('',*,*,#8704,.T.);
#12252=ORIENTED_EDGE('',*,*,#8705,.T.);
#12253=ORIENTED_EDGE('',*,*,#8706,.T.);
#12254=ORIENTED_EDGE('',*,*,#8707,.T.);
#12255=ORIENTED_EDGE('',*,*,#8708,.T.);
#12256=ORIENTED_EDGE('',*,*,#8709,.T.);
#12257=ORIENTED_EDGE('',*,*,#8710,.T.);
#12258=ORIENTED_EDGE('',*,*,#8711,.T.);
#12259=ORIENTED_EDGE('',*,*,#8712,.T.);
#12260=ORIENTED_EDGE('',*,*,#8713,.T.);
#12261=ORIENTED_EDGE('',*,*,#8714,.T.);
#12262=ORIENTED_EDGE('',*,*,#8715,.T.);
#12263=ORIENTED_EDGE('',*,*,#8716,.T.);
#12264=ORIENTED_EDGE('',*,*,#8717,.T.);
#12265=ORIENTED_EDGE('',*,*,#8718,.T.);
#12266=ORIENTED_EDGE('',*,*,#8719,.T.);
#12267=ORIENTED_EDGE('',*,*,#8720,.T.);
#12268=ORIENTED_EDGE('',*,*,#8721,.T.);
#12269=ORIENTED_EDGE('',*,*,#8722,.T.);
#12270=ORIENTED_EDGE('',*,*,#8723,.T.);
#12271=ORIENTED_EDGE('',*,*,#8724,.T.);
#12272=ORIENTED_EDGE('',*,*,#8725,.T.);
#12273=ORIENTED_EDGE('',*,*,#8726,.T.);
#12274=ORIENTED_EDGE('',*,*,#8727,.T.);
#12275=ORIENTED_EDGE('',*,*,#8726,.F.);
#12276=ORIENTED_EDGE('',*,*,#8728,.F.);
#12277=ORIENTED_EDGE('',*,*,#8729,.T.);
#12278=ORIENTED_EDGE('',*,*,#8730,.F.);
#12279=ORIENTED_EDGE('',*,*,#8677,.F.);
#12280=ORIENTED_EDGE('',*,*,#8731,.F.);
#12281=ORIENTED_EDGE('',*,*,#8678,.F.);
#12282=ORIENTED_EDGE('',*,*,#8730,.T.);
#12283=ORIENTED_EDGE('',*,*,#8732,.T.);
#12284=ORIENTED_EDGE('',*,*,#8733,.F.);
#12285=ORIENTED_EDGE('',*,*,#8732,.F.);
#12286=ORIENTED_EDGE('',*,*,#8729,.F.);
#12287=ORIENTED_EDGE('',*,*,#8734,.F.);
#12288=ORIENTED_EDGE('',*,*,#8735,.T.);
#12289=ORIENTED_EDGE('',*,*,#8736,.F.);
#12290=ORIENTED_EDGE('',*,*,#8680,.F.);
#12291=ORIENTED_EDGE('',*,*,#8737,.F.);
#12292=ORIENTED_EDGE('',*,*,#8681,.F.);
#12293=ORIENTED_EDGE('',*,*,#8736,.T.);
#12294=ORIENTED_EDGE('',*,*,#8738,.T.);
#12295=ORIENTED_EDGE('',*,*,#8739,.F.);
#12296=ORIENTED_EDGE('',*,*,#8738,.F.);
#12297=ORIENTED_EDGE('',*,*,#8735,.F.);
#12298=ORIENTED_EDGE('',*,*,#8740,.F.);
#12299=ORIENTED_EDGE('',*,*,#8741,.T.);
#12300=ORIENTED_EDGE('',*,*,#8742,.F.);
#12301=ORIENTED_EDGE('',*,*,#8683,.F.);
#12302=ORIENTED_EDGE('',*,*,#8743,.F.);
#12303=ORIENTED_EDGE('',*,*,#8684,.F.);
#12304=ORIENTED_EDGE('',*,*,#8742,.T.);
#12305=ORIENTED_EDGE('',*,*,#8744,.T.);
#12306=ORIENTED_EDGE('',*,*,#8745,.F.);
#12307=ORIENTED_EDGE('',*,*,#8744,.F.);
#12308=ORIENTED_EDGE('',*,*,#8741,.F.);
#12309=ORIENTED_EDGE('',*,*,#8746,.F.);
#12310=ORIENTED_EDGE('',*,*,#8747,.T.);
#12311=ORIENTED_EDGE('',*,*,#8748,.F.);
#12312=ORIENTED_EDGE('',*,*,#8686,.F.);
#12313=ORIENTED_EDGE('',*,*,#8749,.F.);
#12314=ORIENTED_EDGE('',*,*,#8687,.F.);
#12315=ORIENTED_EDGE('',*,*,#8748,.T.);
#12316=ORIENTED_EDGE('',*,*,#8750,.T.);
#12317=ORIENTED_EDGE('',*,*,#8751,.F.);
#12318=ORIENTED_EDGE('',*,*,#8750,.F.);
#12319=ORIENTED_EDGE('',*,*,#8747,.F.);
#12320=ORIENTED_EDGE('',*,*,#8752,.F.);
#12321=ORIENTED_EDGE('',*,*,#8753,.T.);
#12322=ORIENTED_EDGE('',*,*,#8754,.F.);
#12323=ORIENTED_EDGE('',*,*,#8689,.F.);
#12324=ORIENTED_EDGE('',*,*,#8755,.F.);
#12325=ORIENTED_EDGE('',*,*,#8690,.F.);
#12326=ORIENTED_EDGE('',*,*,#8754,.T.);
#12327=ORIENTED_EDGE('',*,*,#8756,.T.);
#12328=ORIENTED_EDGE('',*,*,#8757,.F.);
#12329=ORIENTED_EDGE('',*,*,#8756,.F.);
#12330=ORIENTED_EDGE('',*,*,#8753,.F.);
#12331=ORIENTED_EDGE('',*,*,#8758,.F.);
#12332=ORIENTED_EDGE('',*,*,#8759,.T.);
#12333=ORIENTED_EDGE('',*,*,#8760,.F.);
#12334=ORIENTED_EDGE('',*,*,#8692,.F.);
#12335=ORIENTED_EDGE('',*,*,#8761,.F.);
#12336=ORIENTED_EDGE('',*,*,#8693,.F.);
#12337=ORIENTED_EDGE('',*,*,#8760,.T.);
#12338=ORIENTED_EDGE('',*,*,#8762,.T.);
#12339=ORIENTED_EDGE('',*,*,#8763,.F.);
#12340=ORIENTED_EDGE('',*,*,#8762,.F.);
#12341=ORIENTED_EDGE('',*,*,#8759,.F.);
#12342=ORIENTED_EDGE('',*,*,#8764,.F.);
#12343=ORIENTED_EDGE('',*,*,#8765,.T.);
#12344=ORIENTED_EDGE('',*,*,#8766,.F.);
#12345=ORIENTED_EDGE('',*,*,#8695,.F.);
#12346=ORIENTED_EDGE('',*,*,#8767,.F.);
#12347=ORIENTED_EDGE('',*,*,#8696,.F.);
#12348=ORIENTED_EDGE('',*,*,#8766,.T.);
#12349=ORIENTED_EDGE('',*,*,#8768,.T.);
#12350=ORIENTED_EDGE('',*,*,#8769,.F.);
#12351=ORIENTED_EDGE('',*,*,#8768,.F.);
#12352=ORIENTED_EDGE('',*,*,#8765,.F.);
#12353=ORIENTED_EDGE('',*,*,#8770,.F.);
#12354=ORIENTED_EDGE('',*,*,#8771,.T.);
#12355=ORIENTED_EDGE('',*,*,#8772,.F.);
#12356=ORIENTED_EDGE('',*,*,#8698,.F.);
#12357=ORIENTED_EDGE('',*,*,#8773,.F.);
#12358=ORIENTED_EDGE('',*,*,#8699,.F.);
#12359=ORIENTED_EDGE('',*,*,#8772,.T.);
#12360=ORIENTED_EDGE('',*,*,#8774,.T.);
#12361=ORIENTED_EDGE('',*,*,#8775,.F.);
#12362=ORIENTED_EDGE('',*,*,#8774,.F.);
#12363=ORIENTED_EDGE('',*,*,#8771,.F.);
#12364=ORIENTED_EDGE('',*,*,#8776,.F.);
#12365=ORIENTED_EDGE('',*,*,#8777,.T.);
#12366=ORIENTED_EDGE('',*,*,#8778,.F.);
#12367=ORIENTED_EDGE('',*,*,#8701,.F.);
#12368=ORIENTED_EDGE('',*,*,#8779,.F.);
#12369=ORIENTED_EDGE('',*,*,#8702,.F.);
#12370=ORIENTED_EDGE('',*,*,#8778,.T.);
#12371=ORIENTED_EDGE('',*,*,#8780,.T.);
#12372=ORIENTED_EDGE('',*,*,#8781,.F.);
#12373=ORIENTED_EDGE('',*,*,#8780,.F.);
#12374=ORIENTED_EDGE('',*,*,#8777,.F.);
#12375=ORIENTED_EDGE('',*,*,#8782,.F.);
#12376=ORIENTED_EDGE('',*,*,#8783,.T.);
#12377=ORIENTED_EDGE('',*,*,#8784,.F.);
#12378=ORIENTED_EDGE('',*,*,#8704,.F.);
#12379=ORIENTED_EDGE('',*,*,#8785,.F.);
#12380=ORIENTED_EDGE('',*,*,#8705,.F.);
#12381=ORIENTED_EDGE('',*,*,#8784,.T.);
#12382=ORIENTED_EDGE('',*,*,#8786,.T.);
#12383=ORIENTED_EDGE('',*,*,#8787,.F.);
#12384=ORIENTED_EDGE('',*,*,#8786,.F.);
#12385=ORIENTED_EDGE('',*,*,#8783,.F.);
#12386=ORIENTED_EDGE('',*,*,#8788,.F.);
#12387=ORIENTED_EDGE('',*,*,#8789,.T.);
#12388=ORIENTED_EDGE('',*,*,#8790,.F.);
#12389=ORIENTED_EDGE('',*,*,#8707,.F.);
#12390=ORIENTED_EDGE('',*,*,#8791,.F.);
#12391=ORIENTED_EDGE('',*,*,#8708,.F.);
#12392=ORIENTED_EDGE('',*,*,#8790,.T.);
#12393=ORIENTED_EDGE('',*,*,#8792,.T.);
#12394=ORIENTED_EDGE('',*,*,#8793,.F.);
#12395=ORIENTED_EDGE('',*,*,#8792,.F.);
#12396=ORIENTED_EDGE('',*,*,#8789,.F.);
#12397=ORIENTED_EDGE('',*,*,#8794,.F.);
#12398=ORIENTED_EDGE('',*,*,#8795,.T.);
#12399=ORIENTED_EDGE('',*,*,#8796,.F.);
#12400=ORIENTED_EDGE('',*,*,#8710,.F.);
#12401=ORIENTED_EDGE('',*,*,#8797,.F.);
#12402=ORIENTED_EDGE('',*,*,#8711,.F.);
#12403=ORIENTED_EDGE('',*,*,#8796,.T.);
#12404=ORIENTED_EDGE('',*,*,#8798,.T.);
#12405=ORIENTED_EDGE('',*,*,#8799,.F.);
#12406=ORIENTED_EDGE('',*,*,#8798,.F.);
#12407=ORIENTED_EDGE('',*,*,#8795,.F.);
#12408=ORIENTED_EDGE('',*,*,#8800,.F.);
#12409=ORIENTED_EDGE('',*,*,#8801,.T.);
#12410=ORIENTED_EDGE('',*,*,#8802,.F.);
#12411=ORIENTED_EDGE('',*,*,#8713,.F.);
#12412=ORIENTED_EDGE('',*,*,#8803,.F.);
#12413=ORIENTED_EDGE('',*,*,#8714,.F.);
#12414=ORIENTED_EDGE('',*,*,#8802,.T.);
#12415=ORIENTED_EDGE('',*,*,#8804,.T.);
#12416=ORIENTED_EDGE('',*,*,#8805,.F.);
#12417=ORIENTED_EDGE('',*,*,#8804,.F.);
#12418=ORIENTED_EDGE('',*,*,#8801,.F.);
#12419=ORIENTED_EDGE('',*,*,#8806,.F.);
#12420=ORIENTED_EDGE('',*,*,#8807,.T.);
#12421=ORIENTED_EDGE('',*,*,#8808,.F.);
#12422=ORIENTED_EDGE('',*,*,#8716,.F.);
#12423=ORIENTED_EDGE('',*,*,#8809,.F.);
#12424=ORIENTED_EDGE('',*,*,#8717,.F.);
#12425=ORIENTED_EDGE('',*,*,#8808,.T.);
#12426=ORIENTED_EDGE('',*,*,#8810,.T.);
#12427=ORIENTED_EDGE('',*,*,#8811,.F.);
#12428=ORIENTED_EDGE('',*,*,#8810,.F.);
#12429=ORIENTED_EDGE('',*,*,#8807,.F.);
#12430=ORIENTED_EDGE('',*,*,#8812,.F.);
#12431=ORIENTED_EDGE('',*,*,#8813,.T.);
#12432=ORIENTED_EDGE('',*,*,#8814,.F.);
#12433=ORIENTED_EDGE('',*,*,#8719,.F.);
#12434=ORIENTED_EDGE('',*,*,#8815,.F.);
#12435=ORIENTED_EDGE('',*,*,#8720,.F.);
#12436=ORIENTED_EDGE('',*,*,#8814,.T.);
#12437=ORIENTED_EDGE('',*,*,#8816,.T.);
#12438=ORIENTED_EDGE('',*,*,#8817,.F.);
#12439=ORIENTED_EDGE('',*,*,#8816,.F.);
#12440=ORIENTED_EDGE('',*,*,#8813,.F.);
#12441=ORIENTED_EDGE('',*,*,#8818,.F.);
#12442=ORIENTED_EDGE('',*,*,#8819,.T.);
#12443=ORIENTED_EDGE('',*,*,#8820,.F.);
#12444=ORIENTED_EDGE('',*,*,#8722,.F.);
#12445=ORIENTED_EDGE('',*,*,#8821,.F.);
#12446=ORIENTED_EDGE('',*,*,#8723,.F.);
#12447=ORIENTED_EDGE('',*,*,#8820,.T.);
#12448=ORIENTED_EDGE('',*,*,#8822,.T.);
#12449=ORIENTED_EDGE('',*,*,#8823,.F.);
#12450=ORIENTED_EDGE('',*,*,#8822,.F.);
#12451=ORIENTED_EDGE('',*,*,#8819,.F.);
#12452=ORIENTED_EDGE('',*,*,#8824,.F.);
#12453=ORIENTED_EDGE('',*,*,#8825,.T.);
#12454=ORIENTED_EDGE('',*,*,#8826,.F.);
#12455=ORIENTED_EDGE('',*,*,#8725,.F.);
#12456=ORIENTED_EDGE('',*,*,#8827,.F.);
#12457=ORIENTED_EDGE('',*,*,#8620,.F.);
#12458=ORIENTED_EDGE('',*,*,#8826,.T.);
#12459=ORIENTED_EDGE('',*,*,#8828,.T.);
#12460=ORIENTED_EDGE('',*,*,#8829,.F.);
#12461=ORIENTED_EDGE('',*,*,#8828,.F.);
#12462=ORIENTED_EDGE('',*,*,#8825,.F.);
#12463=ORIENTED_EDGE('',*,*,#8830,.F.);
#12464=ORIENTED_EDGE('',*,*,#8831,.F.);
#12465=ORIENTED_EDGE('',*,*,#8832,.T.);
#12466=ORIENTED_EDGE('',*,*,#8833,.F.);
#12467=ORIENTED_EDGE('',*,*,#8622,.F.);
#12468=ORIENTED_EDGE('',*,*,#8834,.F.);
#12469=ORIENTED_EDGE('',*,*,#8623,.F.);
#12470=ORIENTED_EDGE('',*,*,#8833,.T.);
#12471=ORIENTED_EDGE('',*,*,#8835,.T.);
#12472=ORIENTED_EDGE('',*,*,#8836,.F.);
#12473=ORIENTED_EDGE('',*,*,#8835,.F.);
#12474=ORIENTED_EDGE('',*,*,#8832,.F.);
#12475=ORIENTED_EDGE('',*,*,#8837,.F.);
#12476=ORIENTED_EDGE('',*,*,#8838,.T.);
#12477=ORIENTED_EDGE('',*,*,#8839,.F.);
#12478=ORIENTED_EDGE('',*,*,#8625,.F.);
#12479=ORIENTED_EDGE('',*,*,#8840,.F.);
#12480=ORIENTED_EDGE('',*,*,#8626,.F.);
#12481=ORIENTED_EDGE('',*,*,#8839,.T.);
#12482=ORIENTED_EDGE('',*,*,#8841,.T.);
#12483=ORIENTED_EDGE('',*,*,#8842,.F.);
#12484=ORIENTED_EDGE('',*,*,#8841,.F.);
#12485=ORIENTED_EDGE('',*,*,#8838,.F.);
#12486=ORIENTED_EDGE('',*,*,#8843,.F.);
#12487=ORIENTED_EDGE('',*,*,#8844,.T.);
#12488=ORIENTED_EDGE('',*,*,#8845,.F.);
#12489=ORIENTED_EDGE('',*,*,#8628,.F.);
#12490=ORIENTED_EDGE('',*,*,#8846,.F.);
#12491=ORIENTED_EDGE('',*,*,#8629,.F.);
#12492=ORIENTED_EDGE('',*,*,#8845,.T.);
#12493=ORIENTED_EDGE('',*,*,#8847,.T.);
#12494=ORIENTED_EDGE('',*,*,#8848,.F.);
#12495=ORIENTED_EDGE('',*,*,#8847,.F.);
#12496=ORIENTED_EDGE('',*,*,#8844,.F.);
#12497=ORIENTED_EDGE('',*,*,#8849,.F.);
#12498=ORIENTED_EDGE('',*,*,#8850,.T.);
#12499=ORIENTED_EDGE('',*,*,#8851,.F.);
#12500=ORIENTED_EDGE('',*,*,#8631,.F.);
#12501=ORIENTED_EDGE('',*,*,#8852,.F.);
#12502=ORIENTED_EDGE('',*,*,#8632,.F.);
#12503=ORIENTED_EDGE('',*,*,#8851,.T.);
#12504=ORIENTED_EDGE('',*,*,#8853,.T.);
#12505=ORIENTED_EDGE('',*,*,#8854,.F.);
#12506=ORIENTED_EDGE('',*,*,#8853,.F.);
#12507=ORIENTED_EDGE('',*,*,#8850,.F.);
#12508=ORIENTED_EDGE('',*,*,#8855,.F.);
#12509=ORIENTED_EDGE('',*,*,#8856,.T.);
#12510=ORIENTED_EDGE('',*,*,#8857,.F.);
#12511=ORIENTED_EDGE('',*,*,#8634,.F.);
#12512=ORIENTED_EDGE('',*,*,#8858,.F.);
#12513=ORIENTED_EDGE('',*,*,#8635,.F.);
#12514=ORIENTED_EDGE('',*,*,#8857,.T.);
#12515=ORIENTED_EDGE('',*,*,#8859,.T.);
#12516=ORIENTED_EDGE('',*,*,#8860,.F.);
#12517=ORIENTED_EDGE('',*,*,#8859,.F.);
#12518=ORIENTED_EDGE('',*,*,#8856,.F.);
#12519=ORIENTED_EDGE('',*,*,#8861,.F.);
#12520=ORIENTED_EDGE('',*,*,#8862,.T.);
#12521=ORIENTED_EDGE('',*,*,#8863,.F.);
#12522=ORIENTED_EDGE('',*,*,#8637,.F.);
#12523=ORIENTED_EDGE('',*,*,#8864,.F.);
#12524=ORIENTED_EDGE('',*,*,#8638,.F.);
#12525=ORIENTED_EDGE('',*,*,#8863,.T.);
#12526=ORIENTED_EDGE('',*,*,#8865,.T.);
#12527=ORIENTED_EDGE('',*,*,#8866,.F.);
#12528=ORIENTED_EDGE('',*,*,#8865,.F.);
#12529=ORIENTED_EDGE('',*,*,#8862,.F.);
#12530=ORIENTED_EDGE('',*,*,#8867,.F.);
#12531=ORIENTED_EDGE('',*,*,#8868,.T.);
#12532=ORIENTED_EDGE('',*,*,#8869,.F.);
#12533=ORIENTED_EDGE('',*,*,#8640,.F.);
#12534=ORIENTED_EDGE('',*,*,#8870,.F.);
#12535=ORIENTED_EDGE('',*,*,#8641,.F.);
#12536=ORIENTED_EDGE('',*,*,#8869,.T.);
#12537=ORIENTED_EDGE('',*,*,#8871,.T.);
#12538=ORIENTED_EDGE('',*,*,#8872,.F.);
#12539=ORIENTED_EDGE('',*,*,#8871,.F.);
#12540=ORIENTED_EDGE('',*,*,#8868,.F.);
#12541=ORIENTED_EDGE('',*,*,#8873,.F.);
#12542=ORIENTED_EDGE('',*,*,#8874,.T.);
#12543=ORIENTED_EDGE('',*,*,#8875,.F.);
#12544=ORIENTED_EDGE('',*,*,#8643,.F.);
#12545=ORIENTED_EDGE('',*,*,#8876,.F.);
#12546=ORIENTED_EDGE('',*,*,#8644,.F.);
#12547=ORIENTED_EDGE('',*,*,#8875,.T.);
#12548=ORIENTED_EDGE('',*,*,#8877,.T.);
#12549=ORIENTED_EDGE('',*,*,#8878,.F.);
#12550=ORIENTED_EDGE('',*,*,#8877,.F.);
#12551=ORIENTED_EDGE('',*,*,#8874,.F.);
#12552=ORIENTED_EDGE('',*,*,#8879,.F.);
#12553=ORIENTED_EDGE('',*,*,#8880,.T.);
#12554=ORIENTED_EDGE('',*,*,#8881,.F.);
#12555=ORIENTED_EDGE('',*,*,#8646,.F.);
#12556=ORIENTED_EDGE('',*,*,#8882,.F.);
#12557=ORIENTED_EDGE('',*,*,#8647,.F.);
#12558=ORIENTED_EDGE('',*,*,#8881,.T.);
#12559=ORIENTED_EDGE('',*,*,#8883,.T.);
#12560=ORIENTED_EDGE('',*,*,#8884,.F.);
#12561=ORIENTED_EDGE('',*,*,#8883,.F.);
#12562=ORIENTED_EDGE('',*,*,#8880,.F.);
#12563=ORIENTED_EDGE('',*,*,#8885,.F.);
#12564=ORIENTED_EDGE('',*,*,#8886,.T.);
#12565=ORIENTED_EDGE('',*,*,#8887,.F.);
#12566=ORIENTED_EDGE('',*,*,#8649,.F.);
#12567=ORIENTED_EDGE('',*,*,#8888,.F.);
#12568=ORIENTED_EDGE('',*,*,#8650,.F.);
#12569=ORIENTED_EDGE('',*,*,#8887,.T.);
#12570=ORIENTED_EDGE('',*,*,#8889,.T.);
#12571=ORIENTED_EDGE('',*,*,#8890,.F.);
#12572=ORIENTED_EDGE('',*,*,#8889,.F.);
#12573=ORIENTED_EDGE('',*,*,#8886,.F.);
#12574=ORIENTED_EDGE('',*,*,#8891,.F.);
#12575=ORIENTED_EDGE('',*,*,#8892,.T.);
#12576=ORIENTED_EDGE('',*,*,#8893,.F.);
#12577=ORIENTED_EDGE('',*,*,#8652,.F.);
#12578=ORIENTED_EDGE('',*,*,#8894,.F.);
#12579=ORIENTED_EDGE('',*,*,#8653,.F.);
#12580=ORIENTED_EDGE('',*,*,#8893,.T.);
#12581=ORIENTED_EDGE('',*,*,#8895,.T.);
#12582=ORIENTED_EDGE('',*,*,#8896,.F.);
#12583=ORIENTED_EDGE('',*,*,#8895,.F.);
#12584=ORIENTED_EDGE('',*,*,#8892,.F.);
#12585=ORIENTED_EDGE('',*,*,#8897,.F.);
#12586=ORIENTED_EDGE('',*,*,#8898,.T.);
#12587=ORIENTED_EDGE('',*,*,#8899,.F.);
#12588=ORIENTED_EDGE('',*,*,#8655,.F.);
#12589=ORIENTED_EDGE('',*,*,#8900,.F.);
#12590=ORIENTED_EDGE('',*,*,#8656,.F.);
#12591=ORIENTED_EDGE('',*,*,#8899,.T.);
#12592=ORIENTED_EDGE('',*,*,#8901,.T.);
#12593=ORIENTED_EDGE('',*,*,#8902,.F.);
#12594=ORIENTED_EDGE('',*,*,#8901,.F.);
#12595=ORIENTED_EDGE('',*,*,#8898,.F.);
#12596=ORIENTED_EDGE('',*,*,#8903,.F.);
#12597=ORIENTED_EDGE('',*,*,#8904,.T.);
#12598=ORIENTED_EDGE('',*,*,#8905,.F.);
#12599=ORIENTED_EDGE('',*,*,#8658,.F.);
#12600=ORIENTED_EDGE('',*,*,#8906,.F.);
#12601=ORIENTED_EDGE('',*,*,#8659,.F.);
#12602=ORIENTED_EDGE('',*,*,#8905,.T.);
#12603=ORIENTED_EDGE('',*,*,#8907,.T.);
#12604=ORIENTED_EDGE('',*,*,#8908,.F.);
#12605=ORIENTED_EDGE('',*,*,#8907,.F.);
#12606=ORIENTED_EDGE('',*,*,#8904,.F.);
#12607=ORIENTED_EDGE('',*,*,#8909,.F.);
#12608=ORIENTED_EDGE('',*,*,#8910,.T.);
#12609=ORIENTED_EDGE('',*,*,#8911,.F.);
#12610=ORIENTED_EDGE('',*,*,#8661,.F.);
#12611=ORIENTED_EDGE('',*,*,#8912,.F.);
#12612=ORIENTED_EDGE('',*,*,#8662,.F.);
#12613=ORIENTED_EDGE('',*,*,#8911,.T.);
#12614=ORIENTED_EDGE('',*,*,#8913,.T.);
#12615=ORIENTED_EDGE('',*,*,#8914,.F.);
#12616=ORIENTED_EDGE('',*,*,#8913,.F.);
#12617=ORIENTED_EDGE('',*,*,#8910,.F.);
#12618=ORIENTED_EDGE('',*,*,#8915,.F.);
#12619=ORIENTED_EDGE('',*,*,#8916,.T.);
#12620=ORIENTED_EDGE('',*,*,#8917,.F.);
#12621=ORIENTED_EDGE('',*,*,#8664,.F.);
#12622=ORIENTED_EDGE('',*,*,#8918,.F.);
#12623=ORIENTED_EDGE('',*,*,#8665,.F.);
#12624=ORIENTED_EDGE('',*,*,#8917,.T.);
#12625=ORIENTED_EDGE('',*,*,#8919,.T.);
#12626=ORIENTED_EDGE('',*,*,#8920,.F.);
#12627=ORIENTED_EDGE('',*,*,#8919,.F.);
#12628=ORIENTED_EDGE('',*,*,#8916,.F.);
#12629=ORIENTED_EDGE('',*,*,#8921,.F.);
#12630=ORIENTED_EDGE('',*,*,#8922,.T.);
#12631=ORIENTED_EDGE('',*,*,#8923,.F.);
#12632=ORIENTED_EDGE('',*,*,#8667,.F.);
#12633=ORIENTED_EDGE('',*,*,#8924,.F.);
#12634=ORIENTED_EDGE('',*,*,#8668,.F.);
#12635=ORIENTED_EDGE('',*,*,#8923,.T.);
#12636=ORIENTED_EDGE('',*,*,#8925,.T.);
#12637=ORIENTED_EDGE('',*,*,#8926,.F.);
#12638=ORIENTED_EDGE('',*,*,#8925,.F.);
#12639=ORIENTED_EDGE('',*,*,#8922,.F.);
#12640=ORIENTED_EDGE('',*,*,#8927,.F.);
#12641=ORIENTED_EDGE('',*,*,#8928,.T.);
#12642=ORIENTED_EDGE('',*,*,#8929,.F.);
#12643=ORIENTED_EDGE('',*,*,#8670,.F.);
#12644=ORIENTED_EDGE('',*,*,#8930,.F.);
#12645=ORIENTED_EDGE('',*,*,#8671,.F.);
#12646=ORIENTED_EDGE('',*,*,#8929,.T.);
#12647=ORIENTED_EDGE('',*,*,#8931,.T.);
#12648=ORIENTED_EDGE('',*,*,#8932,.F.);
#12649=ORIENTED_EDGE('',*,*,#8931,.F.);
#12650=ORIENTED_EDGE('',*,*,#8928,.F.);
#12651=ORIENTED_EDGE('',*,*,#8933,.F.);
#12652=ORIENTED_EDGE('',*,*,#8934,.T.);
#12653=ORIENTED_EDGE('',*,*,#8935,.F.);
#12654=ORIENTED_EDGE('',*,*,#8673,.F.);
#12655=ORIENTED_EDGE('',*,*,#8936,.F.);
#12656=ORIENTED_EDGE('',*,*,#8674,.F.);
#12657=ORIENTED_EDGE('',*,*,#8935,.T.);
#12658=ORIENTED_EDGE('',*,*,#8937,.T.);
#12659=ORIENTED_EDGE('',*,*,#8938,.F.);
#12660=ORIENTED_EDGE('',*,*,#8937,.F.);
#12661=ORIENTED_EDGE('',*,*,#8934,.F.);
#12662=ORIENTED_EDGE('',*,*,#8829,.T.);
#12663=ORIENTED_EDGE('',*,*,#8939,.T.);
#12664=ORIENTED_EDGE('',*,*,#8609,.T.);
#12665=ORIENTED_EDGE('',*,*,#8939,.F.);
#12666=ORIENTED_EDGE('',*,*,#8830,.T.);
#12667=ORIENTED_EDGE('',*,*,#8824,.T.);
#12668=ORIENTED_EDGE('',*,*,#8724,.F.);
#12669=ORIENTED_EDGE('',*,*,#8821,.T.);
#12670=ORIENTED_EDGE('',*,*,#8823,.T.);
#12671=ORIENTED_EDGE('',*,*,#8818,.T.);
#12672=ORIENTED_EDGE('',*,*,#8721,.F.);
#12673=ORIENTED_EDGE('',*,*,#8815,.T.);
#12674=ORIENTED_EDGE('',*,*,#8817,.T.);
#12675=ORIENTED_EDGE('',*,*,#8812,.T.);
#12676=ORIENTED_EDGE('',*,*,#8718,.F.);
#12677=ORIENTED_EDGE('',*,*,#8809,.T.);
#12678=ORIENTED_EDGE('',*,*,#8811,.T.);
#12679=ORIENTED_EDGE('',*,*,#8806,.T.);
#12680=ORIENTED_EDGE('',*,*,#8715,.F.);
#12681=ORIENTED_EDGE('',*,*,#8803,.T.);
#12682=ORIENTED_EDGE('',*,*,#8805,.T.);
#12683=ORIENTED_EDGE('',*,*,#8800,.T.);
#12684=ORIENTED_EDGE('',*,*,#8712,.F.);
#12685=ORIENTED_EDGE('',*,*,#8797,.T.);
#12686=ORIENTED_EDGE('',*,*,#8799,.T.);
#12687=ORIENTED_EDGE('',*,*,#8794,.T.);
#12688=ORIENTED_EDGE('',*,*,#8709,.F.);
#12689=ORIENTED_EDGE('',*,*,#8791,.T.);
#12690=ORIENTED_EDGE('',*,*,#8793,.T.);
#12691=ORIENTED_EDGE('',*,*,#8788,.T.);
#12692=ORIENTED_EDGE('',*,*,#8706,.F.);
#12693=ORIENTED_EDGE('',*,*,#8785,.T.);
#12694=ORIENTED_EDGE('',*,*,#8787,.T.);
#12695=ORIENTED_EDGE('',*,*,#8782,.T.);
#12696=ORIENTED_EDGE('',*,*,#8703,.F.);
#12697=ORIENTED_EDGE('',*,*,#8779,.T.);
#12698=ORIENTED_EDGE('',*,*,#8781,.T.);
#12699=ORIENTED_EDGE('',*,*,#8776,.T.);
#12700=ORIENTED_EDGE('',*,*,#8700,.F.);
#12701=ORIENTED_EDGE('',*,*,#8773,.T.);
#12702=ORIENTED_EDGE('',*,*,#8775,.T.);
#12703=ORIENTED_EDGE('',*,*,#8770,.T.);
#12704=ORIENTED_EDGE('',*,*,#8697,.F.);
#12705=ORIENTED_EDGE('',*,*,#8767,.T.);
#12706=ORIENTED_EDGE('',*,*,#8769,.T.);
#12707=ORIENTED_EDGE('',*,*,#8764,.T.);
#12708=ORIENTED_EDGE('',*,*,#8694,.F.);
#12709=ORIENTED_EDGE('',*,*,#8761,.T.);
#12710=ORIENTED_EDGE('',*,*,#8763,.T.);
#12711=ORIENTED_EDGE('',*,*,#8758,.T.);
#12712=ORIENTED_EDGE('',*,*,#8691,.F.);
#12713=ORIENTED_EDGE('',*,*,#8755,.T.);
#12714=ORIENTED_EDGE('',*,*,#8757,.T.);
#12715=ORIENTED_EDGE('',*,*,#8752,.T.);
#12716=ORIENTED_EDGE('',*,*,#8688,.F.);
#12717=ORIENTED_EDGE('',*,*,#8749,.T.);
#12718=ORIENTED_EDGE('',*,*,#8751,.T.);
#12719=ORIENTED_EDGE('',*,*,#8746,.T.);
#12720=ORIENTED_EDGE('',*,*,#8685,.F.);
#12721=ORIENTED_EDGE('',*,*,#8743,.T.);
#12722=ORIENTED_EDGE('',*,*,#8745,.T.);
#12723=ORIENTED_EDGE('',*,*,#8740,.T.);
#12724=ORIENTED_EDGE('',*,*,#8682,.F.);
#12725=ORIENTED_EDGE('',*,*,#8737,.T.);
#12726=ORIENTED_EDGE('',*,*,#8739,.T.);
#12727=ORIENTED_EDGE('',*,*,#8734,.T.);
#12728=ORIENTED_EDGE('',*,*,#8679,.F.);
#12729=ORIENTED_EDGE('',*,*,#8731,.T.);
#12730=ORIENTED_EDGE('',*,*,#8733,.T.);
#12731=ORIENTED_EDGE('',*,*,#8728,.T.);
#12732=ORIENTED_EDGE('',*,*,#8676,.F.);
#12733=ORIENTED_EDGE('',*,*,#8616,.T.);
#12734=ORIENTED_EDGE('',*,*,#8619,.T.);
#12735=ORIENTED_EDGE('',*,*,#8612,.T.);
#12736=ORIENTED_EDGE('',*,*,#8675,.F.);
#12737=ORIENTED_EDGE('',*,*,#8936,.T.);
#12738=ORIENTED_EDGE('',*,*,#8938,.T.);
#12739=ORIENTED_EDGE('',*,*,#8933,.T.);
#12740=ORIENTED_EDGE('',*,*,#8672,.F.);
#12741=ORIENTED_EDGE('',*,*,#8930,.T.);
#12742=ORIENTED_EDGE('',*,*,#8932,.T.);
#12743=ORIENTED_EDGE('',*,*,#8927,.T.);
#12744=ORIENTED_EDGE('',*,*,#8669,.F.);
#12745=ORIENTED_EDGE('',*,*,#8924,.T.);
#12746=ORIENTED_EDGE('',*,*,#8926,.T.);
#12747=ORIENTED_EDGE('',*,*,#8921,.T.);
#12748=ORIENTED_EDGE('',*,*,#8666,.F.);
#12749=ORIENTED_EDGE('',*,*,#8918,.T.);
#12750=ORIENTED_EDGE('',*,*,#8920,.T.);
#12751=ORIENTED_EDGE('',*,*,#8915,.T.);
#12752=ORIENTED_EDGE('',*,*,#8663,.F.);
#12753=ORIENTED_EDGE('',*,*,#8912,.T.);
#12754=ORIENTED_EDGE('',*,*,#8914,.T.);
#12755=ORIENTED_EDGE('',*,*,#8909,.T.);
#12756=ORIENTED_EDGE('',*,*,#8660,.F.);
#12757=ORIENTED_EDGE('',*,*,#8906,.T.);
#12758=ORIENTED_EDGE('',*,*,#8908,.T.);
#12759=ORIENTED_EDGE('',*,*,#8903,.T.);
#12760=ORIENTED_EDGE('',*,*,#8657,.F.);
#12761=ORIENTED_EDGE('',*,*,#8900,.T.);
#12762=ORIENTED_EDGE('',*,*,#8902,.T.);
#12763=ORIENTED_EDGE('',*,*,#8897,.T.);
#12764=ORIENTED_EDGE('',*,*,#8654,.F.);
#12765=ORIENTED_EDGE('',*,*,#8894,.T.);
#12766=ORIENTED_EDGE('',*,*,#8896,.T.);
#12767=ORIENTED_EDGE('',*,*,#8891,.T.);
#12768=ORIENTED_EDGE('',*,*,#8651,.F.);
#12769=ORIENTED_EDGE('',*,*,#8888,.T.);
#12770=ORIENTED_EDGE('',*,*,#8890,.T.);
#12771=ORIENTED_EDGE('',*,*,#8885,.T.);
#12772=ORIENTED_EDGE('',*,*,#8648,.F.);
#12773=ORIENTED_EDGE('',*,*,#8882,.T.);
#12774=ORIENTED_EDGE('',*,*,#8884,.T.);
#12775=ORIENTED_EDGE('',*,*,#8879,.T.);
#12776=ORIENTED_EDGE('',*,*,#8645,.F.);
#12777=ORIENTED_EDGE('',*,*,#8876,.T.);
#12778=ORIENTED_EDGE('',*,*,#8878,.T.);
#12779=ORIENTED_EDGE('',*,*,#8873,.T.);
#12780=ORIENTED_EDGE('',*,*,#8642,.F.);
#12781=ORIENTED_EDGE('',*,*,#8870,.T.);
#12782=ORIENTED_EDGE('',*,*,#8872,.T.);
#12783=ORIENTED_EDGE('',*,*,#8867,.T.);
#12784=ORIENTED_EDGE('',*,*,#8639,.F.);
#12785=ORIENTED_EDGE('',*,*,#8864,.T.);
#12786=ORIENTED_EDGE('',*,*,#8866,.T.);
#12787=ORIENTED_EDGE('',*,*,#8861,.T.);
#12788=ORIENTED_EDGE('',*,*,#8636,.F.);
#12789=ORIENTED_EDGE('',*,*,#8858,.T.);
#12790=ORIENTED_EDGE('',*,*,#8860,.T.);
#12791=ORIENTED_EDGE('',*,*,#8855,.T.);
#12792=ORIENTED_EDGE('',*,*,#8633,.F.);
#12793=ORIENTED_EDGE('',*,*,#8852,.T.);
#12794=ORIENTED_EDGE('',*,*,#8854,.T.);
#12795=ORIENTED_EDGE('',*,*,#8849,.T.);
#12796=ORIENTED_EDGE('',*,*,#8630,.F.);
#12797=ORIENTED_EDGE('',*,*,#8846,.T.);
#12798=ORIENTED_EDGE('',*,*,#8848,.T.);
#12799=ORIENTED_EDGE('',*,*,#8843,.T.);
#12800=ORIENTED_EDGE('',*,*,#8627,.F.);
#12801=ORIENTED_EDGE('',*,*,#8840,.T.);
#12802=ORIENTED_EDGE('',*,*,#8842,.T.);
#12803=ORIENTED_EDGE('',*,*,#8837,.T.);
#12804=ORIENTED_EDGE('',*,*,#8624,.F.);
#12805=ORIENTED_EDGE('',*,*,#8834,.T.);
#12806=ORIENTED_EDGE('',*,*,#8836,.T.);
#12807=ORIENTED_EDGE('',*,*,#8831,.T.);
#12808=ORIENTED_EDGE('',*,*,#8621,.F.);
#12809=ORIENTED_EDGE('',*,*,#8827,.T.);
#12810=ORIENTED_EDGE('',*,*,#8727,.F.);
#12811=ORIENTED_EDGE('',*,*,#8940,.T.);
#12812=ORIENTED_EDGE('',*,*,#8941,.T.);
#12813=ORIENTED_EDGE('',*,*,#8942,.T.);
#12814=ORIENTED_EDGE('',*,*,#8943,.T.);
#12815=ORIENTED_EDGE('',*,*,#8944,.T.);
#12816=ORIENTED_EDGE('',*,*,#8945,.T.);
#12817=ORIENTED_EDGE('',*,*,#8946,.F.);
#12818=ORIENTED_EDGE('',*,*,#8947,.T.);
#12819=ORIENTED_EDGE('',*,*,#8948,.F.);
#12820=ORIENTED_EDGE('',*,*,#8949,.T.);
#12821=ORIENTED_EDGE('',*,*,#8950,.F.);
#12822=ORIENTED_EDGE('',*,*,#8951,.T.);
#12823=ORIENTED_EDGE('',*,*,#8952,.F.);
#12824=ORIENTED_EDGE('',*,*,#8953,.T.);
#12825=ORIENTED_EDGE('',*,*,#8954,.F.);
#12826=ORIENTED_EDGE('',*,*,#8955,.T.);
#12827=ORIENTED_EDGE('',*,*,#8956,.F.);
#12828=ORIENTED_EDGE('',*,*,#8957,.T.);
#12829=ORIENTED_EDGE('',*,*,#8958,.T.);
#12830=ORIENTED_EDGE('',*,*,#8957,.F.);
#12831=ORIENTED_EDGE('',*,*,#8955,.F.);
#12832=ORIENTED_EDGE('',*,*,#8953,.F.);
#12833=ORIENTED_EDGE('',*,*,#8951,.F.);
#12834=ORIENTED_EDGE('',*,*,#8949,.F.);
#12835=ORIENTED_EDGE('',*,*,#8947,.F.);
#12836=ORIENTED_EDGE('',*,*,#8958,.F.);
#12837=ORIENTED_EDGE('',*,*,#8940,.F.);
#12838=ORIENTED_EDGE('',*,*,#8959,.T.);
#12839=ORIENTED_EDGE('',*,*,#8946,.T.);
#12840=ORIENTED_EDGE('',*,*,#8960,.F.);
#12841=ORIENTED_EDGE('',*,*,#8945,.F.);
#12842=ORIENTED_EDGE('',*,*,#8961,.T.);
#12843=ORIENTED_EDGE('',*,*,#8956,.T.);
#12844=ORIENTED_EDGE('',*,*,#8959,.F.);
#12845=ORIENTED_EDGE('',*,*,#8944,.F.);
#12846=ORIENTED_EDGE('',*,*,#8962,.T.);
#12847=ORIENTED_EDGE('',*,*,#8954,.T.);
#12848=ORIENTED_EDGE('',*,*,#8961,.F.);
#12849=ORIENTED_EDGE('',*,*,#8943,.F.);
#12850=ORIENTED_EDGE('',*,*,#8963,.T.);
#12851=ORIENTED_EDGE('',*,*,#8952,.T.);
#12852=ORIENTED_EDGE('',*,*,#8962,.F.);
#12853=ORIENTED_EDGE('',*,*,#8942,.F.);
#12854=ORIENTED_EDGE('',*,*,#8964,.T.);
#12855=ORIENTED_EDGE('',*,*,#8950,.T.);
#12856=ORIENTED_EDGE('',*,*,#8963,.F.);
#12857=ORIENTED_EDGE('',*,*,#8941,.F.);
#12858=ORIENTED_EDGE('',*,*,#8960,.T.);
#12859=ORIENTED_EDGE('',*,*,#8948,.T.);
#12860=ORIENTED_EDGE('',*,*,#8964,.F.);
#12970=CYLINDRICAL_SURFACE('',#14611,2.40538);
#12971=CYLINDRICAL_SURFACE('',#14613,2.40538);
#12972=CYLINDRICAL_SURFACE('',#14614,2.40538);
#12973=CYLINDRICAL_SURFACE('',#14615,2.40538);
#12974=CYLINDRICAL_SURFACE('',#14616,2.40538);
#12975=CYLINDRICAL_SURFACE('',#14617,2.40538);
#12976=CYLINDRICAL_SURFACE('',#14618,2.40538);
#12977=CYLINDRICAL_SURFACE('',#14619,2.40538);
#12978=CYLINDRICAL_SURFACE('',#14620,2.40538);
#12979=CYLINDRICAL_SURFACE('',#14621,2.40538);
#12980=CYLINDRICAL_SURFACE('',#14622,2.40538);
#12981=CYLINDRICAL_SURFACE('',#14623,2.40538);
#12982=CYLINDRICAL_SURFACE('',#14624,2.40538);
#12983=CYLINDRICAL_SURFACE('',#14625,2.40538);
#12984=CYLINDRICAL_SURFACE('',#14626,3.11023);
#12985=CYLINDRICAL_SURFACE('',#14629,2.40538);
#12986=CYLINDRICAL_SURFACE('',#14828,4.7625);
#13487=ADVANCED_FACE('',(#2527),#12970,.T.);
#13488=ADVANCED_FACE('',(#2528),#12971,.T.);
#13489=ADVANCED_FACE('',(#2529),#12972,.T.);
#13490=ADVANCED_FACE('',(#2530),#12973,.T.);
#13491=ADVANCED_FACE('',(#2531),#12974,.T.);
#13492=ADVANCED_FACE('',(#2532),#12975,.T.);
#13493=ADVANCED_FACE('',(#2533),#12976,.T.);
#13494=ADVANCED_FACE('',(#2534),#12977,.T.);
#13495=ADVANCED_FACE('',(#2535),#12978,.T.);
#13496=ADVANCED_FACE('',(#2536),#12979,.T.);
#13497=ADVANCED_FACE('',(#2537),#12980,.T.);
#13498=ADVANCED_FACE('',(#2538),#12981,.T.);
#13499=ADVANCED_FACE('',(#2539),#12982,.T.);
#13500=ADVANCED_FACE('',(#2540),#12983,.T.);
#13501=ADVANCED_FACE('',(#2541),#12984,.T.);
#13502=ADVANCED_FACE('',(#2542),#12985,.T.);
#13503=ADVANCED_FACE('',(#2543),#1902,.T.);
#13504=ADVANCED_FACE('',(#2544),#1010,.F.);
#13505=ADVANCED_FACE('',(#2545),#1903,.F.);
#13506=ADVANCED_FACE('',(#2546),#1011,.F.);
#13507=ADVANCED_FACE('',(#2547),#1005,.F.);
#13508=ADVANCED_FACE('',(#2548,#1563),#1904,.F.);
#13509=ADVANCED_FACE('',(#2549),#1100,.T.);
#13510=ADVANCED_FACE('',(#2550),#1905,.F.);
#13511=ADVANCED_FACE('',(#2551),#1906,.F.);
#13512=ADVANCED_FACE('',(#2552),#1907,.F.);
#13513=ADVANCED_FACE('',(#2553),#1908,.F.);
#13514=ADVANCED_FACE('',(#2554),#1101,.T.);
#13515=ADVANCED_FACE('',(#2555),#1909,.F.);
#13516=ADVANCED_FACE('',(#2556),#1910,.F.);
#13517=ADVANCED_FACE('',(#2557),#1911,.F.);
#13518=ADVANCED_FACE('',(#2558),#1912,.F.);
#13519=ADVANCED_FACE('',(#2559),#1913,.F.);
#13520=ADVANCED_FACE('',(#2560),#1914,.F.);
#13521=ADVANCED_FACE('',(#2561),#1915,.F.);
#13522=ADVANCED_FACE('',(#2562),#1916,.F.);
#13523=ADVANCED_FACE('',(#2563),#1917,.F.);
#13524=ADVANCED_FACE('',(#2564),#1918,.F.);
#13525=ADVANCED_FACE('',(#2565),#1919,.F.);
#13526=ADVANCED_FACE('',(#2566),#1920,.F.);
#13527=ADVANCED_FACE('',(#2567),#1921,.F.);
#13528=ADVANCED_FACE('',(#2568),#1922,.F.);
#13529=ADVANCED_FACE('',(#2569),#1923,.F.);
#13530=ADVANCED_FACE('',(#2570),#1924,.F.);
#13531=ADVANCED_FACE('',(#2571),#1925,.F.);
#13532=ADVANCED_FACE('',(#2572),#1926,.F.);
#13533=ADVANCED_FACE('',(#2573),#1927,.F.);
#13534=ADVANCED_FACE('',(#2574),#1928,.F.);
#13535=ADVANCED_FACE('',(#2575),#1929,.F.);
#13536=ADVANCED_FACE('',(#2576),#1930,.F.);
#13537=ADVANCED_FACE('',(#2577),#1931,.F.);
#13538=ADVANCED_FACE('',(#2578),#1932,.F.);
#13539=ADVANCED_FACE('',(#2579),#1933,.F.);
#13540=ADVANCED_FACE('',(#2580),#1934,.F.);
#13541=ADVANCED_FACE('',(#2581),#1935,.F.);
#13542=ADVANCED_FACE('',(#2582),#1936,.F.);
#13543=ADVANCED_FACE('',(#2583),#1937,.F.);
#13544=ADVANCED_FACE('',(#2584),#1938,.F.);
#13545=ADVANCED_FACE('',(#2585),#1939,.F.);
#13546=ADVANCED_FACE('',(#2586),#1940,.F.);
#13547=ADVANCED_FACE('',(#2587),#1941,.F.);
#13548=ADVANCED_FACE('',(#2588),#1942,.F.);
#13549=ADVANCED_FACE('',(#2589),#1943,.F.);
#13550=ADVANCED_FACE('',(#2590),#1944,.F.);
#13551=ADVANCED_FACE('',(#2591),#1945,.F.);
#13552=ADVANCED_FACE('',(#2592),#1946,.F.);
#13553=ADVANCED_FACE('',(#2593),#1947,.F.);
#13554=ADVANCED_FACE('',(#2594),#1948,.F.);
#13555=ADVANCED_FACE('',(#2595),#1949,.F.);
#13556=ADVANCED_FACE('',(#2596),#1950,.F.);
#13557=ADVANCED_FACE('',(#2597),#1951,.F.);
#13558=ADVANCED_FACE('',(#2598),#1952,.F.);
#13559=ADVANCED_FACE('',(#2599),#1953,.F.);
#13560=ADVANCED_FACE('',(#2600),#1954,.F.);
#13561=ADVANCED_FACE('',(#2601),#1955,.F.);
#13562=ADVANCED_FACE('',(#2602),#1956,.F.);
#13563=ADVANCED_FACE('',(#2603),#1957,.F.);
#13564=ADVANCED_FACE('',(#2604),#1958,.F.);
#13565=ADVANCED_FACE('',(#2605),#1959,.F.);
#13566=ADVANCED_FACE('',(#2606),#1960,.F.);
#13567=ADVANCED_FACE('',(#2607),#1961,.F.);
#13568=ADVANCED_FACE('',(#2608),#1962,.F.);
#13569=ADVANCED_FACE('',(#2609),#1963,.F.);
#13570=ADVANCED_FACE('',(#2610),#1964,.F.);
#13571=ADVANCED_FACE('',(#2611),#1965,.F.);
#13572=ADVANCED_FACE('',(#2612),#1966,.F.);
#13573=ADVANCED_FACE('',(#2613),#1967,.F.);
#13574=ADVANCED_FACE('',(#2614),#1968,.F.);
#13575=ADVANCED_FACE('',(#2615),#1969,.F.);
#13576=ADVANCED_FACE('',(#2616),#1970,.F.);
#13577=ADVANCED_FACE('',(#2617),#1971,.F.);
#13578=ADVANCED_FACE('',(#2618),#1972,.F.);
#13579=ADVANCED_FACE('',(#2619),#1973,.F.);
#13580=ADVANCED_FACE('',(#2620),#1974,.F.);
#13581=ADVANCED_FACE('',(#2621),#1975,.F.);
#13582=ADVANCED_FACE('',(#2622),#1976,.F.);
#13583=ADVANCED_FACE('',(#2623),#1977,.F.);
#13584=ADVANCED_FACE('',(#2624),#1978,.F.);
#13585=ADVANCED_FACE('',(#2625),#1979,.F.);
#13586=ADVANCED_FACE('',(#2626),#1980,.F.);
#13587=ADVANCED_FACE('',(#2627),#1981,.F.);
#13588=ADVANCED_FACE('',(#2628),#1982,.F.);
#13589=ADVANCED_FACE('',(#2629),#1983,.F.);
#13590=ADVANCED_FACE('',(#2630),#1984,.F.);
#13591=ADVANCED_FACE('',(#2631),#1985,.F.);
#13592=ADVANCED_FACE('',(#2632),#1986,.F.);
#13593=ADVANCED_FACE('',(#2633),#1987,.F.);
#13594=ADVANCED_FACE('',(#2634),#1988,.F.);
#13595=ADVANCED_FACE('',(#2635),#1989,.F.);
#13596=ADVANCED_FACE('',(#2636),#1990,.F.);
#13597=ADVANCED_FACE('',(#2637),#1991,.F.);
#13598=ADVANCED_FACE('',(#2638),#1992,.F.);
#13599=ADVANCED_FACE('',(#2639),#1993,.F.);
#13600=ADVANCED_FACE('',(#2640),#1994,.F.);
#13601=ADVANCED_FACE('',(#2641),#1995,.F.);
#13602=ADVANCED_FACE('',(#2642),#1996,.F.);
#13603=ADVANCED_FACE('',(#2643),#1997,.F.);
#13604=ADVANCED_FACE('',(#2644),#1998,.F.);
#13605=ADVANCED_FACE('',(#2645),#1999,.F.);
#13606=ADVANCED_FACE('',(#2646),#2000,.F.);
#13607=ADVANCED_FACE('',(#2647),#2001,.F.);
#13608=ADVANCED_FACE('',(#2648),#2002,.F.);
#13609=ADVANCED_FACE('',(#2649),#2003,.F.);
#13610=ADVANCED_FACE('',(#2650),#2004,.F.);
#13611=ADVANCED_FACE('',(#2651),#2005,.F.);
#13612=ADVANCED_FACE('',(#2652),#2006,.F.);
#13613=ADVANCED_FACE('',(#2653),#2007,.F.);
#13614=ADVANCED_FACE('',(#2654),#2008,.F.);
#13615=ADVANCED_FACE('',(#2655),#2009,.F.);
#13616=ADVANCED_FACE('',(#2656),#2010,.F.);
#13617=ADVANCED_FACE('',(#2657),#2011,.F.);
#13618=ADVANCED_FACE('',(#2658),#2012,.F.);
#13619=ADVANCED_FACE('',(#2659),#2013,.F.);
#13620=ADVANCED_FACE('',(#2660),#12986,.T.);
#13621=ADVANCED_FACE('',(#2661,#1564),#2014,.T.);
#13622=ADVANCED_FACE('',(#2662),#2015,.F.);
#13623=ADVANCED_FACE('',(#2663),#2016,.F.);
#13624=ADVANCED_FACE('',(#2664),#2017,.F.);
#13625=ADVANCED_FACE('',(#2665),#2018,.F.);
#13626=ADVANCED_FACE('',(#2666),#2019,.F.);
#13627=ADVANCED_FACE('',(#2667),#2020,.F.);
#13628=ADVANCED_FACE('',(#2668),#1102,.F.);
#13629=ADVANCED_FACE('',(#2669),#2021,.F.);
#13630=ADVANCED_FACE('',(#2670),#2022,.F.);
#13631=ADVANCED_FACE('',(#2671),#2023,.F.);
#13632=ADVANCED_FACE('',(#2672),#2024,.F.);
#13633=ADVANCED_FACE('',(#2673),#2025,.F.);
#13634=ADVANCED_FACE('',(#2674),#2026,.F.);
#13644=CLOSED_SHELL('',(#13487,#13488,#13489,#13490,#13491,#13492,#13493,
#13494,#13495,#13496,#13497,#13498,#13499,#13500,#13501,#13502,#13503,#13504,
#13505,#13506,#13507,#13508,#13509,#13510,#13511,#13512,#13513,#13514,#13515,
#13516,#13517,#13518,#13519,#13520,#13521,#13522,#13523,#13524,#13525,#13526,
#13527,#13528,#13529,#13530,#13531,#13532,#13533,#13534,#13535,#13536,#13537,
#13538,#13539,#13540,#13541,#13542,#13543,#13544,#13545,#13546,#13547,#13548,
#13549,#13550,#13551,#13552,#13553,#13554,#13555,#13556,#13557,#13558,#13559,
#13560,#13561,#13562,#13563,#13564,#13565,#13566,#13567,#13568,#13569,#13570,
#13571,#13572,#13573,#13574,#13575,#13576,#13577,#13578,#13579,#13580,#13581,
#13582,#13583,#13584,#13585,#13586,#13587,#13588,#13589,#13590,#13591,#13592,
#13593,#13594,#13595,#13596,#13597,#13598,#13599,#13600,#13601,#13602,#13603,
#13604,#13605,#13606,#13607,#13608,#13609,#13610,#13611,#13612,#13613,#13614,
#13615,#13616,#13617,#13618,#13619,#13620,#13621,#13622,#13623,#13624,#13625,
#13626,#13627,#13628,#13629,#13630,#13631,#13632,#13633,#13634));
#14610=AXIS2_PLACEMENT_3D('',#59757,#17446,#17447);
#14611=AXIS2_PLACEMENT_3D('',#59758,#17448,#17449);
#14612=AXIS2_PLACEMENT_3D('',#59918,#17451,#17452);
#14613=AXIS2_PLACEMENT_3D('',#60031,#17453,#17454);
#14614=AXIS2_PLACEMENT_3D('',#60431,#17456,#17457);
#14615=AXIS2_PLACEMENT_3D('',#60647,#17459,#17460);
#14616=AXIS2_PLACEMENT_3D('',#60869,#17462,#17463);
#14617=AXIS2_PLACEMENT_3D('',#61252,#17465,#17466);
#14618=AXIS2_PLACEMENT_3D('',#61637,#17468,#17469);
#14619=AXIS2_PLACEMENT_3D('',#62094,#17471,#17472);
#14620=AXIS2_PLACEMENT_3D('',#62577,#17474,#17475);
#14621=AXIS2_PLACEMENT_3D('',#63072,#17477,#17478);
#14622=AXIS2_PLACEMENT_3D('',#63303,#17480,#17481);
#14623=AXIS2_PLACEMENT_3D('',#63540,#17483,#17484);
#14624=AXIS2_PLACEMENT_3D('',#63911,#17486,#17487);
#14625=AXIS2_PLACEMENT_3D('',#64379,#17489,#17490);
#14626=AXIS2_PLACEMENT_3D('',#64761,#17492,#17493);
#14627=AXIS2_PLACEMENT_3D('',#64835,#17494,#17495);
#14628=AXIS2_PLACEMENT_3D('',#67071,#17496,#17497);
#14629=AXIS2_PLACEMENT_3D('',#69226,#17498,#17499);
#14630=AXIS2_PLACEMENT_3D('',#69407,#17500,#17501);
#14631=AXIS2_PLACEMENT_3D('',#69554,#17502,#17503);
#14632=AXIS2_PLACEMENT_3D('',#69557,#17504,#17505);
#14633=AXIS2_PLACEMENT_3D('',#69745,#17506,#17507);
#14634=AXIS2_PLACEMENT_3D('',#70226,#17508,#17509);
#14635=AXIS2_PLACEMENT_3D('',#70229,#17510,#17511);
#14636=AXIS2_PLACEMENT_3D('',#70321,#17512,#17513);
#14637=AXIS2_PLACEMENT_3D('',#70714,#17514,#17515);
#14638=AXIS2_PLACEMENT_3D('',#70716,#17516,#17517);
#14639=AXIS2_PLACEMENT_3D('',#70717,#17518,#17519);
#14640=AXIS2_PLACEMENT_3D('',#70718,#17520,#17521);
#14641=AXIS2_PLACEMENT_3D('',#70720,#17522,#17523);
#14642=AXIS2_PLACEMENT_3D('',#70721,#17524,#17525);
#14643=AXIS2_PLACEMENT_3D('',#70724,#17527,#17528);
#14644=AXIS2_PLACEMENT_3D('',#70725,#17529,#17530);
#14645=AXIS2_PLACEMENT_3D('',#70726,#17531,#17532);
#14646=AXIS2_PLACEMENT_3D('',#70737,#17536,#17537);
#14647=AXIS2_PLACEMENT_3D('',#70745,#17540,#17541);
#14648=AXIS2_PLACEMENT_3D('',#70746,#17542,#17543);
#14649=AXIS2_PLACEMENT_3D('',#70747,#17544,#17545);
#14650=AXIS2_PLACEMENT_3D('',#70754,#17546,#17547);
#14651=AXIS2_PLACEMENT_3D('',#70764,#17548,#17549);
#14652=AXIS2_PLACEMENT_3D('',#70774,#17550,#17551);
#14653=AXIS2_PLACEMENT_3D('',#70784,#17552,#17553);
#14654=AXIS2_PLACEMENT_3D('',#70794,#17554,#17555);
#14655=AXIS2_PLACEMENT_3D('',#70804,#17556,#17557);
#14656=AXIS2_PLACEMENT_3D('',#70814,#17558,#17559);
#14657=AXIS2_PLACEMENT_3D('',#70824,#17560,#17561);
#14658=AXIS2_PLACEMENT_3D('',#70834,#17562,#17563);
#14659=AXIS2_PLACEMENT_3D('',#70844,#17564,#17565);
#14660=AXIS2_PLACEMENT_3D('',#70854,#17566,#17567);
#14661=AXIS2_PLACEMENT_3D('',#70864,#17568,#17569);
#14662=AXIS2_PLACEMENT_3D('',#70874,#17570,#17571);
#14663=AXIS2_PLACEMENT_3D('',#70884,#17572,#17573);
#14664=AXIS2_PLACEMENT_3D('',#70894,#17574,#17575);
#14665=AXIS2_PLACEMENT_3D('',#70904,#17576,#17577);
#14666=AXIS2_PLACEMENT_3D('',#70914,#17578,#17579);
#14667=AXIS2_PLACEMENT_3D('',#70924,#17580,#17581);
#14668=AXIS2_PLACEMENT_3D('',#70933,#17582,#17583);
#14669=AXIS2_PLACEMENT_3D('',#70935,#17584,#17585);
#14670=AXIS2_PLACEMENT_3D('',#70945,#17586,#17587);
#14671=AXIS2_PLACEMENT_3D('',#70955,#17588,#17589);
#14672=AXIS2_PLACEMENT_3D('',#70965,#17590,#17591);
#14673=AXIS2_PLACEMENT_3D('',#70975,#17592,#17593);
#14674=AXIS2_PLACEMENT_3D('',#70985,#17594,#17595);
#14675=AXIS2_PLACEMENT_3D('',#70995,#17596,#17597);
#14676=AXIS2_PLACEMENT_3D('',#71005,#17598,#17599);
#14677=AXIS2_PLACEMENT_3D('',#71015,#17600,#17601);
#14678=AXIS2_PLACEMENT_3D('',#71025,#17602,#17603);
#14679=AXIS2_PLACEMENT_3D('',#71035,#17604,#17605);
#14680=AXIS2_PLACEMENT_3D('',#71045,#17606,#17607);
#14681=AXIS2_PLACEMENT_3D('',#71055,#17608,#17609);
#14682=AXIS2_PLACEMENT_3D('',#71065,#17610,#17611);
#14683=AXIS2_PLACEMENT_3D('',#71075,#17612,#17613);
#14684=AXIS2_PLACEMENT_3D('',#71085,#17614,#17615);
#14685=AXIS2_PLACEMENT_3D('',#71095,#17616,#17617);
#14686=AXIS2_PLACEMENT_3D('',#71101,#17619,#17620);
#14687=AXIS2_PLACEMENT_3D('',#71102,#17621,#17622);
#14688=AXIS2_PLACEMENT_3D('',#71108,#17626,#17627);
#14689=AXIS2_PLACEMENT_3D('',#71112,#17630,#17631);
#14690=AXIS2_PLACEMENT_3D('',#71113,#17632,#17633);
#14691=AXIS2_PLACEMENT_3D('',#71114,#17634,#17635);
#14692=AXIS2_PLACEMENT_3D('',#71120,#17639,#17640);
#14693=AXIS2_PLACEMENT_3D('',#71124,#17643,#17644);
#14694=AXIS2_PLACEMENT_3D('',#71125,#17645,#17646);
#14695=AXIS2_PLACEMENT_3D('',#71126,#17647,#17648);
#14696=AXIS2_PLACEMENT_3D('',#71132,#17652,#17653);
#14697=AXIS2_PLACEMENT_3D('',#71136,#17656,#17657);
#14698=AXIS2_PLACEMENT_3D('',#71137,#17658,#17659);
#14699=AXIS2_PLACEMENT_3D('',#71138,#17660,#17661);
#14700=AXIS2_PLACEMENT_3D('',#71144,#17665,#17666);
#14701=AXIS2_PLACEMENT_3D('',#71148,#17669,#17670);
#14702=AXIS2_PLACEMENT_3D('',#71149,#17671,#17672);
#14703=AXIS2_PLACEMENT_3D('',#71150,#17673,#17674);
#14704=AXIS2_PLACEMENT_3D('',#71156,#17678,#17679);
#14705=AXIS2_PLACEMENT_3D('',#71160,#17682,#17683);
#14706=AXIS2_PLACEMENT_3D('',#71161,#17684,#17685);
#14707=AXIS2_PLACEMENT_3D('',#71162,#17686,#17687);
#14708=AXIS2_PLACEMENT_3D('',#71168,#17691,#17692);
#14709=AXIS2_PLACEMENT_3D('',#71172,#17695,#17696);
#14710=AXIS2_PLACEMENT_3D('',#71173,#17697,#17698);
#14711=AXIS2_PLACEMENT_3D('',#71174,#17699,#17700);
#14712=AXIS2_PLACEMENT_3D('',#71180,#17704,#17705);
#14713=AXIS2_PLACEMENT_3D('',#71184,#17708,#17709);
#14714=AXIS2_PLACEMENT_3D('',#71185,#17710,#17711);
#14715=AXIS2_PLACEMENT_3D('',#71186,#17712,#17713);
#14716=AXIS2_PLACEMENT_3D('',#71192,#17717,#17718);
#14717=AXIS2_PLACEMENT_3D('',#71196,#17721,#17722);
#14718=AXIS2_PLACEMENT_3D('',#71197,#17723,#17724);
#14719=AXIS2_PLACEMENT_3D('',#71198,#17725,#17726);
#14720=AXIS2_PLACEMENT_3D('',#71204,#17730,#17731);
#14721=AXIS2_PLACEMENT_3D('',#71208,#17734,#17735);
#14722=AXIS2_PLACEMENT_3D('',#71209,#17736,#17737);
#14723=AXIS2_PLACEMENT_3D('',#71210,#17738,#17739);
#14724=AXIS2_PLACEMENT_3D('',#71216,#17743,#17744);
#14725=AXIS2_PLACEMENT_3D('',#71220,#17747,#17748);
#14726=AXIS2_PLACEMENT_3D('',#71221,#17749,#17750);
#14727=AXIS2_PLACEMENT_3D('',#71222,#17751,#17752);
#14728=AXIS2_PLACEMENT_3D('',#71228,#17756,#17757);
#14729=AXIS2_PLACEMENT_3D('',#71232,#17760,#17761);
#14730=AXIS2_PLACEMENT_3D('',#71233,#17762,#17763);
#14731=AXIS2_PLACEMENT_3D('',#71234,#17764,#17765);
#14732=AXIS2_PLACEMENT_3D('',#71240,#17769,#17770);
#14733=AXIS2_PLACEMENT_3D('',#71244,#17773,#17774);
#14734=AXIS2_PLACEMENT_3D('',#71245,#17775,#17776);
#14735=AXIS2_PLACEMENT_3D('',#71246,#17777,#17778);
#14736=AXIS2_PLACEMENT_3D('',#71252,#17782,#17783);
#14737=AXIS2_PLACEMENT_3D('',#71256,#17786,#17787);
#14738=AXIS2_PLACEMENT_3D('',#71257,#17788,#17789);
#14739=AXIS2_PLACEMENT_3D('',#71258,#17790,#17791);
#14740=AXIS2_PLACEMENT_3D('',#71264,#17795,#17796);
#14741=AXIS2_PLACEMENT_3D('',#71268,#17799,#17800);
#14742=AXIS2_PLACEMENT_3D('',#71269,#17801,#17802);
#14743=AXIS2_PLACEMENT_3D('',#71270,#17803,#17804);
#14744=AXIS2_PLACEMENT_3D('',#71276,#17808,#17809);
#14745=AXIS2_PLACEMENT_3D('',#71280,#17812,#17813);
#14746=AXIS2_PLACEMENT_3D('',#71281,#17814,#17815);
#14747=AXIS2_PLACEMENT_3D('',#71282,#17816,#17817);
#14748=AXIS2_PLACEMENT_3D('',#71288,#17821,#17822);
#14749=AXIS2_PLACEMENT_3D('',#71292,#17825,#17826);
#14750=AXIS2_PLACEMENT_3D('',#71293,#17827,#17828);
#14751=AXIS2_PLACEMENT_3D('',#71294,#17829,#17830);
#14752=AXIS2_PLACEMENT_3D('',#71300,#17834,#17835);
#14753=AXIS2_PLACEMENT_3D('',#71304,#17838,#17839);
#14754=AXIS2_PLACEMENT_3D('',#71306,#17840,#17841);
#14755=AXIS2_PLACEMENT_3D('',#71307,#17842,#17843);
#14756=AXIS2_PLACEMENT_3D('',#71308,#17844,#17845);
#14757=AXIS2_PLACEMENT_3D('',#71314,#17849,#17850);
#14758=AXIS2_PLACEMENT_3D('',#71318,#17853,#17854);
#14759=AXIS2_PLACEMENT_3D('',#71319,#17855,#17856);
#14760=AXIS2_PLACEMENT_3D('',#71320,#17857,#17858);
#14761=AXIS2_PLACEMENT_3D('',#71326,#17862,#17863);
#14762=AXIS2_PLACEMENT_3D('',#71330,#17866,#17867);
#14763=AXIS2_PLACEMENT_3D('',#71331,#17868,#17869);
#14764=AXIS2_PLACEMENT_3D('',#71332,#17870,#17871);
#14765=AXIS2_PLACEMENT_3D('',#71338,#17875,#17876);
#14766=AXIS2_PLACEMENT_3D('',#71342,#17879,#17880);
#14767=AXIS2_PLACEMENT_3D('',#71343,#17881,#17882);
#14768=AXIS2_PLACEMENT_3D('',#71344,#17883,#17884);
#14769=AXIS2_PLACEMENT_3D('',#71350,#17888,#17889);
#14770=AXIS2_PLACEMENT_3D('',#71354,#17892,#17893);
#14771=AXIS2_PLACEMENT_3D('',#71355,#17894,#17895);
#14772=AXIS2_PLACEMENT_3D('',#71356,#17896,#17897);
#14773=AXIS2_PLACEMENT_3D('',#71362,#17901,#17902);
#14774=AXIS2_PLACEMENT_3D('',#71366,#17905,#17906);
#14775=AXIS2_PLACEMENT_3D('',#71367,#17907,#17908);
#14776=AXIS2_PLACEMENT_3D('',#71368,#17909,#17910);
#14777=AXIS2_PLACEMENT_3D('',#71374,#17914,#17915);
#14778=AXIS2_PLACEMENT_3D('',#71378,#17918,#17919);
#14779=AXIS2_PLACEMENT_3D('',#71379,#17920,#17921);
#14780=AXIS2_PLACEMENT_3D('',#71380,#17922,#17923);
#14781=AXIS2_PLACEMENT_3D('',#71386,#17927,#17928);
#14782=AXIS2_PLACEMENT_3D('',#71390,#17931,#17932);
#14783=AXIS2_PLACEMENT_3D('',#71391,#17933,#17934);
#14784=AXIS2_PLACEMENT_3D('',#71392,#17935,#17936);
#14785=AXIS2_PLACEMENT_3D('',#71398,#17940,#17941);
#14786=AXIS2_PLACEMENT_3D('',#71402,#17944,#17945);
#14787=AXIS2_PLACEMENT_3D('',#71403,#17946,#17947);
#14788=AXIS2_PLACEMENT_3D('',#71404,#17948,#17949);
#14789=AXIS2_PLACEMENT_3D('',#71410,#17953,#17954);
#14790=AXIS2_PLACEMENT_3D('',#71414,#17957,#17958);
#14791=AXIS2_PLACEMENT_3D('',#71415,#17959,#17960);
#14792=AXIS2_PLACEMENT_3D('',#71416,#17961,#17962);
#14793=AXIS2_PLACEMENT_3D('',#71422,#17966,#17967);
#14794=AXIS2_PLACEMENT_3D('',#71426,#17970,#17971);
#14795=AXIS2_PLACEMENT_3D('',#71427,#17972,#17973);
#14796=AXIS2_PLACEMENT_3D('',#71428,#17974,#17975);
#14797=AXIS2_PLACEMENT_3D('',#71434,#17979,#17980);
#14798=AXIS2_PLACEMENT_3D('',#71438,#17983,#17984);
#14799=AXIS2_PLACEMENT_3D('',#71439,#17985,#17986);
#14800=AXIS2_PLACEMENT_3D('',#71440,#17987,#17988);
#14801=AXIS2_PLACEMENT_3D('',#71446,#17992,#17993);
#14802=AXIS2_PLACEMENT_3D('',#71450,#17996,#17997);
#14803=AXIS2_PLACEMENT_3D('',#71451,#17998,#17999);
#14804=AXIS2_PLACEMENT_3D('',#71452,#18000,#18001);
#14805=AXIS2_PLACEMENT_3D('',#71458,#18005,#18006);
#14806=AXIS2_PLACEMENT_3D('',#71462,#18009,#18010);
#14807=AXIS2_PLACEMENT_3D('',#71463,#18011,#18012);
#14808=AXIS2_PLACEMENT_3D('',#71464,#18013,#18014);
#14809=AXIS2_PLACEMENT_3D('',#71470,#18018,#18019);
#14810=AXIS2_PLACEMENT_3D('',#71474,#18022,#18023);
#14811=AXIS2_PLACEMENT_3D('',#71475,#18024,#18025);
#14812=AXIS2_PLACEMENT_3D('',#71476,#18026,#18027);
#14813=AXIS2_PLACEMENT_3D('',#71482,#18031,#18032);
#14814=AXIS2_PLACEMENT_3D('',#71486,#18035,#18036);
#14815=AXIS2_PLACEMENT_3D('',#71487,#18037,#18038);
#14816=AXIS2_PLACEMENT_3D('',#71488,#18039,#18040);
#14817=AXIS2_PLACEMENT_3D('',#71494,#18044,#18045);
#14818=AXIS2_PLACEMENT_3D('',#71498,#18048,#18049);
#14819=AXIS2_PLACEMENT_3D('',#71499,#18050,#18051);
#14820=AXIS2_PLACEMENT_3D('',#71500,#18052,#18053);
#14821=AXIS2_PLACEMENT_3D('',#71506,#18057,#18058);
#14822=AXIS2_PLACEMENT_3D('',#71510,#18061,#18062);
#14823=AXIS2_PLACEMENT_3D('',#71511,#18063,#18064);
#14824=AXIS2_PLACEMENT_3D('',#71512,#18065,#18066);
#14825=AXIS2_PLACEMENT_3D('',#71518,#18070,#18071);
#14826=AXIS2_PLACEMENT_3D('',#71522,#18074,#18075);
#14827=AXIS2_PLACEMENT_3D('',#71523,#18076,#18077);
#14828=AXIS2_PLACEMENT_3D('',#71524,#18078,#18079);
#14829=AXIS2_PLACEMENT_3D('',#71526,#18081,#18082);
#14830=AXIS2_PLACEMENT_3D('',#71539,#18089,#18090);
#14831=AXIS2_PLACEMENT_3D('',#71543,#18092,#18093);
#14832=AXIS2_PLACEMENT_3D('',#71544,#18094,#18095);
#14833=AXIS2_PLACEMENT_3D('',#71547,#18097,#18098);
#14834=AXIS2_PLACEMENT_3D('',#71548,#18099,#18100);
#14835=AXIS2_PLACEMENT_3D('',#71551,#18102,#18103);
#14836=AXIS2_PLACEMENT_3D('',#71552,#18104,#18105);
#14837=AXIS2_PLACEMENT_3D('',#71555,#18107,#18108);
#14838=AXIS2_PLACEMENT_3D('',#71556,#18109,#18110);
#14839=AXIS2_PLACEMENT_3D('',#71559,#18112,#18113);
#14840=AXIS2_PLACEMENT_3D('',#71560,#18114,#18115);
#14841=AXIS2_PLACEMENT_3D('',#71562,#18117,#18118);
#14842=AXIS2_PLACEMENT_3D('',#71563,#18119,#18120);
#14843=AXIS2_PLACEMENT_3D('',#71566,#18122,#18123);
#14844=AXIS2_PLACEMENT_3D('',#71569,#18126,#18127);
#14845=AXIS2_PLACEMENT_3D('',#71571,#18129,#18130);
#14846=AXIS2_PLACEMENT_3D('',#71573,#18132,#18133);
#14847=AXIS2_PLACEMENT_3D('',#71575,#18135,#18136);
#14848=AXIS2_PLACEMENT_3D('',#71577,#18138,#18139);
#17446=DIRECTION('axis',(0.,0.,1.));
#17447=DIRECTION('refdir',(1.,0.,0.));
#17448=DIRECTION('center_axis',(0.,-1.,0.));
#17449=DIRECTION('ref_axis',(0.932069076459839,0.,-0.362280604928421));
#17450=DIRECTION('',(0.,1.,0.));
#17451=DIRECTION('center_axis',(0.,1.,0.));
#17452=DIRECTION('ref_axis',(1.,0.,9.69272361004426E-14));
#17453=DIRECTION('center_axis',(0.,-1.,0.));
#17454=DIRECTION('ref_axis',(0.932069076459839,0.,-0.362280604928421));
#17455=DIRECTION('',(0.,1.,0.));
#17456=DIRECTION('center_axis',(0.,-1.,0.));
#17457=DIRECTION('ref_axis',(0.932069076459839,0.,-0.362280604928421));
#17458=DIRECTION('',(0.,1.,0.));
#17459=DIRECTION('center_axis',(0.,-1.,0.));
#17460=DIRECTION('ref_axis',(0.932069076459839,0.,-0.362280604928421));
#17461=DIRECTION('',(0.,1.,0.));
#17462=DIRECTION('center_axis',(0.,-1.,0.));
#17463=DIRECTION('ref_axis',(0.932069076459839,0.,-0.362280604928421));
#17464=DIRECTION('',(0.,1.,0.));
#17465=DIRECTION('center_axis',(0.,-1.,0.));
#17466=DIRECTION('ref_axis',(0.932069076459839,0.,-0.362280604928421));
#17467=DIRECTION('',(0.,1.,0.));
#17468=DIRECTION('center_axis',(0.,-1.,0.));
#17469=DIRECTION('ref_axis',(0.932069076459839,0.,-0.362280604928421));
#17470=DIRECTION('',(0.,1.,0.));
#17471=DIRECTION('center_axis',(0.,-1.,0.));
#17472=DIRECTION('ref_axis',(0.932069076459839,0.,-0.362280604928421));
#17473=DIRECTION('',(0.,1.,0.));
#17474=DIRECTION('center_axis',(0.,-1.,0.));
#17475=DIRECTION('ref_axis',(0.932069076459839,0.,-0.362280604928421));
#17476=DIRECTION('',(0.,1.,0.));
#17477=DIRECTION('center_axis',(0.,-1.,0.));
#17478=DIRECTION('ref_axis',(0.932069076459839,0.,-0.362280604928421));
#17479=DIRECTION('',(0.,1.,0.));
#17480=DIRECTION('center_axis',(0.,-1.,0.));
#17481=DIRECTION('ref_axis',(0.932069076459839,0.,-0.362280604928421));
#17482=DIRECTION('',(0.,1.,0.));
#17483=DIRECTION('center_axis',(0.,-1.,0.));
#17484=DIRECTION('ref_axis',(0.932069076459839,0.,-0.362280604928421));
#17485=DIRECTION('',(0.,1.,0.));
#17486=DIRECTION('center_axis',(0.,-1.,0.));
#17487=DIRECTION('ref_axis',(0.932069076459839,0.,-0.362280604928421));
#17488=DIRECTION('',(0.,1.,0.));
#17489=DIRECTION('center_axis',(0.,-1.,0.));
#17490=DIRECTION('ref_axis',(0.932069076459839,0.,-0.362280604928421));
#17491=DIRECTION('',(0.,1.,0.));
#17492=DIRECTION('center_axis',(0.,-1.,0.));
#17493=DIRECTION('ref_axis',(1.,0.,0.));
#17494=DIRECTION('center_axis',(0.,1.,0.));
#17495=DIRECTION('ref_axis',(1.,0.,0.));
#17496=DIRECTION('center_axis',(0.,-1.,0.));
#17497=DIRECTION('ref_axis',(1.,0.,0.));
#17498=DIRECTION('center_axis',(0.,-1.,0.));
#17499=DIRECTION('ref_axis',(0.846353653806749,0.,-0.532621340811618));
#17500=DIRECTION('center_axis',(0.,-1.,0.));
#17501=DIRECTION('ref_axis',(1.,0.,9.69272361004426E-14));
#17502=DIRECTION('center_axis',(0.,1.,0.));
#17503=DIRECTION('ref_axis',(0.,0.,1.));
#17504=DIRECTION('center_axis',(0.,-1.,0.));
#17505=DIRECTION('ref_axis',(1.,0.,0.));
#17506=DIRECTION('center_axis',(0.,-1.,0.));
#17507=DIRECTION('ref_axis',(1.,0.,0.));
#17508=DIRECTION('center_axis',(0.,1.,0.));
#17509=DIRECTION('ref_axis',(0.,0.,1.));
#17510=DIRECTION('center_axis',(0.,1.,0.));
#17511=DIRECTION('ref_axis',(1.,0.,0.));
#17512=DIRECTION('center_axis',(0.,1.,0.));
#17513=DIRECTION('ref_axis',(1.,0.,0.));
#17514=DIRECTION('center_axis',(0.,1.,0.));
#17515=DIRECTION('ref_axis',(0.,0.,1.));
#17516=DIRECTION('center_axis',(0.,-1.,0.));
#17517=DIRECTION('ref_axis',(1.,0.,0.));
#17518=DIRECTION('center_axis',(1.,0.,0.));
#17519=DIRECTION('ref_axis',(0.,0.,-1.));
#17520=DIRECTION('center_axis',(0.,1.,0.));
#17521=DIRECTION('ref_axis',(1.,0.,0.));
#17522=DIRECTION('center_axis',(0.,1.,0.));
#17523=DIRECTION('ref_axis',(1.,0.,0.));
#17524=DIRECTION('center_axis',(0.,1.,0.));
#17525=DIRECTION('ref_axis',(1.,0.,0.));
#17526=DIRECTION('',(0.707106781186547,-0.707106781186548,-8.65956056235493E-17));
#17527=DIRECTION('center_axis',(0.,1.,0.));
#17528=DIRECTION('ref_axis',(1.,0.,0.));
#17529=DIRECTION('center_axis',(0.,1.,0.));
#17530=DIRECTION('ref_axis',(1.,0.,0.));
#17531=DIRECTION('center_axis',(-0.241286600017018,0.,0.970453902383945));
#17532=DIRECTION('ref_axis',(-0.970453902383945,0.,-0.241286600017018));
#17533=DIRECTION('',(0.,1.,0.));
#17534=DIRECTION('',(-0.970453902383945,0.,-0.241286600017018));
#17535=DIRECTION('',(0.,-1.,0.));
#17536=DIRECTION('center_axis',(-0.558650020314823,0.,-0.829403493362699));
#17537=DIRECTION('ref_axis',(0.829403493362699,0.,-0.558650020314823));
#17538=DIRECTION('',(0.,-1.,0.));
#17539=DIRECTION('',(0.829403493362699,0.,-0.558650020314823));
#17540=DIRECTION('center_axis',(0.,-1.,0.));
#17541=DIRECTION('ref_axis',(-0.17364817766693,0.,-0.984807753012208));
#17542=DIRECTION('center_axis',(0.,-1.,0.));
#17543=DIRECTION('ref_axis',(1.,0.,0.));
#17544=DIRECTION('center_axis',(0.,-1.,0.));
#17545=DIRECTION('ref_axis',(1.,0.,0.));
#17546=DIRECTION('center_axis',(0.,1.,0.));
#17547=DIRECTION('ref_axis',(1.,0.,0.));
#17548=DIRECTION('center_axis',(0.,1.,0.));
#17549=DIRECTION('ref_axis',(1.,0.,0.));
#17550=DIRECTION('center_axis',(0.,1.,0.));
#17551=DIRECTION('ref_axis',(1.,0.,0.));
#17552=DIRECTION('center_axis',(0.,1.,0.));
#17553=DIRECTION('ref_axis',(1.,0.,0.));
#17554=DIRECTION('center_axis',(0.,1.,0.));
#17555=DIRECTION('ref_axis',(1.,0.,0.));
#17556=DIRECTION('center_axis',(0.,1.,0.));
#17557=DIRECTION('ref_axis',(1.,0.,0.));
#17558=DIRECTION('center_axis',(0.,1.,0.));
#17559=DIRECTION('ref_axis',(1.,0.,0.));
#17560=DIRECTION('center_axis',(0.,1.,0.));
#17561=DIRECTION('ref_axis',(1.,0.,0.));
#17562=DIRECTION('center_axis',(0.,1.,0.));
#17563=DIRECTION('ref_axis',(1.,0.,0.));
#17564=DIRECTION('center_axis',(0.,1.,0.));
#17565=DIRECTION('ref_axis',(1.,0.,0.));
#17566=DIRECTION('center_axis',(0.,1.,0.));
#17567=DIRECTION('ref_axis',(1.,0.,0.));
#17568=DIRECTION('center_axis',(0.,1.,0.));
#17569=DIRECTION('ref_axis',(1.,0.,0.));
#17570=DIRECTION('center_axis',(0.,1.,0.));
#17571=DIRECTION('ref_axis',(1.,0.,0.));
#17572=DIRECTION('center_axis',(0.,1.,0.));
#17573=DIRECTION('ref_axis',(1.,0.,0.));
#17574=DIRECTION('center_axis',(0.,1.,0.));
#17575=DIRECTION('ref_axis',(1.,0.,0.));
#17576=DIRECTION('center_axis',(0.,1.,0.));
#17577=DIRECTION('ref_axis',(1.,0.,0.));
#17578=DIRECTION('center_axis',(0.,1.,0.));
#17579=DIRECTION('ref_axis',(1.,0.,0.));
#17580=DIRECTION('center_axis',(0.,1.,0.));
#17581=DIRECTION('ref_axis',(1.,0.,0.));
#17582=DIRECTION('center_axis',(0.,1.,0.));
#17583=DIRECTION('ref_axis',(1.,0.,0.));
#17584=DIRECTION('center_axis',(0.,1.,0.));
#17585=DIRECTION('ref_axis',(1.,0.,0.));
#17586=DIRECTION('center_axis',(0.,1.,0.));
#17587=DIRECTION('ref_axis',(1.,0.,0.));
#17588=DIRECTION('center_axis',(0.,1.,0.));
#17589=DIRECTION('ref_axis',(1.,0.,0.));
#17590=DIRECTION('center_axis',(0.,1.,0.));
#17591=DIRECTION('ref_axis',(1.,0.,0.));
#17592=DIRECTION('center_axis',(0.,1.,0.));
#17593=DIRECTION('ref_axis',(1.,0.,0.));
#17594=DIRECTION('center_axis',(0.,1.,0.));
#17595=DIRECTION('ref_axis',(1.,0.,0.));
#17596=DIRECTION('center_axis',(0.,1.,0.));
#17597=DIRECTION('ref_axis',(1.,0.,0.));
#17598=DIRECTION('center_axis',(0.,1.,0.));
#17599=DIRECTION('ref_axis',(1.,0.,0.));
#17600=DIRECTION('center_axis',(0.,1.,0.));
#17601=DIRECTION('ref_axis',(1.,0.,0.));
#17602=DIRECTION('center_axis',(0.,1.,0.));
#17603=DIRECTION('ref_axis',(1.,0.,0.));
#17604=DIRECTION('center_axis',(0.,1.,0.));
#17605=DIRECTION('ref_axis',(1.,0.,0.));
#17606=DIRECTION('center_axis',(0.,1.,0.));
#17607=DIRECTION('ref_axis',(1.,0.,0.));
#17608=DIRECTION('center_axis',(0.,1.,0.));
#17609=DIRECTION('ref_axis',(1.,0.,0.));
#17610=DIRECTION('center_axis',(0.,1.,0.));
#17611=DIRECTION('ref_axis',(1.,0.,0.));
#17612=DIRECTION('center_axis',(0.,1.,0.));
#17613=DIRECTION('ref_axis',(1.,0.,0.));
#17614=DIRECTION('center_axis',(0.,1.,0.));
#17615=DIRECTION('ref_axis',(1.,0.,0.));
#17616=DIRECTION('center_axis',(0.,1.,0.));
#17617=DIRECTION('ref_axis',(1.,0.,0.));
#17618=DIRECTION('',(0.707106781186547,0.707106781186548,8.65956056235493E-17));
#17619=DIRECTION('center_axis',(0.,-1.,0.));
#17620=DIRECTION('ref_axis',(1.,0.,0.));
#17621=DIRECTION('center_axis',(-0.0691033627359813,0.,0.997609505397066));
#17622=DIRECTION('ref_axis',(-0.997609505397066,0.,-0.0691033627359813));
#17623=DIRECTION('',(0.,1.,0.));
#17624=DIRECTION('',(-0.997609505397066,0.,-0.0691033627359813));
#17625=DIRECTION('',(0.,-1.,0.));
#17626=DIRECTION('center_axis',(-0.694187276399484,0.,-0.719794432657732));
#17627=DIRECTION('ref_axis',(0.719794432657732,0.,-0.694187276399484));
#17628=DIRECTION('',(0.,-1.,0.));
#17629=DIRECTION('',(0.719794432657732,0.,-0.694187276399484));
#17630=DIRECTION('center_axis',(0.,-1.,0.));
#17631=DIRECTION('ref_axis',(-0.342020143325669,0.,-0.939692620785908));
#17632=DIRECTION('center_axis',(0.,-1.,0.));
#17633=DIRECTION('ref_axis',(1.,0.,0.));
#17634=DIRECTION('center_axis',(0.105179545253799,0.,0.994453248403465));
#17635=DIRECTION('ref_axis',(-0.994453248403465,0.,0.105179545253799));
#17636=DIRECTION('',(0.,1.,0.));
#17637=DIRECTION('',(-0.994453248403465,0.,0.105179545253799));
#17638=DIRECTION('',(0.,-1.,0.));
#17639=DIRECTION('center_axis',(-0.808632003366458,0.,-0.588314782350018));
#17640=DIRECTION('ref_axis',(0.588314782350018,0.,-0.808632003366458));
#17641=DIRECTION('',(0.,-1.,0.));
#17642=DIRECTION('',(0.588314782350018,0.,-0.808632003366458));
#17643=DIRECTION('center_axis',(0.,-1.,0.));
#17644=DIRECTION('ref_axis',(-0.5,0.,-0.866025403784438));
#17645=DIRECTION('center_axis',(0.,-1.,0.));
#17646=DIRECTION('ref_axis',(1.,0.,0.));
#17647=DIRECTION('center_axis',(0.27626662598446,0.,0.961081032674749));
#17648=DIRECTION('ref_axis',(-0.961081032674749,0.,0.27626662598446));
#17649=DIRECTION('',(0.,1.,0.));
#17650=DIRECTION('',(-0.961081032674749,0.,0.27626662598446));
#17651=DIRECTION('',(0.,-1.,0.));
#17652=DIRECTION('center_axis',(-0.898506856098679,0.,-0.438959485082243));
#17653=DIRECTION('ref_axis',(0.438959485082243,0.,-0.898506856098679));
#17654=DIRECTION('',(0.,-1.,0.));
#17655=DIRECTION('',(0.438959485082243,0.,-0.898506856098679));
#17656=DIRECTION('center_axis',(0.,-1.,0.));
#17657=DIRECTION('ref_axis',(-0.64278760968654,0.,-0.766044443118978));
#17658=DIRECTION('center_axis',(0.,-1.,0.));
#17659=DIRECTION('ref_axis',(1.,0.,0.));
#17660=DIRECTION('center_axis',(0.438959485082242,0.,0.89850685609868));
#17661=DIRECTION('ref_axis',(-0.89850685609868,0.,0.438959485082242));
#17662=DIRECTION('',(0.,1.,0.));
#17663=DIRECTION('',(-0.89850685609868,0.,0.438959485082242));
#17664=DIRECTION('',(0.,-1.,0.));
#17665=DIRECTION('center_axis',(-0.961081032674749,0.,-0.276266625984462));
#17666=DIRECTION('ref_axis',(0.276266625984462,0.,-0.961081032674749));
#17667=DIRECTION('',(0.,-1.,0.));
#17668=DIRECTION('',(0.276266625984462,0.,-0.961081032674749));
#17669=DIRECTION('center_axis',(0.,-1.,0.));
#17670=DIRECTION('ref_axis',(-0.766044443118978,0.,-0.642787609686539));
#17671=DIRECTION('center_axis',(0.,-1.,0.));
#17672=DIRECTION('ref_axis',(1.,0.,0.));
#17673=DIRECTION('center_axis',(0.588314782350017,0.,0.808632003366459));
#17674=DIRECTION('ref_axis',(-0.808632003366459,0.,0.588314782350017));
#17675=DIRECTION('',(0.,1.,0.));
#17676=DIRECTION('',(-0.808632003366459,0.,0.588314782350017));
#17677=DIRECTION('',(0.,-1.,0.));
#17678=DIRECTION('center_axis',(-0.994453248403465,0.,-0.1051795452538));
#17679=DIRECTION('ref_axis',(0.1051795452538,0.,-0.994453248403465));
#17680=DIRECTION('',(0.,-1.,0.));
#17681=DIRECTION('',(0.1051795452538,0.,-0.994453248403465));
#17682=DIRECTION('center_axis',(0.,-1.,0.));
#17683=DIRECTION('ref_axis',(-0.866025403784439,0.,-0.5));
#17684=DIRECTION('center_axis',(0.,-1.,0.));
#17685=DIRECTION('ref_axis',(1.,0.,0.));
#17686=DIRECTION('center_axis',(0.719794432657731,0.,0.694187276399485));
#17687=DIRECTION('ref_axis',(-0.694187276399485,0.,0.719794432657731));
#17688=DIRECTION('',(0.,1.,0.));
#17689=DIRECTION('',(-0.694187276399485,0.,0.719794432657731));
#17690=DIRECTION('',(0.,-1.,0.));
#17691=DIRECTION('center_axis',(-0.997609505397066,0.,0.0691033627359807));
#17692=DIRECTION('ref_axis',(-0.0691033627359807,0.,-0.997609505397066));
#17693=DIRECTION('',(0.,-1.,0.));
#17694=DIRECTION('',(-0.0691033627359807,0.,-0.997609505397066));
#17695=DIRECTION('center_axis',(0.,-1.,0.));
#17696=DIRECTION('ref_axis',(-0.939692620785909,0.,-0.342020143325668));
#17697=DIRECTION('center_axis',(0.,-1.,0.));
#17698=DIRECTION('ref_axis',(1.,0.,0.));
#17699=DIRECTION('center_axis',(0.829403493362698,0.,0.558650020314824));
#17700=DIRECTION('ref_axis',(-0.558650020314824,0.,0.829403493362698));
#17701=DIRECTION('',(0.,1.,0.));
#17702=DIRECTION('',(-0.558650020314824,0.,0.829403493362698));
#17703=DIRECTION('',(0.,-1.,0.));
#17704=DIRECTION('center_axis',(-0.970453902383945,0.,0.241286600017017));
#17705=DIRECTION('ref_axis',(-0.241286600017017,0.,-0.970453902383945));
#17706=DIRECTION('',(0.,-1.,0.));
#17707=DIRECTION('',(-0.241286600017017,0.,-0.970453902383945));
#17708=DIRECTION('center_axis',(0.,-1.,0.));
#17709=DIRECTION('ref_axis',(-0.984807753012208,0.,-0.17364817766693));
#17710=DIRECTION('center_axis',(0.,-1.,0.));
#17711=DIRECTION('ref_axis',(1.,0.,0.));
#17712=DIRECTION('center_axis',(0.913811548620257,0.,0.406138466053448));
#17713=DIRECTION('ref_axis',(-0.406138466053448,0.,0.913811548620257));
#17714=DIRECTION('',(0.,1.,0.));
#17715=DIRECTION('',(-0.406138466053448,0.,0.913811548620257));
#17716=DIRECTION('',(0.,-1.,0.));
#17717=DIRECTION('center_axis',(-0.913811548620258,0.,0.406138466053447));
#17718=DIRECTION('ref_axis',(-0.406138466053447,0.,-0.913811548620258));
#17719=DIRECTION('',(0.,-1.,0.));
#17720=DIRECTION('',(-0.406138466053447,0.,-0.913811548620257));
#17721=DIRECTION('center_axis',(0.,-1.,0.));
#17722=DIRECTION('ref_axis',(-1.,0.,1.83697019872103E-16));
#17723=DIRECTION('center_axis',(0.,-1.,0.));
#17724=DIRECTION('ref_axis',(1.,0.,0.));
#17725=DIRECTION('center_axis',(0.970453902383945,0.,0.241286600017018));
#17726=DIRECTION('ref_axis',(-0.241286600017018,0.,0.970453902383945));
#17727=DIRECTION('',(0.,1.,0.));
#17728=DIRECTION('',(-0.241286600017018,0.,0.970453902383945));
#17729=DIRECTION('',(0.,-1.,0.));
#17730=DIRECTION('center_axis',(-0.829403493362699,0.,0.558650020314823));
#17731=DIRECTION('ref_axis',(-0.558650020314823,0.,-0.829403493362699));
#17732=DIRECTION('',(0.,-1.,0.));
#17733=DIRECTION('',(-0.558650020314823,0.,-0.829403493362699));
#17734=DIRECTION('center_axis',(0.,-1.,0.));
#17735=DIRECTION('ref_axis',(-0.984807753012208,0.,0.17364817766693));
#17736=DIRECTION('center_axis',(0.,-1.,0.));
#17737=DIRECTION('ref_axis',(1.,0.,0.));
#17738=DIRECTION('center_axis',(0.997609505397066,0.,0.0691033627359814));
#17739=DIRECTION('ref_axis',(-0.0691033627359814,0.,0.997609505397066));
#17740=DIRECTION('',(0.,1.,0.));
#17741=DIRECTION('',(-0.0691033627359814,0.,0.997609505397066));
#17742=DIRECTION('',(0.,-1.,0.));
#17743=DIRECTION('center_axis',(-0.719794432657732,0.,0.694187276399484));
#17744=DIRECTION('ref_axis',(-0.694187276399484,0.,-0.719794432657732));
#17745=DIRECTION('',(0.,-1.,0.));
#17746=DIRECTION('',(-0.694187276399484,0.,-0.719794432657732));
#17747=DIRECTION('center_axis',(0.,-1.,0.));
#17748=DIRECTION('ref_axis',(-0.939692620785908,0.,0.342020143325669));
#17749=DIRECTION('center_axis',(0.,-1.,0.));
#17750=DIRECTION('ref_axis',(1.,0.,0.));
#17751=DIRECTION('center_axis',(0.994453248403465,0.,-0.105179545253799));
#17752=DIRECTION('ref_axis',(0.105179545253799,0.,0.994453248403465));
#17753=DIRECTION('',(0.,1.,0.));
#17754=DIRECTION('',(0.105179545253799,0.,0.994453248403465));
#17755=DIRECTION('',(0.,-1.,0.));
#17756=DIRECTION('center_axis',(-0.588314782350018,0.,0.808632003366458));
#17757=DIRECTION('ref_axis',(-0.808632003366458,0.,-0.588314782350018));
#17758=DIRECTION('',(0.,-1.,0.));
#17759=DIRECTION('',(-0.808632003366458,0.,-0.588314782350018));
#17760=DIRECTION('center_axis',(0.,-1.,0.));
#17761=DIRECTION('ref_axis',(-0.866025403784438,0.,0.5));
#17762=DIRECTION('center_axis',(0.,-1.,0.));
#17763=DIRECTION('ref_axis',(1.,0.,0.));
#17764=DIRECTION('center_axis',(0.961081032674749,0.,-0.27626662598446));
#17765=DIRECTION('ref_axis',(0.27626662598446,0.,0.961081032674749));
#17766=DIRECTION('',(0.,1.,0.));
#17767=DIRECTION('',(0.27626662598446,0.,0.961081032674749));
#17768=DIRECTION('',(0.,-1.,0.));
#17769=DIRECTION('center_axis',(-0.438959485082243,0.,0.898506856098679));
#17770=DIRECTION('ref_axis',(-0.898506856098679,0.,-0.438959485082243));
#17771=DIRECTION('',(0.,-1.,0.));
#17772=DIRECTION('',(-0.898506856098679,0.,-0.438959485082243));
#17773=DIRECTION('center_axis',(0.,-1.,0.));
#17774=DIRECTION('ref_axis',(-0.766044443118978,0.,0.642787609686539));
#17775=DIRECTION('center_axis',(0.,-1.,0.));
#17776=DIRECTION('ref_axis',(1.,0.,0.));
#17777=DIRECTION('center_axis',(0.89850685609868,0.,-0.438959485082242));
#17778=DIRECTION('ref_axis',(0.438959485082242,0.,0.89850685609868));
#17779=DIRECTION('',(0.,1.,0.));
#17780=DIRECTION('',(0.438959485082242,0.,0.89850685609868));
#17781=DIRECTION('',(0.,-1.,0.));
#17782=DIRECTION('center_axis',(-0.276266625984462,0.,0.961081032674749));
#17783=DIRECTION('ref_axis',(-0.961081032674749,0.,-0.276266625984462));
#17784=DIRECTION('',(0.,-1.,0.));
#17785=DIRECTION('',(-0.961081032674749,0.,-0.276266625984462));
#17786=DIRECTION('center_axis',(0.,-1.,0.));
#17787=DIRECTION('ref_axis',(-0.642787609686539,0.,0.766044443118978));
#17788=DIRECTION('center_axis',(0.,-1.,0.));
#17789=DIRECTION('ref_axis',(1.,0.,0.));
#17790=DIRECTION('center_axis',(0.808632003366458,0.,-0.588314782350017));
#17791=DIRECTION('ref_axis',(0.588314782350017,0.,0.808632003366458));
#17792=DIRECTION('',(0.,1.,0.));
#17793=DIRECTION('',(0.588314782350017,0.,0.808632003366458));
#17794=DIRECTION('',(0.,-1.,0.));
#17795=DIRECTION('center_axis',(-0.1051795452538,0.,0.994453248403465));
#17796=DIRECTION('ref_axis',(-0.994453248403465,0.,-0.1051795452538));
#17797=DIRECTION('',(0.,-1.,0.));
#17798=DIRECTION('',(-0.994453248403465,0.,-0.1051795452538));
#17799=DIRECTION('center_axis',(0.,-1.,0.));
#17800=DIRECTION('ref_axis',(-0.5,0.,0.866025403784439));
#17801=DIRECTION('center_axis',(0.,-1.,0.));
#17802=DIRECTION('ref_axis',(1.,0.,0.));
#17803=DIRECTION('center_axis',(0.694187276399485,0.,-0.719794432657731));
#17804=DIRECTION('ref_axis',(0.719794432657731,0.,0.694187276399485));
#17805=DIRECTION('',(0.,1.,0.));
#17806=DIRECTION('',(0.719794432657731,0.,0.694187276399485));
#17807=DIRECTION('',(0.,-1.,0.));
#17808=DIRECTION('center_axis',(0.0691033627359802,0.,0.997609505397066));
#17809=DIRECTION('ref_axis',(-0.997609505397067,0.,0.0691033627359802));
#17810=DIRECTION('',(0.,-1.,0.));
#17811=DIRECTION('',(-0.997609505397066,0.,0.0691033627359802));
#17812=DIRECTION('center_axis',(0.,-1.,0.));
#17813=DIRECTION('ref_axis',(-0.342020143325669,0.,0.939692620785908));
#17814=DIRECTION('center_axis',(0.,-1.,0.));
#17815=DIRECTION('ref_axis',(1.,0.,0.));
#17816=DIRECTION('center_axis',(0.558650020314824,0.,-0.829403493362698));
#17817=DIRECTION('ref_axis',(0.829403493362698,0.,0.558650020314824));
#17818=DIRECTION('',(0.,1.,0.));
#17819=DIRECTION('',(0.829403493362698,0.,0.558650020314824));
#17820=DIRECTION('',(0.,-1.,0.));
#17821=DIRECTION('center_axis',(0.241286600017017,0.,0.970453902383945));
#17822=DIRECTION('ref_axis',(-0.970453902383945,0.,0.241286600017017));
#17823=DIRECTION('',(0.,-1.,0.));
#17824=DIRECTION('',(-0.970453902383945,0.,0.241286600017017));
#17825=DIRECTION('center_axis',(0.,-1.,0.));
#17826=DIRECTION('ref_axis',(-0.17364817766693,0.,0.984807753012208));
#17827=DIRECTION('center_axis',(0.,-1.,0.));
#17828=DIRECTION('ref_axis',(1.,0.,0.));
#17829=DIRECTION('center_axis',(0.406138466053448,0.,-0.913811548620257));
#17830=DIRECTION('ref_axis',(0.913811548620257,0.,0.406138466053448));
#17831=DIRECTION('',(0.,1.,0.));
#17832=DIRECTION('',(0.913811548620257,0.,0.406138466053448));
#17833=DIRECTION('',(0.,-1.,0.));
#17834=DIRECTION('center_axis',(0.406138466053447,0.,0.913811548620258));
#17835=DIRECTION('ref_axis',(-0.913811548620258,0.,0.406138466053447));
#17836=DIRECTION('',(0.,-1.,0.));
#17837=DIRECTION('',(-0.913811548620257,0.,0.406138466053447));
#17838=DIRECTION('center_axis',(0.,-1.,0.));
#17839=DIRECTION('ref_axis',(1.22464679914735E-16,0.,1.));
#17840=DIRECTION('center_axis',(0.,-1.,0.));
#17841=DIRECTION('ref_axis',(1.,0.,0.));
#17842=DIRECTION('center_axis',(0.,-1.,0.));
#17843=DIRECTION('ref_axis',(1.,0.,0.));
#17844=DIRECTION('center_axis',(0.241286600017018,0.,-0.970453902383945));
#17845=DIRECTION('ref_axis',(0.970453902383945,0.,0.241286600017018));
#17846=DIRECTION('',(0.,1.,0.));
#17847=DIRECTION('',(0.970453902383945,0.,0.241286600017018));
#17848=DIRECTION('',(0.,-1.,0.));
#17849=DIRECTION('center_axis',(0.558650020314823,0.,0.829403493362698));
#17850=DIRECTION('ref_axis',(-0.829403493362698,0.,0.558650020314823));
#17851=DIRECTION('',(0.,-1.,0.));
#17852=DIRECTION('',(-0.829403493362698,0.,0.558650020314823));
#17853=DIRECTION('center_axis',(0.,-1.,0.));
#17854=DIRECTION('ref_axis',(0.173648177666931,0.,0.984807753012208));
#17855=DIRECTION('center_axis',(0.,-1.,0.));
#17856=DIRECTION('ref_axis',(1.,0.,0.));
#17857=DIRECTION('center_axis',(0.0691033627359819,0.,-0.997609505397066));
#17858=DIRECTION('ref_axis',(0.997609505397066,0.,0.0691033627359819));
#17859=DIRECTION('',(0.,1.,0.));
#17860=DIRECTION('',(0.997609505397066,0.,0.0691033627359819));
#17861=DIRECTION('',(0.,-1.,0.));
#17862=DIRECTION('center_axis',(0.694187276399484,0.,0.719794432657732));
#17863=DIRECTION('ref_axis',(-0.719794432657732,0.,0.694187276399484));
#17864=DIRECTION('',(0.,-1.,0.));
#17865=DIRECTION('',(-0.719794432657732,0.,0.694187276399484));
#17866=DIRECTION('center_axis',(0.,-1.,0.));
#17867=DIRECTION('ref_axis',(0.342020143325669,0.,0.939692620785908));
#17868=DIRECTION('center_axis',(0.,-1.,0.));
#17869=DIRECTION('ref_axis',(1.,0.,0.));
#17870=DIRECTION('center_axis',(-0.105179545253798,0.,-0.994453248403465));
#17871=DIRECTION('ref_axis',(0.994453248403465,0.,-0.105179545253798));
#17872=DIRECTION('',(0.,1.,0.));
#17873=DIRECTION('',(0.994453248403465,0.,-0.105179545253798));
#17874=DIRECTION('',(0.,-1.,0.));
#17875=DIRECTION('center_axis',(0.808632003366457,0.,0.588314782350019));
#17876=DIRECTION('ref_axis',(-0.588314782350019,0.,0.808632003366457));
#17877=DIRECTION('',(0.,-1.,0.));
#17878=DIRECTION('',(-0.588314782350019,0.,0.808632003366457));
#17879=DIRECTION('center_axis',(0.,-1.,0.));
#17880=DIRECTION('ref_axis',(0.5,0.,0.866025403784439));
#17881=DIRECTION('center_axis',(0.,-1.,0.));
#17882=DIRECTION('ref_axis',(1.,0.,0.));
#17883=DIRECTION('center_axis',(-0.27626662598446,0.,-0.961081032674749));
#17884=DIRECTION('ref_axis',(0.961081032674749,0.,-0.27626662598446));
#17885=DIRECTION('',(0.,1.,0.));
#17886=DIRECTION('',(0.961081032674749,0.,-0.27626662598446));
#17887=DIRECTION('',(0.,-1.,0.));
#17888=DIRECTION('center_axis',(0.898506856098679,0.,0.438959485082243));
#17889=DIRECTION('ref_axis',(-0.438959485082243,0.,0.898506856098679));
#17890=DIRECTION('',(0.,-1.,0.));
#17891=DIRECTION('',(-0.438959485082243,0.,0.898506856098679));
#17892=DIRECTION('center_axis',(0.,-1.,0.));
#17893=DIRECTION('ref_axis',(0.642787609686539,0.,0.766044443118978));
#17894=DIRECTION('center_axis',(0.,-1.,0.));
#17895=DIRECTION('ref_axis',(1.,0.,0.));
#17896=DIRECTION('center_axis',(-0.438959485082242,0.,-0.89850685609868));
#17897=DIRECTION('ref_axis',(0.89850685609868,0.,-0.438959485082242));
#17898=DIRECTION('',(0.,1.,0.));
#17899=DIRECTION('',(0.89850685609868,0.,-0.438959485082242));
#17900=DIRECTION('',(0.,-1.,0.));
#17901=DIRECTION('center_axis',(0.961081032674749,0.,0.276266625984462));
#17902=DIRECTION('ref_axis',(-0.276266625984462,0.,0.961081032674749));
#17903=DIRECTION('',(0.,-1.,0.));
#17904=DIRECTION('',(-0.276266625984462,0.,0.961081032674749));
#17905=DIRECTION('center_axis',(0.,-1.,0.));
#17906=DIRECTION('ref_axis',(0.766044443118978,0.,0.642787609686539));
#17907=DIRECTION('center_axis',(0.,-1.,0.));
#17908=DIRECTION('ref_axis',(1.,0.,0.));
#17909=DIRECTION('center_axis',(-0.588314782350017,0.,-0.808632003366458));
#17910=DIRECTION('ref_axis',(0.808632003366458,0.,-0.588314782350017));
#17911=DIRECTION('',(0.,1.,0.));
#17912=DIRECTION('',(0.808632003366458,0.,-0.588314782350017));
#17913=DIRECTION('',(0.,-1.,0.));
#17914=DIRECTION('center_axis',(0.994453248403465,0.,0.1051795452538));
#17915=DIRECTION('ref_axis',(-0.1051795452538,0.,0.994453248403465));
#17916=DIRECTION('',(0.,-1.,0.));
#17917=DIRECTION('',(-0.1051795452538,0.,0.994453248403465));
#17918=DIRECTION('center_axis',(0.,-1.,0.));
#17919=DIRECTION('ref_axis',(0.866025403784439,0.,0.5));
#17920=DIRECTION('center_axis',(0.,-1.,0.));
#17921=DIRECTION('ref_axis',(1.,0.,0.));
#17922=DIRECTION('center_axis',(-0.719794432657731,0.,-0.694187276399485));
#17923=DIRECTION('ref_axis',(0.694187276399485,0.,-0.719794432657731));
#17924=DIRECTION('',(0.,1.,0.));
#17925=DIRECTION('',(0.694187276399485,0.,-0.719794432657731));
#17926=DIRECTION('',(0.,-1.,0.));
#17927=DIRECTION('center_axis',(0.997609505397066,0.,-0.0691033627359801));
#17928=DIRECTION('ref_axis',(0.0691033627359801,0.,0.997609505397067));
#17929=DIRECTION('',(0.,-1.,0.));
#17930=DIRECTION('',(0.0691033627359801,0.,0.997609505397066));
#17931=DIRECTION('center_axis',(0.,-1.,0.));
#17932=DIRECTION('ref_axis',(0.939692620785908,0.,0.342020143325669));
#17933=DIRECTION('center_axis',(0.,-1.,0.));
#17934=DIRECTION('ref_axis',(1.,0.,0.));
#17935=DIRECTION('center_axis',(-0.829403493362697,0.,-0.558650020314825));
#17936=DIRECTION('ref_axis',(0.558650020314825,0.,-0.829403493362697));
#17937=DIRECTION('',(0.,1.,0.));
#17938=DIRECTION('',(0.558650020314825,0.,-0.829403493362697));
#17939=DIRECTION('',(0.,-1.,0.));
#17940=DIRECTION('center_axis',(0.970453902383946,0.,-0.241286600017016));
#17941=DIRECTION('ref_axis',(0.241286600017016,0.,0.970453902383946));
#17942=DIRECTION('',(0.,-1.,0.));
#17943=DIRECTION('',(0.241286600017016,0.,0.970453902383946));
#17944=DIRECTION('center_axis',(0.,-1.,0.));
#17945=DIRECTION('ref_axis',(0.984807753012208,0.,0.17364817766693));
#17946=DIRECTION('center_axis',(0.,-1.,0.));
#17947=DIRECTION('ref_axis',(1.,0.,0.));
#17948=DIRECTION('center_axis',(-0.913811548620257,0.,-0.406138466053448));
#17949=DIRECTION('ref_axis',(0.406138466053448,0.,-0.913811548620257));
#17950=DIRECTION('',(0.,1.,0.));
#17951=DIRECTION('',(0.406138466053448,0.,-0.913811548620257));
#17952=DIRECTION('',(0.,-1.,0.));
#17953=DIRECTION('center_axis',(0.913811548620258,0.,-0.406138466053447));
#17954=DIRECTION('ref_axis',(0.406138466053447,0.,0.913811548620258));
#17955=DIRECTION('',(0.,-1.,0.));
#17956=DIRECTION('',(0.406138466053447,0.,0.913811548620257));
#17957=DIRECTION('center_axis',(0.,-1.,0.));
#17958=DIRECTION('ref_axis',(1.,0.,-6.12323399573677E-17));
#17959=DIRECTION('center_axis',(0.,-1.,0.));
#17960=DIRECTION('ref_axis',(1.,0.,0.));
#17961=DIRECTION('center_axis',(-0.970453902383945,0.,-0.241286600017018));
#17962=DIRECTION('ref_axis',(0.241286600017018,0.,-0.970453902383945));
#17963=DIRECTION('',(0.,1.,0.));
#17964=DIRECTION('',(0.241286600017018,0.,-0.970453902383945));
#17965=DIRECTION('',(0.,-1.,0.));
#17966=DIRECTION('center_axis',(0.829403493362699,0.,-0.558650020314823));
#17967=DIRECTION('ref_axis',(0.558650020314823,0.,0.829403493362699));
#17968=DIRECTION('',(0.,-1.,0.));
#17969=DIRECTION('',(0.558650020314823,0.,0.829403493362699));
#17970=DIRECTION('center_axis',(0.,-1.,0.));
#17971=DIRECTION('ref_axis',(0.984807753012208,0.,-0.17364817766693));
#17972=DIRECTION('center_axis',(0.,-1.,0.));
#17973=DIRECTION('ref_axis',(1.,0.,0.));
#17974=DIRECTION('center_axis',(-0.997609505397066,0.,-0.069103362735982));
#17975=DIRECTION('ref_axis',(0.069103362735982,0.,-0.997609505397066));
#17976=DIRECTION('',(0.,1.,0.));
#17977=DIRECTION('',(0.069103362735982,0.,-0.997609505397066));
#17978=DIRECTION('',(0.,-1.,0.));
#17979=DIRECTION('center_axis',(0.719794432657732,0.,-0.694187276399484));
#17980=DIRECTION('ref_axis',(0.694187276399484,0.,0.719794432657732));
#17981=DIRECTION('',(0.,-1.,0.));
#17982=DIRECTION('',(0.694187276399484,0.,0.719794432657732));
#17983=DIRECTION('center_axis',(0.,-1.,0.));
#17984=DIRECTION('ref_axis',(0.939692620785908,0.,-0.342020143325669));
#17985=DIRECTION('center_axis',(0.,-1.,0.));
#17986=DIRECTION('ref_axis',(1.,0.,0.));
#17987=DIRECTION('center_axis',(-0.994453248403465,0.,0.105179545253798));
#17988=DIRECTION('ref_axis',(-0.105179545253798,0.,-0.994453248403465));
#17989=DIRECTION('',(0.,1.,0.));
#17990=DIRECTION('',(-0.105179545253798,0.,-0.994453248403465));
#17991=DIRECTION('',(0.,-1.,0.));
#17992=DIRECTION('center_axis',(0.588314782350018,0.,-0.808632003366458));
#17993=DIRECTION('ref_axis',(0.808632003366458,0.,0.588314782350018));
#17994=DIRECTION('',(0.,-1.,0.));
#17995=DIRECTION('',(0.808632003366457,0.,0.588314782350018));
#17996=DIRECTION('center_axis',(0.,-1.,0.));
#17997=DIRECTION('ref_axis',(0.866025403784439,0.,-0.5));
#17998=DIRECTION('center_axis',(0.,-1.,0.));
#17999=DIRECTION('ref_axis',(1.,0.,0.));
#18000=DIRECTION('center_axis',(-0.961081032674749,0.,0.27626662598446));
#18001=DIRECTION('ref_axis',(-0.27626662598446,0.,-0.961081032674749));
#18002=DIRECTION('',(0.,1.,0.));
#18003=DIRECTION('',(-0.27626662598446,0.,-0.961081032674749));
#18004=DIRECTION('',(0.,-1.,0.));
#18005=DIRECTION('center_axis',(0.438959485082244,0.,-0.898506856098679));
#18006=DIRECTION('ref_axis',(0.898506856098679,0.,0.438959485082244));
#18007=DIRECTION('',(0.,-1.,0.));
#18008=DIRECTION('',(0.898506856098678,0.,0.438959485082244));
#18009=DIRECTION('center_axis',(0.,-1.,0.));
#18010=DIRECTION('ref_axis',(0.766044443118978,0.,-0.642787609686539));
#18011=DIRECTION('center_axis',(0.,-1.,0.));
#18012=DIRECTION('ref_axis',(1.,0.,0.));
#18013=DIRECTION('center_axis',(-0.89850685609868,0.,0.438959485082242));
#18014=DIRECTION('ref_axis',(-0.438959485082242,0.,-0.89850685609868));
#18015=DIRECTION('',(0.,1.,0.));
#18016=DIRECTION('',(-0.438959485082242,0.,-0.89850685609868));
#18017=DIRECTION('',(0.,-1.,0.));
#18018=DIRECTION('center_axis',(0.276266625984462,0.,-0.961081032674749));
#18019=DIRECTION('ref_axis',(0.961081032674749,0.,0.276266625984462));
#18020=DIRECTION('',(0.,-1.,0.));
#18021=DIRECTION('',(0.961081032674749,0.,0.276266625984462));
#18022=DIRECTION('center_axis',(0.,-1.,0.));
#18023=DIRECTION('ref_axis',(0.642787609686539,0.,-0.766044443118978));
#18024=DIRECTION('center_axis',(0.,-1.,0.));
#18025=DIRECTION('ref_axis',(1.,0.,0.));
#18026=DIRECTION('center_axis',(-0.808632003366459,0.,0.588314782350017));
#18027=DIRECTION('ref_axis',(-0.588314782350017,0.,-0.808632003366459));
#18028=DIRECTION('',(0.,1.,0.));
#18029=DIRECTION('',(-0.588314782350017,0.,-0.808632003366458));
#18030=DIRECTION('',(0.,-1.,0.));
#18031=DIRECTION('center_axis',(0.1051795452538,0.,-0.994453248403465));
#18032=DIRECTION('ref_axis',(0.994453248403465,0.,0.1051795452538));
#18033=DIRECTION('',(0.,-1.,0.));
#18034=DIRECTION('',(0.994453248403465,0.,0.1051795452538));
#18035=DIRECTION('center_axis',(0.,-1.,0.));
#18036=DIRECTION('ref_axis',(0.5,0.,-0.866025403784439));
#18037=DIRECTION('center_axis',(0.,-1.,0.));
#18038=DIRECTION('ref_axis',(1.,0.,0.));
#18039=DIRECTION('center_axis',(-0.694187276399485,0.,0.719794432657731));
#18040=DIRECTION('ref_axis',(-0.719794432657731,0.,-0.694187276399485));
#18041=DIRECTION('',(0.,1.,0.));
#18042=DIRECTION('',(-0.719794432657731,0.,-0.694187276399485));
#18043=DIRECTION('',(0.,-1.,0.));
#18044=DIRECTION('center_axis',(-0.0691033627359801,0.,-0.997609505397066));
#18045=DIRECTION('ref_axis',(0.997609505397067,0.,-0.0691033627359801));
#18046=DIRECTION('',(0.,-1.,0.));
#18047=DIRECTION('',(0.997609505397066,0.,-0.0691033627359801));
#18048=DIRECTION('center_axis',(0.,-1.,0.));
#18049=DIRECTION('ref_axis',(0.342020143325669,0.,-0.939692620785908));
#18050=DIRECTION('center_axis',(0.,-1.,0.));
#18051=DIRECTION('ref_axis',(1.,0.,0.));
#18052=DIRECTION('center_axis',(-0.558650020314825,0.,0.829403493362697));
#18053=DIRECTION('ref_axis',(-0.829403493362697,0.,-0.558650020314825));
#18054=DIRECTION('',(0.,1.,0.));
#18055=DIRECTION('',(-0.829403493362697,0.,-0.558650020314825));
#18056=DIRECTION('',(0.,-1.,0.));
#18057=DIRECTION('center_axis',(-0.241286600017016,0.,-0.970453902383946));
#18058=DIRECTION('ref_axis',(0.970453902383946,0.,-0.241286600017016));
#18059=DIRECTION('',(0.,-1.,0.));
#18060=DIRECTION('',(0.970453902383946,0.,-0.241286600017016));
#18061=DIRECTION('center_axis',(0.,-1.,0.));
#18062=DIRECTION('ref_axis',(0.17364817766693,0.,-0.984807753012208));
#18063=DIRECTION('center_axis',(0.,-1.,0.));
#18064=DIRECTION('ref_axis',(1.,0.,0.));
#18065=DIRECTION('center_axis',(-0.406138466053448,0.,0.913811548620257));
#18066=DIRECTION('ref_axis',(-0.913811548620257,0.,-0.406138466053448));
#18067=DIRECTION('',(0.,1.,0.));
#18068=DIRECTION('',(-0.913811548620257,0.,-0.406138466053448));
#18069=DIRECTION('',(0.,-1.,0.));
#18070=DIRECTION('center_axis',(-0.406138466053447,0.,-0.913811548620258));
#18071=DIRECTION('ref_axis',(0.913811548620258,0.,-0.406138466053447));
#18072=DIRECTION('',(0.,-1.,0.));
#18073=DIRECTION('',(0.913811548620257,0.,-0.406138466053447));
#18074=DIRECTION('center_axis',(0.,-1.,0.));
#18075=DIRECTION('ref_axis',(0.,0.,-1.));
#18076=DIRECTION('center_axis',(0.,-1.,0.));
#18077=DIRECTION('ref_axis',(1.,0.,0.));
#18078=DIRECTION('center_axis',(0.,1.,0.));
#18079=DIRECTION('ref_axis',(1.,0.,0.));
#18080=DIRECTION('',(0.,-1.,0.));
#18081=DIRECTION('center_axis',(0.,1.,0.));
#18082=DIRECTION('ref_axis',(1.,0.,0.));
#18083=DIRECTION('',(0.499999999999999,0.,-0.866025403784439));
#18084=DIRECTION('',(1.,0.,0.));
#18085=DIRECTION('',(0.5,0.,0.866025403784438));
#18086=DIRECTION('',(-0.5,0.,0.866025403784439));
#18087=DIRECTION('',(-1.,0.,0.));
#18088=DIRECTION('',(-0.500000000000001,0.,-0.866025403784438));
#18089=DIRECTION('center_axis',(0.,1.,0.));
#18090=DIRECTION('ref_axis',(0.,0.,1.));
#18091=DIRECTION('',(0.499999999999999,0.,-0.866025403784439));
#18092=DIRECTION('center_axis',(0.,-1.,0.));
#18093=DIRECTION('ref_axis',(1.,0.,0.));
#18094=DIRECTION('center_axis',(0.,1.,0.));
#18095=DIRECTION('ref_axis',(0.,0.,1.));
#18096=DIRECTION('',(1.,0.,0.));
#18097=DIRECTION('center_axis',(0.,-1.,0.));
#18098=DIRECTION('ref_axis',(1.,0.,0.));
#18099=DIRECTION('center_axis',(0.,1.,0.));
#18100=DIRECTION('ref_axis',(0.,0.,1.));
#18101=DIRECTION('',(0.5,0.,0.866025403784438));
#18102=DIRECTION('center_axis',(0.,-1.,0.));
#18103=DIRECTION('ref_axis',(1.,0.,0.));
#18104=DIRECTION('center_axis',(0.,1.,0.));
#18105=DIRECTION('ref_axis',(0.,0.,1.));
#18106=DIRECTION('',(-0.5,0.,0.866025403784439));
#18107=DIRECTION('center_axis',(0.,-1.,0.));
#18108=DIRECTION('ref_axis',(1.,0.,0.));
#18109=DIRECTION('center_axis',(0.,1.,0.));
#18110=DIRECTION('ref_axis',(0.,0.,1.));
#18111=DIRECTION('',(-1.,0.,0.));
#18112=DIRECTION('center_axis',(0.,-1.,0.));
#18113=DIRECTION('ref_axis',(1.,0.,0.));
#18114=DIRECTION('center_axis',(0.,1.,0.));
#18115=DIRECTION('ref_axis',(0.,0.,1.));
#18116=DIRECTION('',(-0.500000000000001,0.,-0.866025403784438));
#18117=DIRECTION('center_axis',(0.,-1.,0.));
#18118=DIRECTION('ref_axis',(1.,0.,0.));
#18119=DIRECTION('center_axis',(0.,1.,0.));
#18120=DIRECTION('ref_axis',(1.,0.,0.));
#18121=DIRECTION('',(-0.85716730070211,0.515038074910058,1.04972719113862E-16));
#18122=DIRECTION('center_axis',(-0.866025403784439,0.,-0.499999999999999));
#18123=DIRECTION('ref_axis',(0.499999999999999,0.,-0.866025403784439));
#18124=DIRECTION('',(0.,-1.,0.));
#18125=DIRECTION('',(0.,-1.,0.));
#18126=DIRECTION('center_axis',(-0.866025403784438,0.,0.500000000000001));
#18127=DIRECTION('ref_axis',(-0.500000000000001,0.,-0.866025403784438));
#18128=DIRECTION('',(0.,-1.,0.));
#18129=DIRECTION('center_axis',(0.,0.,1.));
#18130=DIRECTION('ref_axis',(-1.,0.,0.));
#18131=DIRECTION('',(0.,-1.,0.));
#18132=DIRECTION('center_axis',(0.866025403784439,0.,0.5));
#18133=DIRECTION('ref_axis',(-0.5,0.,0.866025403784439));
#18134=DIRECTION('',(0.,-1.,0.));
#18135=DIRECTION('center_axis',(0.866025403784439,0.,-0.5));
#18136=DIRECTION('ref_axis',(0.5,0.,0.866025403784439));
#18137=DIRECTION('',(0.,-1.,0.));
#18138=DIRECTION('center_axis',(0.,0.,-1.));
#18139=DIRECTION('ref_axis',(1.,0.,0.));
#59757=CARTESIAN_POINT('',(0.,0.,0.));
#59758=CARTESIAN_POINT('Origin',(39.2,8.05522481984854,-9.525));
#59759=CARTESIAN_POINT('',(36.958019684865,4.68963520761331,-8.65357747851728));
#59760=CARTESIAN_POINT('',(36.958019684865,4.95526326543997,-8.65357747851728));
#59761=CARTESIAN_POINT('',(36.958019684865,8.05522481984854,-8.65357747851728));
#59762=CARTESIAN_POINT('',(37.7316252379159,5.69997297025342,-11.430184637371));
#59763=CARTESIAN_POINT('Ctrl Pts',(37.7316252379159,5.69997297025341,-11.430184637371));
#59764=CARTESIAN_POINT('Ctrl Pts',(37.7946541587511,5.69324594371103,-11.4787626464628));
#59765=CARTESIAN_POINT('Ctrl Pts',(37.860217046903,5.68651891716864,-11.5243024976679));
#59766=CARTESIAN_POINT('Ctrl Pts',(37.9279877925796,5.67979189062625,-11.5665283217662));
#59767=CARTESIAN_POINT('Ctrl Pts',(37.9956622585872,5.67307442094918,-11.6086941570253));
#59768=CARTESIAN_POINT('Ctrl Pts',(38.0655379578993,5.6663569512721,-11.6475550673986));
#59769=CARTESIAN_POINT('Ctrl Pts',(38.1372568992143,5.65963948159503,-11.6828762814704));
#59770=CARTESIAN_POINT('Ctrl Pts',(38.20889476234,5.6529296060105,-11.718157564946));
#59771=CARTESIAN_POINT('Ctrl Pts',(38.2823713070823,5.64621973042597,-11.7499068967576));
#59772=CARTESIAN_POINT('Ctrl Pts',(38.3573021640367,5.63950985484144,-11.7779343758003));
#59773=CARTESIAN_POINT('Ctrl Pts',(38.4321873033431,5.63280407316085,-11.8059447544057));
#59774=CARTESIAN_POINT('Ctrl Pts',(38.5085245543671,5.62609829148025,-11.830237622806));
#59775=CARTESIAN_POINT('Ctrl Pts',(38.5859088393635,5.61939250979966,-11.8506708689813));
#59776=CARTESIAN_POINT('Ctrl Pts',(38.6632702320777,5.61268871186352,-11.8710980704714));
#59777=CARTESIAN_POINT('Ctrl Pts',(38.7416775892241,5.60598491392738,-11.8876677971188));
#59778=CARTESIAN_POINT('Ctrl Pts',(38.8207113660228,5.59928111599125,-11.9002879986511));
#59779=CARTESIAN_POINT('Ctrl Pts',(38.8997466029625,5.59257719420313,-11.9129084333402));
#59780=CARTESIAN_POINT('Ctrl Pts',(38.9794078178049,5.58587327241501,-11.9215791257643));
#59781=CARTESIAN_POINT('Ctrl Pts',(39.0592674844931,5.57916935062689,-11.9262595243911));
#59782=CARTESIAN_POINT('Ctrl Pts',(39.1392051954725,5.57245887731099,-11.9309444970214));
#59783=CARTESIAN_POINT('Ctrl Pts',(39.2193412750867,5.5657484039951,-11.9316313621234));
#59784=CARTESIAN_POINT('Ctrl Pts',(39.2992460045512,5.5590379306792,-11.9283316822654));
#59785=CARTESIAN_POINT('Ctrl Pts',(39.3791919454358,5.55232399639,-11.9250303005745));
#59786=CARTESIAN_POINT('Ctrl Pts',(39.4589058300058,5.5456100621008,-11.9177383230545));
#59787=CARTESIAN_POINT('Ctrl Pts',(39.537963392915,5.5388961278116,-11.9065191977915));
#59788=CARTESIAN_POINT('Ctrl Pts',(39.6171534627766,5.53217094041848,-11.8952812683553));
#59789=CARTESIAN_POINT('Ctrl Pts',(39.6956845522583,5.52544575302536,-11.880103136358));
#59790=CARTESIAN_POINT('Ctrl Pts',(39.7731433517624,5.51872056563224,-11.8610992364903));
#59791=CARTESIAN_POINT('Ctrl Pts',(39.8253287138061,5.51418968804095,-11.8482959733209));
#59792=CARTESIAN_POINT('Ctrl Pts',(39.8770276482391,5.50965881044965,-11.8337572644404));
#59793=CARTESIAN_POINT('Ctrl Pts',(39.9281186537803,5.50512793285836,-11.8175305167908));
#59794=CARTESIAN_POINT('Ctrl Pts',(40.0043885499032,5.49836412855323,-11.7933068331006));
#59795=CARTESIAN_POINT('Ctrl Pts',(40.0795843205461,5.49160032424809,-11.765229718215));
#59796=CARTESIAN_POINT('Ctrl Pts',(40.1532902141198,5.48483651994295,-11.733413618882));
#59797=CARTESIAN_POINT('Ctrl Pts',(40.2268937455063,5.47808210915803,-11.7016417055069));
#59798=CARTESIAN_POINT('Ctrl Pts',(40.2990110865368,5.47132769837312,-11.6661413046116));
#59799=CARTESIAN_POINT('Ctrl Pts',(40.3692424293285,5.4645732875882,-11.627076374887));
#59800=CARTESIAN_POINT('Ctrl Pts',(40.4393964787615,5.45782631039455,-11.5880544382122));
#59801=CARTESIAN_POINT('Ctrl Pts',(40.5076682512703,5.45107933320089,-11.5454759943738));
#59802=CARTESIAN_POINT('Ctrl Pts',(40.5736800233579,5.44433235600723,-11.4995521360115));
#59803=CARTESIAN_POINT('Ctrl Pts',(40.6396521803153,5.4375894278244,-11.4536558375763));
#59804=CARTESIAN_POINT('Ctrl Pts',(40.7033666490523,5.43084649964157,-11.404418375072));
#59805=CARTESIAN_POINT('Ctrl Pts',(40.764473347711,5.42410357145874,-11.3520949862287));
#59806=CARTESIAN_POINT('Ctrl Pts',(40.8255620129165,5.41736263320962,-11.2997870387593));
#59807=CARTESIAN_POINT('Ctrl Pts',(40.8840440839884,5.4106216949605,-11.2443952757339));
#59808=CARTESIAN_POINT('Ctrl Pts',(40.9396024696636,5.40388075671138,-11.1862152756161));
#59809=CARTESIAN_POINT('Ctrl Pts',(40.995161404406,5.39713975184354,-11.1280347005224));
#59810=CARTESIAN_POINT('Ctrl Pts',(41.0477962765987,5.3903987469757,-11.0670661705574));
#59811=CARTESIAN_POINT('Ctrl Pts',(41.0972277989088,5.38365774210786,-11.0036411408613));
#59812=CARTESIAN_POINT('Ctrl Pts',(41.1467088547655,5.37690998232205,-10.9401525552292));
#59813=CARTESIAN_POINT('Ctrl Pts',(41.1929798626493,5.37016222253623,-10.8742029201246));
#59814=CARTESIAN_POINT('Ctrl Pts',(41.2358030610351,5.36341446275041,-10.8061552759443));
#59815=CARTESIAN_POINT('Ctrl Pts',(41.2786472428939,5.35666339654565,-10.7380742882504));
#59816=CARTESIAN_POINT('Ctrl Pts',(41.3180400216499,5.34991233034089,-10.6678936488724));
#59817=CARTESIAN_POINT('Ctrl Pts',(41.3537893422957,5.34316126413612,-10.5960015935625));
#59818=CARTESIAN_POINT('Ctrl Pts',(41.3896024134546,5.33639815899114,-10.5239813356651));
#59819=CARTESIAN_POINT('Ctrl Pts',(41.4217588576558,5.32963505384615,-10.4502439903742));
#59820=CARTESIAN_POINT('Ctrl Pts',(41.4501146492602,5.32287194870117,-10.3751982178202));
#59821=CARTESIAN_POINT('Ctrl Pts',(41.4757598513906,5.31675534293357,-10.307326227751));
#59822=CARTESIAN_POINT('Ctrl Pts',(41.4982968666121,5.31063873716598,-10.2383844746568));
#59823=CARTESIAN_POINT('Ctrl Pts',(41.5176549374898,5.30452213139838,-10.1686835675463));
#59824=CARTESIAN_POINT('Ctrl Pts',(41.539001577617,5.29777719369539,-10.0918225936393));
#59825=CARTESIAN_POINT('Ctrl Pts',(41.5565610866446,5.29103225599239,-10.0137529010872));
#59826=CARTESIAN_POINT('Ctrl Pts',(41.5702003061424,5.28428731828939,-9.93488224304359));
#59827=CARTESIAN_POINT('Ctrl Pts',(41.5838198456394,5.27755211284268,-9.85612538730496));
#59828=CARTESIAN_POINT('Ctrl Pts',(41.5935302500593,5.27081690739596,-9.77657031808186));
#59829=CARTESIAN_POINT('Ctrl Pts',(41.5992484348811,5.26408170194925,-9.69663884210919));
#59830=CARTESIAN_POINT('Ctrl Pts',(41.6049599526811,5.25735434930243,-9.61680056090113));
#59831=CARTESIAN_POINT('Ctrl Pts',(41.6066884678706,5.25062699665562,-9.53658720908332));
#59832=CARTESIAN_POINT('Ctrl Pts',(41.6044023885841,5.2438996440088,-9.45642815321961));
#59833=CARTESIAN_POINT('Ctrl Pts',(41.6021177687439,5.23717658614268,-9.37632027135907));
#59834=CARTESIAN_POINT('Ctrl Pts',(41.5958236548841,5.23045352827655,-9.29626708279406));
#59835=CARTESIAN_POINT('Ctrl Pts',(41.5855405196536,5.22373047041043,-9.21669921587696));
#59836=CARTESIAN_POINT('Ctrl Pts',(41.5752607609415,5.21700962009372,-9.13715747546372));
#59837=CARTESIAN_POINT('Ctrl Pts',(41.5609946417497,5.210288769777,-9.0581012036375));
#59838=CARTESIAN_POINT('Ctrl Pts',(41.542814470651,5.20356791946028,-8.97995568940831));
#59839=CARTESIAN_POINT('Ctrl Pts',(41.5246346324385,5.19684719220502,-8.90181160605471));
#59840=CARTESIAN_POINT('Ctrl Pts',(41.502540992042,5.19012646494976,-8.82457870228018));
#59841=CARTESIAN_POINT('Ctrl Pts',(41.476656608748,5.18340573769449,-8.74867041133033));
#59842=CARTESIAN_POINT('Ctrl Pts',(41.4507468145623,5.17667841265128,-8.67268760064649));
#59843=CARTESIAN_POINT('Ctrl Pts',(41.4210389948421,5.16995108760807,-8.59803244405444));
#59844=CARTESIAN_POINT('Ctrl Pts',(41.3877054086384,5.16322376256486,-8.52510101039437));
#59845=CARTESIAN_POINT('Ctrl Pts',(41.3543560238464,5.15649324907867,-8.45213501058568));
#59846=CARTESIAN_POINT('Ctrl Pts',(41.3173776648435,5.14976273559249,-8.38089477681323));
#59847=CARTESIAN_POINT('Ctrl Pts',(41.276988728776,5.1430322221063,-8.31175197715497));
#59848=CARTESIAN_POINT('Ctrl Pts',(41.2365273114332,5.13628963015881,-8.24248509504269));
#59849=CARTESIAN_POINT('Ctrl Pts',(41.1926433434954,5.12954703821132,-8.17532356061939));
#59850=CARTESIAN_POINT('Ctrl Pts',(41.1455986367173,5.12280444626383,-8.11061006465549));
#59851=CARTESIAN_POINT('Ctrl Pts',(41.1016696402205,5.11650840748868,-8.05018246010271));
#59852=CARTESIAN_POINT('Ctrl Pts',(41.0549853224597,5.11021236871354,-7.99188928961594));
#59853=CARTESIAN_POINT('Ctrl Pts',(41.0057884671268,5.1039163299384,-7.93598113403525));
#59854=CARTESIAN_POINT('Ctrl Pts',(40.9530101637372,5.09716195016395,-7.87600295906406));
#59855=CARTESIAN_POINT('Ctrl Pts',(40.897142926318,5.0904075703895,-7.81854634138377));
#59856=CARTESIAN_POINT('Ctrl Pts',(40.8384569591934,5.08365319061505,-7.76394584487846));
#59857=CARTESIAN_POINT('Ctrl Pts',(40.7798545226603,5.07690842467788,-7.7094230639157));
#59858=CARTESIAN_POINT('Ctrl Pts',(40.7184416631837,5.07016365874072,-7.65774864502113));
#59859=CARTESIAN_POINT('Ctrl Pts',(40.6545276273748,5.06341889280355,-7.60922278810829));
#59860=CARTESIAN_POINT('Ctrl Pts',(40.5906867420979,5.05668184634788,-7.56075246973574));
#59861=CARTESIAN_POINT('Ctrl Pts',(40.5243507391328,5.04994479989221,-7.51542383191998));
#59862=CARTESIAN_POINT('Ctrl Pts',(40.4558632505349,5.04320775343655,-7.47349800381381));
#59863=CARTESIAN_POINT('Ctrl Pts',(40.3874186421023,5.03647492506029,-7.43159842555964));
#59864=CARTESIAN_POINT('Ctrl Pts',(40.3168256185414,5.02974209668404,-7.39309767046601));
#59865=CARTESIAN_POINT('Ctrl Pts',(40.2444572366038,5.02300926830778,-7.35821389488813));
#59866=CARTESIAN_POINT('Ctrl Pts',(40.1721119045171,5.01627858438585,-7.32334123004399));
#59867=CARTESIAN_POINT('Ctrl Pts',(40.0979927566051,5.00954790046392,-7.29208345902033));
#59868=CARTESIAN_POINT('Ctrl Pts',(40.0224966321684,5.002817216542,-7.26461237074884));
#59869=CARTESIAN_POINT('Ctrl Pts',(39.947001332213,4.99608660612481,-7.23714158248478));
#59870=CARTESIAN_POINT('Ctrl Pts',(39.8701295240859,4.98935599570762,-7.21345755282289));
#59871=CARTESIAN_POINT('Ctrl Pts',(39.7922957941855,4.98262538529043,-7.1936830681801));
#59872=CARTESIAN_POINT('Ctrl Pts',(39.7143856592388,4.9758881678071,-7.17388917202488));
#59873=CARTESIAN_POINT('Ctrl Pts',(39.6355121690381,4.96915095032378,-7.15801260222684));
#59874=CARTESIAN_POINT('Ctrl Pts',(39.5561022097792,4.96241373284045,-7.14612544244335));
#59875=CARTESIAN_POINT('Ctrl Pts',(39.4766544235731,4.95567330608246,-7.13423262020932));
#59876=CARTESIAN_POINT('Ctrl Pts',(39.3966701236061,4.94893287932447,-7.12633304002858));
#59877=CARTESIAN_POINT('Ctrl Pts',(39.3165809532889,4.94219245256649,-7.12244681105074));
#59878=CARTESIAN_POINT('Ctrl Pts',(39.2363492234279,4.93544002777981,-7.11855366454551));
#59879=CARTESIAN_POINT('Ctrl Pts',(39.1560127174399,4.92868760299314,-7.11868814320593));
#59880=CARTESIAN_POINT('Ctrl Pts',(39.0760025199875,4.92193517820646,-7.12281816480298));
#59881=CARTESIAN_POINT('Ctrl Pts',(39.0024407033413,4.91572696163044,-7.12661532942874));
#59882=CARTESIAN_POINT('Ctrl Pts',(38.9291549525295,4.90951874505443,-7.13378931389573));
#59883=CARTESIAN_POINT('Ctrl Pts',(38.8564731110546,4.90331052847841,-7.14427695416467));
#59884=CARTESIAN_POINT('Ctrl Pts',(38.7774012967453,4.89655650383719,-7.15568663679048));
#59885=CARTESIAN_POINT('Ctrl Pts',(38.6987526508042,4.88980247919597,-7.1710609960329));
#59886=CARTESIAN_POINT('Ctrl Pts',(38.6209549970016,4.88304845455474,-7.19035659491593));
#59887=CARTESIAN_POINT('Ctrl Pts',(38.5432678452317,4.87630402317778,-7.20962478676552));
#59888=CARTESIAN_POINT('Ctrl Pts',(38.4664297337037,4.86955959180082,-7.23280304510437));
#59889=CARTESIAN_POINT('Ctrl Pts',(38.3908610433311,4.86281516042386,-7.25979645656273));
#59890=CARTESIAN_POINT('Ctrl Pts',(38.3153784780905,4.85607841563033,-7.28675910381023));
#59891=CARTESIAN_POINT('Ctrl Pts',(38.2411628955007,4.84934167083679,-7.31752810667642));
#59892=CARTESIAN_POINT('Ctrl Pts',(38.1686207484526,4.84260492604325,-7.35195840263526));
#59893=CARTESIAN_POINT('Ctrl Pts',(38.0961238045776,4.8358723791161,-7.38636724405086));
#59894=CARTESIAN_POINT('Ctrl Pts',(38.0252986462831,4.82913983218896,-7.42443265030117));
#59895=CARTESIAN_POINT('Ctrl Pts',(37.9565318165698,4.82240728526182,-7.46596143280491));
#59896=CARTESIAN_POINT('Ctrl Pts',(37.8877866794154,4.81567686212272,-7.50747711501646));
#59897=CARTESIAN_POINT('Ctrl Pts',(37.8210989800708,4.80894643898362,-7.55245376294581));
#59898=CARTESIAN_POINT('Ctrl Pts',(37.7568294249252,4.80221601584453,-7.60065293264489));
#59899=CARTESIAN_POINT('Ctrl Pts',(37.6925603698258,4.79548564507117,-7.64885172733259));
#59900=CARTESIAN_POINT('Ctrl Pts',(37.6307097935878,4.78875527429782,-7.70027271314879));
#59901=CARTESIAN_POINT('Ctrl Pts',(37.5716070605675,4.78202490352446,-7.7546358060539));
#59902=CARTESIAN_POINT('Ctrl Pts',(37.5124459981869,4.77528789044877,-7.80905255069848));
#59903=CARTESIAN_POINT('Ctrl Pts',(37.4560385400727,4.76855087737308,-7.8664168862985));
#59904=CARTESIAN_POINT('Ctrl Pts',(37.4026783093107,4.76181386429738,-7.92641072048584));
#59905=CARTESIAN_POINT('Ctrl Pts',(37.3492925094672,4.7550736229891,-7.98643330243549));
#59906=CARTESIAN_POINT('Ctrl Pts',(37.2989571383783,4.74833338168082,-8.04908752939983));
#59907=CARTESIAN_POINT('Ctrl Pts',(37.2519248885662,4.74159314037254,-8.11402292555401));
#59908=CARTESIAN_POINT('Ctrl Pts',(37.2048086772705,4.73484086645552,-8.17907424370259));
#59909=CARTESIAN_POINT('Ctrl Pts',(37.1610076247398,4.72808859253849,-8.24641447659392));
#59910=CARTESIAN_POINT('Ctrl Pts',(37.1207304078408,4.72133631862147,-8.31566509703801));
#59911=CARTESIAN_POINT('Ctrl Pts',(37.0836846824358,4.71512578808712,-8.37935965357939));
#59912=CARTESIAN_POINT('Ctrl Pts',(37.0496196278822,4.70891525755277,-8.44466980386474));
#59913=CARTESIAN_POINT('Ctrl Pts',(37.0186616191027,4.70270472701843,-8.51128612891783));
#59914=CARTESIAN_POINT('Ctrl Pts',(36.9969454766975,4.69834822055006,-8.55801554267529));
#59915=CARTESIAN_POINT('Ctrl Pts',(36.9767154860701,4.69399171408168,-8.605477254752));
#59916=CARTESIAN_POINT('Ctrl Pts',(36.958019684865,4.68963520761331,-8.65357747851728));
#59917=CARTESIAN_POINT('',(40.6683886799113,5.7,-11.4301739104629));
#59918=CARTESIAN_POINT('Origin',(39.2,5.7,-9.525));
#59919=CARTESIAN_POINT('Ctrl Pts',(40.6683886799113,5.7,-11.4301739104629));
#59920=CARTESIAN_POINT('Ctrl Pts',(40.7334765795775,5.69309458976092,-11.3800082355372));
#59921=CARTESIAN_POINT('Ctrl Pts',(40.7960377610544,5.68618917952184,-11.3264676545935));
#59922=CARTESIAN_POINT('Ctrl Pts',(40.8557196162198,5.67928376928276,-11.2698339453555));
#59923=CARTESIAN_POINT('Ctrl Pts',(40.9153649291418,5.67238258711571,-11.2132349120301));
#59924=CARTESIAN_POINT('Ctrl Pts',(40.9721341083313,5.66548140494865,-11.1535468182329));
#59925=CARTESIAN_POINT('Ctrl Pts',(41.0257091482293,5.6585802227816,-11.0910903711063));
#59926=CARTESIAN_POINT('Ctrl Pts',(41.0792782843711,5.65167980109734,-11.0286408064316));
#59927=CARTESIAN_POINT('Ctrl Pts',(41.1296536902672,5.64477937941309,-10.9634238192556));
#59928=CARTESIAN_POINT('Ctrl Pts',(41.1765561357657,5.63787895772883,-10.895794946944));
#59929=CARTESIAN_POINT('Ctrl Pts',(41.2234574242939,5.63097870626133,-10.8281677428735));
#59930=CARTESIAN_POINT('Ctrl Pts',(41.2668856739803,5.62407845479383,-10.7581291299302));
#59931=CARTESIAN_POINT('Ctrl Pts',(41.3066044364979,5.61717820332633,-10.6860644652763));
#59932=CARTESIAN_POINT('Ctrl Pts',(41.3463319158957,5.61027643749479,-10.6139839849471));
#59933=CARTESIAN_POINT('Ctrl Pts',(41.3823480783771,5.60337467166326,-10.5398769502741));
#59934=CARTESIAN_POINT('Ctrl Pts',(41.4144624914224,5.59647290583172,-10.4641532454735));
#59935=CARTESIAN_POINT('Ctrl Pts',(41.4465917951318,5.58956793982096,-10.3883944294517));
#59936=CARTESIAN_POINT('Ctrl Pts',(41.474815580778,5.5826629738102,-10.3110178534221));
#59937=CARTESIAN_POINT('Ctrl Pts',(41.4989919990329,5.57575800779944,-10.2324522830431));
#59938=CARTESIAN_POINT('Ctrl Pts',(41.5232040150041,5.56884287481443,-10.1537710315545));
#59939=CARTESIAN_POINT('Ctrl Pts',(41.5433566342283,5.56192774182942,-10.0738977070194));
#59940=CARTESIAN_POINT('Ctrl Pts',(41.5593582631339,5.55501260884441,-9.99327505868025));
#59941=CARTESIAN_POINT('Ctrl Pts',(41.5753722850231,5.54809212020899,-9.91258996950013));
#59942=CARTESIAN_POINT('Ctrl Pts',(41.5872288468328,5.54117163157358,-9.83115483134809));
#59943=CARTESIAN_POINT('Ctrl Pts',(41.5948881055281,5.53425114293816,-9.74941904197305));
#59944=CARTESIAN_POINT('Ctrl Pts',(41.6025620627445,5.52731737352031,-9.66752639731028));
#59945=CARTESIAN_POINT('Ctrl Pts',(41.6060226033772,5.52038360410246,-9.58533238461483));
#59946=CARTESIAN_POINT('Ctrl Pts',(41.6052820075671,5.51344983468461,-9.50328805688157));
#59947=CARTESIAN_POINT('Ctrl Pts',(41.6047815801368,5.50876462263641,-9.44784994672573));
#59948=CARTESIAN_POINT('Ctrl Pts',(41.6023640754666,5.50407941058821,-9.39248015451929));
#59949=CARTESIAN_POINT('Ctrl Pts',(41.5980466400686,5.49939419854002,-9.33731607299534));
#59950=CARTESIAN_POINT('Ctrl Pts',(41.5918819269685,5.49270435018622,-9.25854923465905));
#59951=CARTESIAN_POINT('Ctrl Pts',(41.5818184205766,5.48601450183243,-9.17991116903287));
#59952=CARTESIAN_POINT('Ctrl Pts',(41.5678629811776,5.47932465347864,-9.10182409476818));
#59953=CARTESIAN_POINT('Ctrl Pts',(41.5539295969193,5.47264537774405,-9.0238604291156));
#59954=CARTESIAN_POINT('Ctrl Pts',(41.5361165702112,5.46596610200945,-8.94644649046866));
#59955=CARTESIAN_POINT('Ctrl Pts',(41.5144826692387,5.45928682627486,-8.87000158916707));
#59956=CARTESIAN_POINT('Ctrl Pts',(41.4928223421975,5.45259939172508,-8.7934633095043));
#59957=CARTESIAN_POINT('Ctrl Pts',(41.4673318464465,5.44591195717529,-8.71789691467541));
#59958=CARTESIAN_POINT('Ctrl Pts',(41.4381219784085,5.43922452262551,-8.64371516853804));
#59959=CARTESIAN_POINT('Ctrl Pts',(41.4090079777065,5.43255903636162,-8.56977688828589));
#59960=CARTESIAN_POINT('Ctrl Pts',(41.3761991319561,5.42589355009773,-8.49721463561187));
#59961=CARTESIAN_POINT('Ctrl Pts',(41.3398550403091,5.41922806383384,-8.42642212344152));
#59962=CARTESIAN_POINT('Ctrl Pts',(41.3035258815354,5.41256531625065,-8.35565869813428));
#59963=CARTESIAN_POINT('Ctrl Pts',(41.2636645767925,5.40590256866746,-8.28666399368246));
#59964=CARTESIAN_POINT('Ctrl Pts',(41.2204778808029,5.39923982108427,-8.21980956271262));
#59965=CARTESIAN_POINT('Ctrl Pts',(41.1772949733639,5.39257765799027,-8.15296099654437));
#59966=CARTESIAN_POINT('Ctrl Pts',(41.1307875134901,5.38591549489627,-8.08825273057752));
#59967=CARTESIAN_POINT('Ctrl Pts',(41.0812061733673,5.37925333180228,-8.02602825987783));
#59968=CARTESIAN_POINT('Ctrl Pts',(41.031302970757,5.37254792057542,-7.96339985247802));
#59969=CARTESIAN_POINT('Ctrl Pts',(40.9782861245363,5.36584250934857,-7.90328799802043));
#59970=CARTESIAN_POINT('Ctrl Pts',(40.9224518379415,5.35913709812172,-7.84600845434768));
#59971=CARTESIAN_POINT('Ctrl Pts',(40.8669012679019,5.35246575979685,-7.78901997116489));
#59972=CARTESIAN_POINT('Ctrl Pts',(40.8085622135957,5.34579442147197,-7.73483536801589));
#59973=CARTESIAN_POINT('Ctrl Pts',(40.7477613083866,5.3391230831471,-7.68372656113724));
#59974=CARTESIAN_POINT('Ctrl Pts',(40.6864946053458,5.33240063546926,-7.63222620792655));
#59975=CARTESIAN_POINT('Ctrl Pts',(40.6227285632886,5.32567818779141,-7.58384927473834));
#59976=CARTESIAN_POINT('Ctrl Pts',(40.5568272156725,5.31895574011357,-7.53882960166794));
#59977=CARTESIAN_POINT('Ctrl Pts',(40.4909258680564,5.31223329243572,-7.49380992859754));
#59978=CARTESIAN_POINT('Ctrl Pts',(40.422889666234,5.30551084475788,-7.45214771149533));
#59979=CARTESIAN_POINT('Ctrl Pts',(40.3531060649499,5.29878839708003,-7.41402881417679));
#59980=CARTESIAN_POINT('Ctrl Pts',(40.2829266254486,5.29202781720989,-7.37569369247206));
#59981=CARTESIAN_POINT('Ctrl Pts',(40.2107049199298,5.28526723733974,-7.3407918350856));
#59982=CARTESIAN_POINT('Ctrl Pts',(40.1368100741077,5.2785066574696,-7.30954523191055));
#59983=CARTESIAN_POINT('Ctrl Pts',(40.0630205214242,5.27175571078381,-7.278343152178));
#59984=CARTESIAN_POINT('Ctrl Pts',(39.9875629885923,5.26500476409803,-7.25078616139168));
#59985=CARTESIAN_POINT('Ctrl Pts',(39.9108314922945,5.25825381741224,-7.22705058063446));
#59986=CARTESIAN_POINT('Ctrl Pts',(39.8341884282351,5.25151065112115,-7.20334235488317));
#59987=CARTESIAN_POINT('Ctrl Pts',(39.756274761019,5.24476748483006,-7.18344692237463));
#59988=CARTESIAN_POINT('Ctrl Pts',(39.6775034161206,5.23802431853897,-7.16749211411857));
#59989=CARTESIAN_POINT('Ctrl Pts',(39.598781818412,5.23128541082152,-7.15154738194888));
#59990=CARTESIAN_POINT('Ctrl Pts',(39.5192040729623,5.22454650310408,-7.13953842555161));
#59991=CARTESIAN_POINT('Ctrl Pts',(39.4391960348999,5.21780759538663,-7.13154262597218));
#59992=CARTESIAN_POINT('Ctrl Pts',(39.3592140472713,5.21107088184208,-7.12354942980676));
#59993=CARTESIAN_POINT('Ctrl Pts',(39.2788025077089,5.20433416829753,-7.11956684145869));
#59994=CARTESIAN_POINT('Ctrl Pts',(39.1983937510459,5.19759745475299,-7.11962053630528));
#59995=CARTESIAN_POINT('Ctrl Pts',(39.1179865757866,5.19086087369978,-7.11967423009585));
#59996=CARTESIAN_POINT('Ctrl Pts',(39.037582648378,5.18412429264657,-7.1237640476089));
#59997=CARTESIAN_POINT('Ctrl Pts',(38.9576142242073,5.17738771159336,-7.13186354753989));
#59998=CARTESIAN_POINT('Ctrl Pts',(38.8775689910583,5.17064466011245,-7.13997082697036));
#59999=CARTESIAN_POINT('Ctrl Pts',(38.7979605605151,5.16390160863154,-7.15209543533618));
#60000=CARTESIAN_POINT('Ctrl Pts',(38.7192154094158,5.15715855715063,-7.16815908006993));
#60001=CARTESIAN_POINT('Ctrl Pts',(38.640433549353,5.15041236223259,-7.1842302132616));
#60002=CARTESIAN_POINT('Ctrl Pts',(38.5625162217254,5.14366616731455,-7.20424392602886));
#60003=CARTESIAN_POINT('Ctrl Pts',(38.4858766297247,5.13691997239651,-7.22807145160616));
#60004=CARTESIAN_POINT('Ctrl Pts',(38.4091027859999,5.13016195997951,-7.2519407165287));
#60005=CARTESIAN_POINT('Ctrl Pts',(38.3336115882086,5.12340394756252,-7.27963698357706));
#60006=CARTESIAN_POINT('Ctrl Pts',(38.2597978904236,5.11664593514552,-7.31098262483148));
#60007=CARTESIAN_POINT('Ctrl Pts',(38.192576579396,5.11049148863704,-7.33952875059612));
#60008=CARTESIAN_POINT('Ctrl Pts',(38.1267464800312,5.10433704212855,-7.37110078603114));
#60009=CARTESIAN_POINT('Ctrl Pts',(38.0625866948648,5.09818259562006,-7.40553216167326));
#60010=CARTESIAN_POINT('Ctrl Pts',(37.9920899471686,5.09142028396965,-7.44336427091712));
#60011=CARTESIAN_POINT('Ctrl Pts',(37.9233570740887,5.08465797231923,-7.48478487517366));
#60012=CARTESIAN_POINT('Ctrl Pts',(37.856775424105,5.07789566066882,-7.52960513103006));
#60013=CARTESIAN_POINT('Ctrl Pts',(37.7902793533566,5.07114204080451,-7.57436777817255));
#60014=CARTESIAN_POINT('Ctrl Pts',(37.7259293984589,5.0643884209402,-7.62252114485889));
#60015=CARTESIAN_POINT('Ctrl Pts',(37.6640882624756,5.05763480107589,-7.67383061851849));
#60016=CARTESIAN_POINT('Ctrl Pts',(37.6023077439674,5.05088780119645,-7.7250897979735));
#60017=CARTESIAN_POINT('Ctrl Pts',(37.5430315162217,5.04414080131701,-7.77949864537018));
#60018=CARTESIAN_POINT('Ctrl Pts',(37.4865920384997,5.03739380143757,-7.83678019740689));
#60019=CARTESIAN_POINT('Ctrl Pts',(37.4293393750993,5.03054959010443,-7.89488706781365));
#60020=CARTESIAN_POINT('Ctrl Pts',(37.3750062529722,5.0237053787713,-7.95594979801237));
#60021=CARTESIAN_POINT('Ctrl Pts',(37.3239031354747,5.01686116743817,-8.01963841575571));
#60022=CARTESIAN_POINT('Ctrl Pts',(37.2735703380596,5.0101201246336,-8.08236700163276));
#60023=CARTESIAN_POINT('Ctrl Pts',(37.2263711121376,5.00337908182904,-8.14764246220205));
#60024=CARTESIAN_POINT('Ctrl Pts',(37.1825621609754,4.99663803902448,-8.2151154592592));
#60025=CARTESIAN_POINT('Ctrl Pts',(37.1377474963441,4.98974224342706,-8.2841374206294));
#60026=CARTESIAN_POINT('Ctrl Pts',(37.0964810017983,4.98284644782964,-8.35545866392911));
#60027=CARTESIAN_POINT('Ctrl Pts',(37.05898999333,4.97595065223222,-8.42867473086733));
#60028=CARTESIAN_POINT('Ctrl Pts',(37.0214989848616,4.9690548566348,-8.50189079780555));
#60029=CARTESIAN_POINT('Ctrl Pts',(36.9877836755813,4.96215906103738,-8.57700121425903));
#60030=CARTESIAN_POINT('Ctrl Pts',(36.958019684865,4.95526326543996,-8.65357747851728));
#60031=CARTESIAN_POINT('Origin',(39.2,8.05522481984854,-9.525));
#60032=CARTESIAN_POINT('',(36.9580196850403,3.41777315288062,-8.65357747806631));
#60033=CARTESIAN_POINT('',(36.958019684865,3.68510631127449,-8.65357747851727));
#60034=CARTESIAN_POINT('',(36.958019684865,8.05522481984854,-8.65357747851728));
#60035=CARTESIAN_POINT('',(36.7946201341332,4.61461958493973,-9.52419805850888));
#60036=CARTESIAN_POINT('Ctrl Pts',(36.9580196850403,3.41777315288062,-8.65357747806631));
#60037=CARTESIAN_POINT('Ctrl Pts',(36.9593349194975,3.41808797886995,-8.65019366632357));
#60038=CARTESIAN_POINT('Ctrl Pts',(36.9606578277422,3.41840303936403,-8.64681279867953));
#60039=CARTESIAN_POINT('Ctrl Pts',(36.9877525088144,3.42482340968949,-8.57802807636569));
#60040=CARTESIAN_POINT('Ctrl Pts',(37.0163689742119,3.43101227617725,-8.5137885884489));
#60041=CARTESIAN_POINT('Ctrl Pts',(37.0889126010147,3.44545614568467,-8.36842811173175));
#60042=CARTESIAN_POINT('Ctrl Pts',(37.1347754030571,3.45374472789763,-8.28839405107078));
#60043=CARTESIAN_POINT('Ctrl Pts',(37.2429438103379,3.4715372749948,-8.12250437117899));
#60044=CARTESIAN_POINT('Ctrl Pts',(37.3065725150508,3.4810212150294,-8.03772055018812));
#60045=CARTESIAN_POINT('Ctrl Pts',(37.3923506611624,3.49248594432958,-7.93788993403964));
#60046=CARTESIAN_POINT('Ctrl Pts',(37.4094258077318,3.49471002660111,-7.91865049966739));
#60047=CARTESIAN_POINT('Ctrl Pts',(37.4356364992809,3.49803350443211,-7.89005500955978));
#60048=CARTESIAN_POINT('Ctrl Pts',(37.4445443520517,3.49914778652742,-7.88049424535983));
#60049=CARTESIAN_POINT('Ctrl Pts',(37.4610092367117,3.50117898612094,-7.86310879482112));
#60050=CARTESIAN_POINT('Ctrl Pts',(37.4685417756228,3.50209751557398,-7.8552623917427));
#60051=CARTESIAN_POINT('Ctrl Pts',(37.48625346677,3.50423280485122,-7.83706144511141));
#60052=CARTESIAN_POINT('Ctrl Pts',(37.4964735297955,3.50544644338921,-7.82674756194685));
#60053=CARTESIAN_POINT('Ctrl Pts',(37.5307854479325,3.50946283358482,-7.79274212216599));
#60054=CARTESIAN_POINT('Ctrl Pts',(37.5552844415844,3.51223675677904,-7.76946428332693));
#60055=CARTESIAN_POINT('Ctrl Pts',(37.61769324618,3.51909920502861,-7.71262007503551));
#60056=CARTESIAN_POINT('Ctrl Pts',(37.6561886041609,3.52315265981754,-7.67971877114943));
#60057=CARTESIAN_POINT('Ctrl Pts',(37.845657727897,3.54242819202665,-7.52786615872147));
#60058=CARTESIAN_POINT('Ctrl Pts',(38.0094785775956,3.55717542870145,-7.42608412121587));
#60059=CARTESIAN_POINT('Ctrl Pts',(38.2366726010001,3.57725277857447,-7.3201704644883));
#60060=CARTESIAN_POINT('Ctrl Pts',(38.2905559135131,3.5819841610232,-7.29740412773524));
#60061=CARTESIAN_POINT('Ctrl Pts',(38.3672737172541,3.58871506814573,-7.26823749867383));
#60062=CARTESIAN_POINT('Ctrl Pts',(38.389457600915,3.59066066438414,-7.26017528518951));
#60063=CARTESIAN_POINT('Ctrl Pts',(38.4302539410904,3.59423970706849,-7.24602494545069));
#60064=CARTESIAN_POINT('Ctrl Pts',(38.4488291904296,3.59586970297146,-7.2398350908971));
#60065=CARTESIAN_POINT('Ctrl Pts',(38.4868458857951,3.59920779134434,-7.22768033551739));
#60066=CARTESIAN_POINT('Ctrl Pts',(38.5062914963914,3.60091633067944,-7.22173386489734));
#60067=CARTESIAN_POINT('Ctrl Pts',(38.5555106853306,3.60524506442098,-7.20736244497045));
#60068=CARTESIAN_POINT('Ctrl Pts',(38.5853748547347,3.60787545044736,-7.19926440618985));
#60069=CARTESIAN_POINT('Ctrl Pts',(38.7220607272417,3.61993869222232,-7.16501673489835));
#60070=CARTESIAN_POINT('Ctrl Pts',(38.8304252359199,3.62957787645635,-7.14563999734203));
#60071=CARTESIAN_POINT('Ctrl Pts',(39.0273179841395,3.64721128329356,-7.12420879415173));
#60072=CARTESIAN_POINT('Ctrl Pts',(39.1153716064379,3.6551370942823,-7.11949501334781));
#60073=CARTESIAN_POINT('Ctrl Pts',(39.307920757196,3.67243488068461,-7.11977365636811));
#60074=CARTESIAN_POINT('Ctrl Pts',(39.4122516939758,3.68178656166889,-7.12672673736238));
#60075=CARTESIAN_POINT('Ctrl Pts',(39.541230949616,3.6931184791481,-7.14380871599408));
#60076=CARTESIAN_POINT('Ctrl Pts',(39.5665977783173,3.6953356931859,-7.14758192125478));
#60077=CARTESIAN_POINT('Ctrl Pts',(39.6047781775661,3.69865108382608,-7.15388677684076));
#60078=CARTESIAN_POINT('Ctrl Pts',(39.6176383821063,3.69976404308523,-7.15611809152294));
#60079=CARTESIAN_POINT('Ctrl Pts',(39.6411841973916,3.70179413122482,-7.16040113040019));
#60080=CARTESIAN_POINT('Ctrl Pts',(39.6518745538252,3.70271285660973,-7.16242075092119));
#60081=CARTESIAN_POINT('Ctrl Pts',(39.6768226299639,3.70485028175035,-7.16730947590759));
#60082=CARTESIAN_POINT('Ctrl Pts',(39.6910685874196,3.70606583953217,-7.17023544632597));
#60083=CARTESIAN_POINT('Ctrl Pts',(39.7384576614084,3.71009556289681,-7.18041745051984));
#60084=CARTESIAN_POINT('Ctrl Pts',(39.7714756696596,3.7128806429821,-7.18824586407321));
#60085=CARTESIAN_POINT('Ctrl Pts',(39.8536072924712,3.71977782728195,-7.20956409900276));
#60086=CARTESIAN_POINT('Ctrl Pts',(39.9024803365364,3.72385440760067,-7.22392023694661));
#60087=CARTESIAN_POINT('Ctrl Pts',(40.0614028939264,3.73713178791028,-7.27613896083274));
#60088=CARTESIAN_POINT('Ctrl Pts',(40.1691646058674,3.74617540026516,-7.32043357019661));
#60089=CARTESIAN_POINT('Ctrl Pts',(40.3812340085955,3.76479012319636,-7.42617061044486));
#60090=CARTESIAN_POINT('Ctrl Pts',(40.484952411685,3.77434389089163,-7.48801949957636));
#60091=CARTESIAN_POINT('Ctrl Pts',(40.6097556738044,3.78678514089852,-7.57577829045771));
#60092=CARTESIAN_POINT('Ctrl Pts',(40.6355531556078,3.78941133112884,-7.59469865661416));
#60093=CARTESIAN_POINT('Ctrl Pts',(40.6772869714902,3.79375635733544,-7.62660638747983));
#60094=CARTESIAN_POINT('Ctrl Pts',(40.6934483571942,3.79546356438347,-7.63929401707657));
#60095=CARTESIAN_POINT('Ctrl Pts',(40.7247615931006,3.79882143244092,-7.66453176978849));
#60096=CARTESIAN_POINT('Ctrl Pts',(40.7399259470194,3.80047128361934,-7.67706385931336));
#60097=CARTESIAN_POINT('Ctrl Pts',(40.775858112635,3.80443924609642,-7.70750825576055));
#60098=CARTESIAN_POINT('Ctrl Pts',(40.7964761330101,3.80676417554727,-7.72559208224059));
#60099=CARTESIAN_POINT('Ctrl Pts',(40.8703361542095,3.8152743005028,-7.79264259380783));
#60100=CARTESIAN_POINT('Ctrl Pts',(40.9216660134311,3.82154259728327,-7.84364670753645));
#60101=CARTESIAN_POINT('Ctrl Pts',(41.052376799369,3.83850553437088,-7.98579747732892));
#60102=CARTESIAN_POINT('Ctrl Pts',(41.1273159631718,3.84933562970301,-8.08073845455159));
#60103=CARTESIAN_POINT('Ctrl Pts',(41.2603235840797,3.87072742344648,-8.27813632492321));
#60104=CARTESIAN_POINT('Ctrl Pts',(41.3186549492757,3.88125845706078,-8.38005050689291));
#60105=CARTESIAN_POINT('Ctrl Pts',(41.3804161399582,3.89371021654375,-8.5089795001828));
#60106=CARTESIAN_POINT('Ctrl Pts',(41.391137924812,3.89593036170068,-8.53231326458873));
#60107=CARTESIAN_POINT('Ctrl Pts',(41.4067461188607,3.89924921716114,-8.56776699311271));
#60108=CARTESIAN_POINT('Ctrl Pts',(41.4119103814884,3.90036275410026,-8.57976143153011));
#60109=CARTESIAN_POINT('Ctrl Pts',(41.4207733757119,3.90230062786635,-8.60081694606028));
#60110=CARTESIAN_POINT('Ctrl Pts',(41.4245147252638,3.90312737405348,-8.6098590549655));
#60111=CARTESIAN_POINT('Ctrl Pts',(41.4334272387733,3.90511840487546,-8.63177650857913));
#60112=CARTESIAN_POINT('Ctrl Pts',(41.4385423554117,3.90627940840405,-8.6446741577924));
#60113=CARTESIAN_POINT('Ctrl Pts',(41.4543739723483,3.90993423855571,-8.68562366831918));
#60114=CARTESIAN_POINT('Ctrl Pts',(41.4646775074224,3.91240586714179,-8.71383375956975));
#60115=CARTESIAN_POINT('Ctrl Pts',(41.4884031191232,3.91835217647668,-8.78277205112817));
#60116=CARTESIAN_POINT('Ctrl Pts',(41.5012700970713,3.9218027230905,-8.82368150728246));
#60117=CARTESIAN_POINT('Ctrl Pts',(41.5536695550221,3.93703735084219,-9.00729735808516));
#60118=CARTESIAN_POINT('Ctrl Pts',(41.5810704989982,3.94848363400343,-9.15313334783323));
#60119=CARTESIAN_POINT('Ctrl Pts',(41.6046059863442,3.96836056127229,-9.40428041520086));
#60120=CARTESIAN_POINT('Ctrl Pts',(41.607576857524,3.97665301006434,-9.50849911267671));
#60121=CARTESIAN_POINT('Ctrl Pts',(41.6026470661362,3.98770180818317,-9.64381728935149));
#60122=CARTESIAN_POINT('Ctrl Pts',(41.6008997671245,3.99026979060772,-9.67503532655883));
#60123=CARTESIAN_POINT('Ctrl Pts',(41.5970079326382,3.99454404294112,-9.72654897681453));
#60124=CARTESIAN_POINT('Ctrl Pts',(41.5952126438631,3.99623943728665,-9.74686788054385));
#60125=CARTESIAN_POINT('Ctrl Pts',(41.5911699737425,3.99959308236003,-9.78681964440452));
#60126=CARTESIAN_POINT('Ctrl Pts',(41.5889386329375,4.0012507059347,-9.806452532119));
#60127=CARTESIAN_POINT('Ctrl Pts',(41.5829695418447,4.00527023047177,-9.85376955808061));
#60128=CARTESIAN_POINT('Ctrl Pts',(41.5789909846413,4.00763941978551,-9.88141971510631));
#60129=CARTESIAN_POINT('Ctrl Pts',(41.5623135594838,4.01655656271574,-9.98454938083769));
#60130=CARTESIAN_POINT('Ctrl Pts',(41.546497433785,4.02319864062312,-10.0594699090177));
#60131=CARTESIAN_POINT('Ctrl Pts',(41.4920029670353,4.04215576872437,-10.2678774653525));
#60132=CARTESIAN_POINT('Ctrl Pts',(41.4452962297143,4.05466308341572,-10.3989460838626));
#60133=CARTESIAN_POINT('Ctrl Pts',(41.3447781370712,4.07636089683615,-10.6187823799802));
#60134=CARTESIAN_POINT('Ctrl Pts',(41.2960434837016,4.08554313071805,-10.7094999933324));
#60135=CARTESIAN_POINT('Ctrl Pts',(41.2308728583156,4.09622103463023,-10.8141172543996));
#60136=CARTESIAN_POINT('Ctrl Pts',(41.2198828716314,4.0979745801887,-10.8312699306311));
#60137=CARTESIAN_POINT('Ctrl Pts',(41.2020950615439,4.10073709595823,-10.858270939394));
#60138=CARTESIAN_POINT('Ctrl Pts',(41.1954397237062,4.10175457274928,-10.8682112125744));
#60139=CARTESIAN_POINT('Ctrl Pts',(41.1824044956138,4.10371592447883,-10.8873696329386));
#60140=CARTESIAN_POINT('Ctrl Pts',(41.176033911898,4.10466029846762,-10.896593448935));
#60141=CARTESIAN_POINT('Ctrl Pts',(41.1599655937412,4.10700808979212,-10.9195140531975));
#60142=CARTESIAN_POINT('Ctrl Pts',(41.1501882877448,4.10840633807369,-10.9331549150289));
#60143=CARTESIAN_POINT('Ctrl Pts',(41.1105066157445,4.11396665152747,-10.9873108447007));
#60144=CARTESIAN_POINT('Ctrl Pts',(41.0794734953998,4.11806110851368,-11.0269883266445));
#60145=CARTESIAN_POINT('Ctrl Pts',(40.9092298937119,4.13941579932386,-11.231105532998));
#60146=CARTESIAN_POINT('Ctrl Pts',(40.7496410009324,4.15582606096452,-11.3772661891484));
#60147=CARTESIAN_POINT('Ctrl Pts',(40.5212009546674,4.17806399203037,-11.5360234807552));
#60148=CARTESIAN_POINT('Ctrl Pts',(40.4683169050197,4.18313063687343,-11.569788099085));
#60149=CARTESIAN_POINT('Ctrl Pts',(40.3933788918651,4.19024549251481,-11.6136072588675));
#60150=CARTESIAN_POINT('Ctrl Pts',(40.3723990322664,4.19223053260972,-11.6254556376636));
#60151=CARTESIAN_POINT('Ctrl Pts',(40.335518936243,4.19571060183271,-11.6455590071637));
#60152=CARTESIAN_POINT('Ctrl Pts',(40.319697583406,4.19720057279615,-11.653955387708));
#60153=CARTESIAN_POINT('Ctrl Pts',(40.2861509343199,4.20035464571398,-11.6712811955726));
#60154=CARTESIAN_POINT('Ctrl Pts',(40.2684060336639,4.20202003688691,-11.6801694409954));
#60155=CARTESIAN_POINT('Ctrl Pts',(40.2249991967709,4.20608795602905,-11.7012436802878));
#60156=CARTESIAN_POINT('Ctrl Pts',(40.199228098331,4.2084982093548,-11.7131962819359));
#60157=CARTESIAN_POINT('Ctrl Pts',(40.0994795088474,4.21781311161717,-11.7573300481472));
#60158=CARTESIAN_POINT('Ctrl Pts',(40.024120903696,4.22482334666033,-11.786234715184));
#60159=CARTESIAN_POINT('Ctrl Pts',(39.7996781697202,4.24563958834346,-11.8596120323593));
#60160=CARTESIAN_POINT('Ctrl Pts',(39.6475675299655,4.25969457084925,-11.8934809301705));
#60161=CARTESIAN_POINT('Ctrl Pts',(39.4116421127983,4.28096198949319,-11.9224621820517));
#60162=CARTESIAN_POINT('Ctrl Pts',(39.3295390398153,4.28825956304624,-11.9282977830992));
#60163=CARTESIAN_POINT('Ctrl Pts',(39.2275680311205,4.29708849208357,-11.9303028962588));
#60164=CARTESIAN_POINT('Ctrl Pts',(39.2078418519655,4.29878547794429,-11.9304481083016));
#60165=CARTESIAN_POINT('Ctrl Pts',(39.1762899010522,4.30148009113934,-11.9302922100469));
#60166=CARTESIAN_POINT('Ctrl Pts',(39.1644648395972,4.30248555106039,-11.9301465767236));
#60167=CARTESIAN_POINT('Ctrl Pts',(39.141339256127,4.30444261636934,-11.9296911733494));
#60168=CARTESIAN_POINT('Ctrl Pts',(39.1300390608362,4.30539455655823,-11.929388945235));
#60169=CARTESIAN_POINT('Ctrl Pts',(39.1015058901289,4.30778812908807,-11.9284244836011));
#60170=CARTESIAN_POINT('Ctrl Pts',(39.0842766229498,4.30922415578428,-11.9276565487144));
#60171=CARTESIAN_POINT('Ctrl Pts',(39.0125305263457,4.31517106733634,-11.9236851221204));
#60172=CARTESIAN_POINT('Ctrl Pts',(38.9581174383833,4.31960194301343,-11.9188106039989));
#60173=CARTESIAN_POINT('Ctrl Pts',(38.78310588815,4.33373602769284,-11.8971026306808));
#60174=CARTESIAN_POINT('Ctrl Pts',(38.6636021360547,4.34321300819339,-11.8729679713084));
#60175=CARTESIAN_POINT('Ctrl Pts',(38.424298904768,4.36270671317759,-11.805404818618));
#60176=CARTESIAN_POINT('Ctrl Pts',(38.3051017419946,4.37270165331029,-11.7613160017535));
#60177=CARTESIAN_POINT('Ctrl Pts',(38.1554727444249,4.38607733802574,-11.6920853018373));
#60178=CARTESIAN_POINT('Ctrl Pts',(38.1213825474304,4.38918277359544,-11.6753208990794));
#60179=CARTESIAN_POINT('Ctrl Pts',(38.0682080093226,4.39412910690891,-11.647588838696));
#60180=CARTESIAN_POINT('Ctrl Pts',(38.0488516975768,4.39595162432613,-11.6371538788507));
#60181=CARTESIAN_POINT('Ctrl Pts',(38.0129870886127,4.39937163025119,-11.6171798935425));
#60182=CARTESIAN_POINT('Ctrl Pts',(37.9964437406125,4.4009666780374,-11.6077070472827));
#60183=CARTESIAN_POINT('Ctrl Pts',(37.9591958376742,4.40459908865583,-11.5857866311749));
#60184=CARTESIAN_POINT('Ctrl Pts',(37.9385630447664,4.40664052514201,-11.5732219667284));
#60185=CARTESIAN_POINT('Ctrl Pts',(37.8754024078281,4.41298371717641,-11.533442984331));
#60186=CARTESIAN_POINT('Ctrl Pts',(37.8335423996164,4.41732216413543,-11.5052007011732));
#60187=CARTESIAN_POINT('Ctrl Pts',(37.7356636917833,4.42780367380336,-11.4345816941472));
#60188=CARTESIAN_POINT('Ctrl Pts',(37.6805540894529,4.43398492638125,-11.3910293111664));
#60189=CARTESIAN_POINT('Ctrl Pts',(37.5575961585515,4.44843144790128,-11.2847955448982));
#60190=CARTESIAN_POINT('Ctrl Pts',(37.4912932960137,4.45673074992079,-11.2204912259554));
#60191=CARTESIAN_POINT('Ctrl Pts',(37.3571774907485,4.47453880162299,-11.0745416338531));
#60192=CARTESIAN_POINT('Ctrl Pts',(37.2907254102811,4.48402752437495,-10.9918842848524));
#60193=CARTESIAN_POINT('Ctrl Pts',(37.2151744527485,4.49549715542414,-10.8840372471984));
#60194=CARTESIAN_POINT('Ctrl Pts',(37.2007528542799,4.49772156654922,-10.8627315516355));
#60195=CARTESIAN_POINT('Ctrl Pts',(37.1795240863556,4.50104551139799,-10.830258905755));
#60196=CARTESIAN_POINT('Ctrl Pts',(37.1724621803891,4.5021599347227,-10.8192620071867));
#60197=CARTESIAN_POINT('Ctrl Pts',(37.1596905260055,4.50419077934597,-10.7990127066486));
#60198=CARTESIAN_POINT('Ctrl Pts',(37.1539535839346,4.50510881949381,-10.7897787160039));
#60199=CARTESIAN_POINT('Ctrl Pts',(37.1407086773484,4.50724233944137,-10.7681341655149));
#60200=CARTESIAN_POINT('Ctrl Pts',(37.1332500609947,4.50845470668049,-10.7556941242143));
#60201=CARTESIAN_POINT('Ctrl Pts',(37.1088162703426,4.51246590975881,-10.7140929345523));
#60202=CARTESIAN_POINT('Ctrl Pts',(37.0923411596199,4.51523597027895,-10.6846404417925));
#60203=CARTESIAN_POINT('Ctrl Pts',(37.0223520517019,4.52734878408397,-10.5530984496911));
#60204=CARTESIAN_POINT('Ctrl Pts',(36.9755904287197,4.53639380378068,-10.4475755256196));
#60205=CARTESIAN_POINT('Ctrl Pts',(36.9096088648786,4.55166900248483,-10.2641268704389));
#60206=CARTESIAN_POINT('Ctrl Pts',(36.8863869460265,4.55789471082588,-10.1878681683283));
#60207=CARTESIAN_POINT('Ctrl Pts',(36.8434934239081,4.57180552029606,-10.0169818395727));
#60208=CARTESIAN_POINT('Ctrl Pts',(36.8256537930671,4.57950937869751,-9.92204613593157));
#60209=CARTESIAN_POINT('Ctrl Pts',(36.8097500044078,4.58987628827759,-9.7960826735058));
#60210=CARTESIAN_POINT('Ctrl Pts',(36.8065089090259,4.59237964481638,-9.76579262024283));
#60211=CARTESIAN_POINT('Ctrl Pts',(36.802251019455,4.59640768509294,-9.71731297228475));
#60212=CARTESIAN_POINT('Ctrl Pts',(36.800864061711,4.59792085650306,-9.6991584467843));
#60213=CARTESIAN_POINT('Ctrl Pts',(36.7984930904349,4.60097234035345,-9.66267491704818));
#60214=CARTESIAN_POINT('Ctrl Pts',(36.7975125202716,4.60251065399688,-9.64434692865343));
#60215=CARTESIAN_POINT('Ctrl Pts',(36.7960299714833,4.60548238504996,-9.60907372929461));
#60216=CARTESIAN_POINT('Ctrl Pts',(36.7954972013234,4.60691475386162,-9.59213083839908));
#60217=CARTESIAN_POINT('Ctrl Pts',(36.7947878054176,4.60979919286109,-9.55813616266211));
#60218=CARTESIAN_POINT('Ctrl Pts',(36.7946133512244,4.6112512407497,-9.54108538153903));
#60219=CARTESIAN_POINT('Ctrl Pts',(36.7946201936848,4.61270879799127,-9.52403471701899));
#60220=CARTESIAN_POINT('Ctrl Pts',(36.958019684865,4.68963520761331,-8.65357747851728));
#60221=CARTESIAN_POINT('Ctrl Pts',(36.9266910895544,4.68233500011651,-8.73417912956007));
#60222=CARTESIAN_POINT('Ctrl Pts',(36.8996729894311,4.6750347926197,-8.81657491459788));
#60223=CARTESIAN_POINT('Ctrl Pts',(36.8771553691407,4.6677345851229,-8.90030346144062));
#60224=CARTESIAN_POINT('Ctrl Pts',(36.8546928748826,4.66045224947351,-8.98382703002562));
#60225=CARTESIAN_POINT('Ctrl Pts',(36.8367090122413,4.65316991382412,-9.06867653828263));
#60226=CARTESIAN_POINT('Ctrl Pts',(36.8233451126604,4.64588757817474,-9.15437284113991));
#60227=CARTESIAN_POINT('Ctrl Pts',(36.8100296243597,4.63863162308812,-9.23975870558766));
#60228=CARTESIAN_POINT('Ctrl Pts',(36.8013008096218,4.6313756680015,-9.32598491874802));
#60229=CARTESIAN_POINT('Ctrl Pts',(36.7972493975383,4.62411971291489,-9.41256118655141));
#60230=CARTESIAN_POINT('Ctrl Pts',(36.7955102029823,4.62100486867674,-9.44972674032186));
#60231=CARTESIAN_POINT('Ctrl Pts',(36.7946323438184,4.6178900244386,-9.48695662627579));
#60232=CARTESIAN_POINT('Ctrl Pts',(36.7946201292839,4.61477518020045,-9.5242113593961));
#60233=CARTESIAN_POINT('',(36.7946203555469,4.88022481979722,-9.52369215796182));
#60234=CARTESIAN_POINT('Ctrl Pts',(36.958019684865,4.95526326543996,-8.65357747851728));
#60235=CARTESIAN_POINT('Ctrl Pts',(36.9288792425646,4.94851193509457,-8.72854948853697));
#60236=CARTESIAN_POINT('Ctrl Pts',(36.9035262455792,4.94176060474919,-8.80492605243814));
#60237=CARTESIAN_POINT('Ctrl Pts',(36.882075044055,4.93500927440379,-8.88228945628127));
#60238=CARTESIAN_POINT('Ctrl Pts',(36.8605859979768,4.92824603325307,-8.95978934588294));
#60239=CARTESIAN_POINT('Ctrl Pts',(36.8430126020127,4.92148279210234,-9.03827909962506));
#60240=CARTESIAN_POINT('Ctrl Pts',(36.8294181568492,4.91471955095162,-9.11733019571729));
#60241=CARTESIAN_POINT('Ctrl Pts',(36.8179322306018,4.90900529868777,-9.1841203477668));
#60242=CARTESIAN_POINT('Ctrl Pts',(36.8092858028889,4.90329104642392,-9.25131092184784));
#60243=CARTESIAN_POINT('Ctrl Pts',(36.8034880601261,4.89757679416008,-9.31864238215755));
#60244=CARTESIAN_POINT('Ctrl Pts',(36.7976195592362,4.8917928027229,-9.38679558434429));
#60245=CARTESIAN_POINT('Ctrl Pts',(36.7946575928612,4.88600881128573,-9.45520541903671));
#60246=CARTESIAN_POINT('Ctrl Pts',(36.7946203555473,4.88022481984855,-9.52369215735399));
#60247=CARTESIAN_POINT('Ctrl Pts',(36.7946203555469,4.88022481979722,-9.52369215796182));
#60248=CARTESIAN_POINT('Ctrl Pts',(36.7945774403228,4.87355888775427,-9.6026217256193));
#60249=CARTESIAN_POINT('Ctrl Pts',(36.7984237148322,4.86689295571132,-9.68170890384972));
#60250=CARTESIAN_POINT('Ctrl Pts',(36.8061793828676,4.86022702366837,-9.76053300701142));
#60251=CARTESIAN_POINT('Ctrl Pts',(36.8140937523611,4.85342468904469,-9.84097005957397));
#60252=CARTESIAN_POINT('Ctrl Pts',(36.8260793720773,4.84662235442101,-9.92113265213544));
#60253=CARTESIAN_POINT('Ctrl Pts',(36.8421016826417,4.83982001979733,-10.0005717289734));
#60254=CARTESIAN_POINT('Ctrl Pts',(36.8577660106002,4.83316966808927,-10.0782359177502));
#60255=CARTESIAN_POINT('Ctrl Pts',(36.8772884269659,4.82651931638121,-10.1552080876193));
#60256=CARTESIAN_POINT('Ctrl Pts',(36.9005843338745,4.81986896467315,-10.2310740320792));
#60257=CARTESIAN_POINT('Ctrl Pts',(36.9238685954304,4.81322193739851,-10.3069020520365));
#60258=CARTESIAN_POINT('Ctrl Pts',(36.9509224647324,4.80657491012386,-10.3816244864583));
#60259=CARTESIAN_POINT('Ctrl Pts',(36.9816109228423,4.79992788284922,-10.4548402264623));
#60260=CARTESIAN_POINT('Ctrl Pts',(37.0122940669605,4.79328200656913,-10.5280432884805));
#60261=CARTESIAN_POINT('Ctrl Pts',(37.046610364529,4.78663613028903,-10.599739732533));
#60262=CARTESIAN_POINT('Ctrl Pts',(37.084376480927,4.77999025400894,-10.6695479762532));
#60263=CARTESIAN_POINT('Ctrl Pts',(37.1236905226191,4.77307198223321,-10.7422174605904));
#60264=CARTESIAN_POINT('Ctrl Pts',(37.1667430396016,4.76615371045747,-10.8128401164677));
#60265=CARTESIAN_POINT('Ctrl Pts',(37.2132751644996,4.75923543868173,-10.8810152552262));
#60266=CARTESIAN_POINT('Ctrl Pts',(37.2580307062566,4.75258130453197,-10.9465874868011));
#60267=CARTESIAN_POINT('Ctrl Pts',(37.3060046286374,4.74592717038221,-11.0098953432796));
#60268=CARTESIAN_POINT('Ctrl Pts',(37.3569244840516,4.73927303623246,-11.0706149542857));
#60269=CARTESIAN_POINT('Ctrl Pts',(37.4078784733848,4.7326144415108,-11.1313752684374));
#60270=CARTESIAN_POINT('Ctrl Pts',(37.4617819963938,4.72595584678915,-11.1895435375494));
#60271=CARTESIAN_POINT('Ctrl Pts',(37.5183256588246,4.71929725206749,-11.2448326530894));
#60272=CARTESIAN_POINT('Ctrl Pts',(37.5749564181489,4.71262840079559,-11.3002069330845));
#60273=CARTESIAN_POINT('Ctrl Pts',(37.6342350654922,4.70595954952369,-11.3526929041604));
#60274=CARTESIAN_POINT('Ctrl Pts',(37.6958198457973,4.69929069825179,-11.4020442211367));
#60275=CARTESIAN_POINT('Ctrl Pts',(37.7029604337311,4.69851746306789,-11.4077663722392));
#60276=CARTESIAN_POINT('Ctrl Pts',(37.7101319945935,4.69774422788399,-11.4134464308331));
#60277=CARTESIAN_POINT('Ctrl Pts',(37.7173339726834,4.69697099270009,-11.4190840519473));
#60278=CARTESIAN_POINT('Ctrl Pts',(37.7802449250829,4.69021660366409,-11.4683299825981));
#60279=CARTESIAN_POINT('Ctrl Pts',(37.8457282525118,4.68346221462809,-11.514529153661));
#60280=CARTESIAN_POINT('Ctrl Pts',(37.9134568159231,4.6767078255921,-11.5574024158383));
#60281=CARTESIAN_POINT('Ctrl Pts',(37.9810889790601,4.66996305029841,-11.6002146551026));
#60282=CARTESIAN_POINT('Ctrl Pts',(38.0509596405553,4.66321827500472,-11.6397101401676));
#60283=CARTESIAN_POINT('Ctrl Pts',(38.1227096068288,4.65647349971103,-11.6756506813477));
#60284=CARTESIAN_POINT('Ctrl Pts',(38.194377455395,4.64973644380054,-11.7115500886429));
#60285=CARTESIAN_POINT('Ctrl Pts',(38.2679199194095,4.64299938789005,-11.7439024304701));
#60286=CARTESIAN_POINT('Ctrl Pts',(38.3429511939564,4.63626233197956,-11.7725142465531));
#60287=CARTESIAN_POINT('Ctrl Pts',(38.4179354919404,4.62952949409326,-11.8011081489757));
#60288=CARTESIAN_POINT('Ctrl Pts',(38.4944063157194,4.62279665620695,-11.8259660089512));
#60289=CARTESIAN_POINT('Ctrl Pts',(38.5719568429212,4.61606381832065,-11.8469420184937));
#60290=CARTESIAN_POINT('Ctrl Pts',(38.6494826702371,4.60933312484694,-11.8679113471655));
#60291=CARTESIAN_POINT('Ctrl Pts',(38.7280870684362,4.60260243137322,-11.8850011592218));
#60292=CARTESIAN_POINT('Ctrl Pts',(38.8073483679933,4.59587173789951,-11.8981155977496));
#60293=CARTESIAN_POINT('Ctrl Pts',(38.886608802285,4.58914111790222,-11.9112298931121));
#60294=CARTESIAN_POINT('Ctrl Pts',(38.9665256636284,4.58241049790493,-11.9203688265133));
#60295=CARTESIAN_POINT('Ctrl Pts',(39.0466688525193,4.57567987790765,-11.9254879719783));
#60296=CARTESIAN_POINT('Ctrl Pts',(39.1268907131434,4.56894265086679,-11.9306121425994));
#60297=CARTESIAN_POINT('Ctrl Pts',(39.2073388789196,4.56220542382593,-11.9317086130594));
#60298=CARTESIAN_POINT('Ctrl Pts',(39.2875804874595,4.55546819678507,-11.9287850574909));
#60299=CARTESIAN_POINT('Ctrl Pts',(39.3678603190795,4.54872776046696,-11.925860109287));
#60300=CARTESIAN_POINT('Ctrl Pts',(39.4479329324827,4.54198732414885,-11.9189113601794));
#60301=CARTESIAN_POINT('Ctrl Pts',(39.5273703501804,4.53524688783074,-11.9079984469619));
#60302=CARTESIAN_POINT('Ctrl Pts',(39.6069491658313,4.52849445359116,-11.8970661088482));
#60303=CARTESIAN_POINT('Ctrl Pts',(39.6858900674182,4.52174201935158,-11.8821555936922));
#60304=CARTESIAN_POINT('Ctrl Pts',(39.7637752274882,4.514989585112,-11.8633777362245));
#60305=CARTESIAN_POINT('Ctrl Pts',(39.8353821890891,4.50878145382138,-11.8461135318828));
#60306=CARTESIAN_POINT('Ctrl Pts',(39.9060966389583,4.50257332253075,-11.8255810079071));
#60307=CARTESIAN_POINT('Ctrl Pts',(39.9756079607792,4.49636519124012,-11.8019025529381));
#60308=CARTESIAN_POINT('Ctrl Pts',(40.0512315734989,4.48961116464219,-11.7761419967945));
#60309=CARTESIAN_POINT('Ctrl Pts',(40.1257099193966,4.48285713804425,-11.7465622630599));
#60310=CARTESIAN_POINT('Ctrl Pts',(40.1986304658414,4.47610311144631,-11.7132847477176));
#60311=CARTESIAN_POINT('Ctrl Pts',(40.2714474382258,4.46935867805623,-11.6800544987158));
#60312=CARTESIAN_POINT('Ctrl Pts',(40.3427105850688,4.46261424466615,-11.6431370914683));
#60313=CARTESIAN_POINT('Ctrl Pts',(40.4120241589146,4.45586981127607,-11.602703150743));
#60314=CARTESIAN_POINT('Ctrl Pts',(40.4812587373487,4.44913306439332,-11.56231529184));
#60315=CARTESIAN_POINT('Ctrl Pts',(40.548547757972,4.44239631751056,-11.5184190981792));
#60316=CARTESIAN_POINT('Ctrl Pts',(40.6135183888386,4.43565957062781,-11.4712319257517));
#60317=CARTESIAN_POINT('Ctrl Pts',(40.6784485350197,4.42892702156605,-11.4240741567301));
#60318=CARTESIAN_POINT('Ctrl Pts',(40.7410627830016,4.4221944725043,-11.3736297529507));
#60319=CARTESIAN_POINT('Ctrl Pts',(40.8010167239755,4.41546192344254,-11.3201597126581));
#60320=CARTESIAN_POINT('Ctrl Pts',(40.8609517528089,4.40873149812631,-11.2667065391953));
#60321=CARTESIAN_POINT('Ctrl Pts',(40.9182277936001,4.40200107281007,-11.2102299347198));
#60322=CARTESIAN_POINT('Ctrl Pts',(40.9725341581777,4.39527064749383,-11.1510306277845));
#60323=CARTESIAN_POINT('Ctrl Pts',(41.0268401005479,4.38854027450362,-11.0918317810972));
#60324=CARTESIAN_POINT('Ctrl Pts',(41.0781760985413,4.3818099015134,-11.0299106184793));
#60325=CARTESIAN_POINT('Ctrl Pts',(41.1262699310444,4.37507952852318,-10.9656030324674));
#60326=CARTESIAN_POINT('Ctrl Pts',(41.1744112283861,4.36834251318297,-10.9012319799145));
#60327=CARTESIAN_POINT('Ctrl Pts',(41.2193036886749,4.36160549784275,-10.8344701734186));
#60328=CARTESIAN_POINT('Ctrl Pts',(41.2607172139349,4.35486848250254,-10.7656842904593));
#60329=CARTESIAN_POINT('Ctrl Pts',(41.302150583846,4.3481282389001,-10.6968654464845));
#60330=CARTESIAN_POINT('Ctrl Pts',(41.3401014770831,4.34138799529767,-10.6260210051411));
#60331=CARTESIAN_POINT('Ctrl Pts',(41.3743859848242,4.33464775169523,-10.5535419453772));
#60332=CARTESIAN_POINT('Ctrl Pts',(41.4087316970137,4.32789547545999,-10.4809334965343));
#60333=CARTESIAN_POINT('Ctrl Pts',(41.4393977667856,4.32114319922476,-10.4066850302307));
#60334=CARTESIAN_POINT('Ctrl Pts',(41.4662487100064,4.31439092298952,-10.3312070012065));
#60335=CARTESIAN_POINT('Ctrl Pts',(41.490945282584,4.30818041191972,-10.2617849102773));
#60336=CARTESIAN_POINT('Ctrl Pts',(41.5124148755175,4.30196990084993,-10.1913231096163));
#60337=CARTESIAN_POINT('Ctrl Pts',(41.5305901900215,4.29575938978013,-10.1201489818321));
#60338=CARTESIAN_POINT('Ctrl Pts',(41.5503494618059,4.28900763997568,-10.0427721125296));
#60339=CARTESIAN_POINT('Ctrl Pts',(41.5662878541097,4.28225589017123,-9.96426632387336));
#60340=CARTESIAN_POINT('Ctrl Pts',(41.5782812986408,4.27550414036678,-9.88504306539031));
#60341=CARTESIAN_POINT('Ctrl Pts',(41.5902576260479,4.26876202670458,-9.80593287486901));
#60342=CARTESIAN_POINT('Ctrl Pts',(41.5983001183935,4.26201991304238,-9.72610770565665));
#60343=CARTESIAN_POINT('Ctrl Pts',(41.6023350939562,4.25527779938018,-9.64599190364012));
#60344=CARTESIAN_POINT('Ctrl Pts',(41.6063654371608,4.24854342600903,-9.56596807865868));
#60345=CARTESIAN_POINT('Ctrl Pts',(41.6063973838752,4.24180905263788,-9.48565474755449));
#60346=CARTESIAN_POINT('Ctrl Pts',(41.6024089049995,4.23507467926672,-9.40548264737234));
#60347=CARTESIAN_POINT('Ctrl Pts',(41.5984229310417,4.22834453534059,-9.32536089834706));
#60348=CARTESIAN_POINT('Ctrl Pts',(41.5904215668024,4.22161439141446,-9.24538066888293));
#60349=CARTESIAN_POINT('Ctrl Pts',(41.5784348642965,4.21488424748833,-9.16597278557365));
#60350=CARTESIAN_POINT('Ctrl Pts',(41.5664519945955,4.20815625555756,-9.08659029331076));
#60351=CARTESIAN_POINT('Ctrl Pts',(41.5504863869424,4.20142826362679,-9.007780244697));
#60352=CARTESIAN_POINT('Ctrl Pts',(41.530619798486,4.19470027169603,-8.92996697629017));
#60353=CARTESIAN_POINT('Ctrl Pts',(41.5107534380768,4.18797235699541,-8.85215460109645));
#60354=CARTESIAN_POINT('Ctrl Pts',(41.4869863026282,4.18124444229479,-8.77533943502138));
#60355=CARTESIAN_POINT('Ctrl Pts',(41.459450627858,4.17451652759418,-8.69993284838608));
#60356=CARTESIAN_POINT('Ctrl Pts',(41.4318878582798,4.16778199269782,-8.62445206248017));
#60357=CARTESIAN_POINT('Ctrl Pts',(41.4005493023171,4.16104745780147,-8.5503830639371));
#60358=CARTESIAN_POINT('Ctrl Pts',(41.3656160067488,4.15431292290512,-8.47811879579702));
#60359=CARTESIAN_POINT('Ctrl Pts',(41.3306660486845,4.14757517576788,-8.40582005902033));
#60360=CARTESIAN_POINT('Ctrl Pts',(41.2921181591336,4.14083742863065,-8.33532817748099));
#60361=CARTESIAN_POINT('Ctrl Pts',(41.2501989899998,4.13409968149342,-8.26701071316009));
#60362=CARTESIAN_POINT('Ctrl Pts',(41.2082049477827,4.12734989986425,-8.19857122497034));
#60363=CARTESIAN_POINT('Ctrl Pts',(41.1628278580619,4.12060011823509,-8.13231430037839));
#60364=CARTESIAN_POINT('Ctrl Pts',(41.1143371591158,4.11385033660593,-8.06857760741311));
#60365=CARTESIAN_POINT('Ctrl Pts',(41.0695644320259,4.10761808717733,-8.00972785639345));
#60366=CARTESIAN_POINT('Ctrl Pts',(41.0221379048071,4.10138583774874,-7.95302653405436));
#60367=CARTESIAN_POINT('Ctrl Pts',(40.9722975880818,4.09515358832014,-7.8987115250733));
#60368=CARTESIAN_POINT('Ctrl Pts',(40.9182918137351,4.08840047199931,-7.83985708129362));
#60369=CARTESIAN_POINT('Ctrl Pts',(40.8612512106479,4.08164735567848,-7.78358671238853));
#60370=CARTESIAN_POINT('Ctrl Pts',(40.8014527295569,4.07489423935764,-7.73022923486182));
#60371=CARTESIAN_POINT('Ctrl Pts',(40.7417394114184,4.0681507405942,-7.67694774723045));
#60372=CARTESIAN_POINT('Ctrl Pts',(40.679276361022,4.06140724183076,-7.62657121976668));
#60373=CARTESIAN_POINT('Ctrl Pts',(40.6143788556305,4.05466374306732,-7.57939330872213));
#60374=CARTESIAN_POINT('Ctrl Pts',(40.5495556344738,4.04792796317753,-7.53226939936832));
#60375=CARTESIAN_POINT('Ctrl Pts',(40.4823038716433,4.04119218328774,-7.48833710282283));
#60376=CARTESIAN_POINT('Ctrl Pts',(40.4129724165713,4.03445640339796,-7.44785030365236));
#60377=CARTESIAN_POINT('Ctrl Pts',(40.343684367905,4.02772484058387,-7.40738885208816));
#60378=CARTESIAN_POINT('Ctrl Pts',(40.2723196132366,4.02099327776977,-7.37036885037852));
#60379=CARTESIAN_POINT('Ctrl Pts',(40.1992555315112,4.01426171495568,-7.33700061079891));
#60380=CARTESIAN_POINT('Ctrl Pts',(40.1262146949032,4.00753229376801,-7.30364298722417));
#60381=CARTESIAN_POINT('Ctrl Pts',(40.0514760287572,4.00080287258034,-7.27393501205814));
#60382=CARTESIAN_POINT('Ctrl Pts',(39.9754397279329,3.99407345139267,-7.24804014687492));
#60383=CARTESIAN_POINT('Ctrl Pts',(39.8994042050589,3.98734409905574,-7.22214554662989));
#60384=CARTESIAN_POINT('Ctrl Pts',(39.8220715157349,3.98061474671881,-7.2000641278065));
#60385=CARTESIAN_POINT('Ctrl Pts',(39.743858579342,3.97388539438188,-7.18190999104258));
#60386=CARTESIAN_POINT('Ctrl Pts',(39.6655686620604,3.9671494186966,-7.16373798611456));
#60387=CARTESIAN_POINT('Ctrl Pts',(39.5863972223019,3.96041344301131,-7.14950109040008));
#60388=CARTESIAN_POINT('Ctrl Pts',(39.5067724215681,3.95367746732602,-7.13926245664674));
#60389=CARTESIAN_POINT('Ctrl Pts',(39.4271096022657,3.9469382754047,-7.12901893423816));
#60390=CARTESIAN_POINT('Ctrl Pts',(39.3469934562053,3.94019908348338,-7.12277751346746));
#60391=CARTESIAN_POINT('Ctrl Pts',(39.2668558148351,3.93345989156206,-7.12054928425997));
#60392=CARTESIAN_POINT('Ctrl Pts',(39.1865751879476,3.92670867524339,-7.11831707933645));
#60393=CARTESIAN_POINT('Ctrl Pts',(39.1062734564255,3.91995745892471,-7.12011236363538));
#60394=CARTESIAN_POINT('Ctrl Pts',(39.0263808027279,3.91320624260604,-7.12589405845874));
#60395=CARTESIAN_POINT('Ctrl Pts',(38.9527805568328,3.90698675735742,-7.13122038248223));
#60396=CARTESIAN_POINT('Ctrl Pts',(38.8795277139355,3.9007672721088,-7.13992926607577));
#60397=CARTESIAN_POINT('Ctrl Pts',(38.8069505596118,3.89454778686017,-7.15195025719846));
#60398=CARTESIAN_POINT('Ctrl Pts',(38.728148265386,3.8877948394477,-7.16500232142117));
#60399=CARTESIAN_POINT('Ctrl Pts',(38.6498508697298,3.88104189203523,-7.18200801276839));
#60400=CARTESIAN_POINT('Ctrl Pts',(38.5724850870386,3.87428894462276,-7.20291516554391));
#60401=CARTESIAN_POINT('Ctrl Pts',(38.4952294795526,3.86754561396,-7.22379254482306));
#60402=CARTESIAN_POINT('Ctrl Pts',(38.4189032966122,3.86080228329723,-7.24856023024329));
#60403=CARTESIAN_POINT('Ctrl Pts',(38.3439247610938,3.85405895263446,-7.27711474275673));
#60404=CARTESIAN_POINT('Ctrl Pts',(38.2690320282456,3.84732333879055,-7.30563657853939));
#60405=CARTESIAN_POINT('Ctrl Pts',(38.1954843114477,3.84058772494664,-7.337936463867));
#60406=CARTESIAN_POINT('Ctrl Pts',(38.1236848815208,3.83385211110273,-7.37386106675253));
#60407=CARTESIAN_POINT('Ctrl Pts',(38.0519303900041,3.82712071299951,-7.40976318485587));
#60408=CARTESIAN_POINT('Ctrl Pts',(37.9819224291752,3.82038931489629,-7.44928530894816));
#60409=CARTESIAN_POINT('Ctrl Pts',(37.9140433782879,3.81365791679308,-7.49222639935606));
#60410=CARTESIAN_POINT('Ctrl Pts',(37.8461859075688,3.80692865874192,-7.53515383789437));
#60411=CARTESIAN_POINT('Ctrl Pts',(37.7804563964344,3.80019940069076,-7.58149783497121));
#60412=CARTESIAN_POINT('Ctrl Pts',(37.7172104638034,3.79347014263961,-7.63101263580089));
#60413=CARTESIAN_POINT('Ctrl Pts',(37.6539651612174,3.78674095162415,-7.68052694337272));
#60414=CARTESIAN_POINT('Ctrl Pts',(37.5932037542561,3.7800117606087,-7.73321170334964));
#60415=CARTESIAN_POINT('Ctrl Pts',(37.5352496695307,3.77328256959324,-7.78878017474674));
#60416=CARTESIAN_POINT('Ctrl Pts',(37.477238507653,3.76654675120954,-7.84440337378078));
#60417=CARTESIAN_POINT('Ctrl Pts',(37.4220405283669,3.75981093282584,-7.90291563403494));
#60418=CARTESIAN_POINT('Ctrl Pts',(37.3699426403205,3.75307511444214,-7.96399295175109));
#60419=CARTESIAN_POINT('Ctrl Pts',(37.3178198613456,3.74633607787091,-8.02509945051856));
#60420=CARTESIAN_POINT('Ctrl Pts',(37.2688004093012,3.73959704129968,-8.08877307834769));
#60421=CARTESIAN_POINT('Ctrl Pts',(37.2231296017101,3.73285800472846,-8.15465830072746));
#60422=CARTESIAN_POINT('Ctrl Pts',(37.1773772691902,3.72610693860256,-8.22066113188945));
#60423=CARTESIAN_POINT('Ctrl Pts',(37.1349857720421,3.71935587247666,-8.28888304904211));
#60424=CARTESIAN_POINT('Ctrl Pts',(37.0961558408247,3.71260480635077,-8.35894138298974));
#60425=CARTESIAN_POINT('Ctrl Pts',(37.0603750204169,3.70638386603391,-8.42349840347501));
#60426=CARTESIAN_POINT('Ctrl Pts',(37.0276179788031,3.70016292571704,-8.4896142202192));
#60427=CARTESIAN_POINT('Ctrl Pts',(36.9980052420606,3.69394198540018,-8.55697519122324));
#60428=CARTESIAN_POINT('Ctrl Pts',(36.9839854702094,3.69099676069162,-8.5888663822794));
#60429=CARTESIAN_POINT('Ctrl Pts',(36.9706522083476,3.68805153598306,-8.62107674749401));
#60430=CARTESIAN_POINT('Ctrl Pts',(36.958019684865,3.68510631127449,-8.65357747851728));
#60431=CARTESIAN_POINT('Origin',(39.2,8.05522481984854,-9.525));
#60432=CARTESIAN_POINT('',(36.9580197803105,2.14933799730903,-8.65357723295689));
#60433=CARTESIAN_POINT('',(36.960707778965,2.41503531351511,-8.65459504792143));
#60434=CARTESIAN_POINT('',(36.958019684865,8.05522481984854,-8.65357747851728));
#60435=CARTESIAN_POINT('Ctrl Pts',(36.9580197803105,2.14933799730903,-8.65357723295689));
#60436=CARTESIAN_POINT('Ctrl Pts',(36.9800579747574,2.15411338859981,-8.59687777788607));
#60437=CARTESIAN_POINT('Ctrl Pts',(37.004249355822,2.15890857144129,-8.54100834907343));
#60438=CARTESIAN_POINT('Ctrl Pts',(37.0624888151197,2.16964011257482,-8.41939256638918));
#60439=CARTESIAN_POINT('Ctrl Pts',(37.0974851644807,2.17559155144584,-8.35420912979925));
#60440=CARTESIAN_POINT('Ctrl Pts',(37.1496303646409,2.18391232036595,-8.26698420663039));
#60441=CARTESIAN_POINT('Ctrl Pts',(37.164244466139,2.18619260383398,-8.24347018915741));
#60442=CARTESIAN_POINT('Ctrl Pts',(37.1899557644334,2.19012209252849,-8.2036507409405));
#60443=CARTESIAN_POINT('Ctrl Pts',(37.2008539021761,2.19176392095439,-8.18721955301133));
#60444=CARTESIAN_POINT('Ctrl Pts',(37.2234754037399,2.19512570663176,-8.15400676169728));
#60445=CARTESIAN_POINT('Ctrl Pts',(37.2352134364241,2.19684611030984,-8.13723718048166));
#60446=CARTESIAN_POINT('Ctrl Pts',(37.2656209013829,2.20124440430392,-8.09495460620065));
#60447=CARTESIAN_POINT('Ctrl Pts',(37.2845813141517,2.20393317322019,-8.06965695485378));
#60448=CARTESIAN_POINT('Ctrl Pts',(37.3717017419663,2.21606013277,-7.95807009910218));
#60449=CARTESIAN_POINT('Ctrl Pts',(37.4452215697634,2.22570331528963,-7.87615522060898));
#60450=CARTESIAN_POINT('Ctrl Pts',(37.6264572261133,2.24820534351681,-7.70011969644428));
#60451=CARTESIAN_POINT('Ctrl Pts',(37.7374847918337,2.2611304088081,-7.6099876023341));
#60452=CARTESIAN_POINT('Ctrl Pts',(37.9074439623172,2.27935974725653,-7.49546233371284));
#60453=CARTESIAN_POINT('Ctrl Pts',(37.9603780371533,2.28484033899742,-7.46270435203461));
#60454=CARTESIAN_POINT('Ctrl Pts',(38.0301546941842,2.29176698333998,-7.42318235417618));
#60455=CARTESIAN_POINT('Ctrl Pts',(38.0458801747725,2.2933091781783,-7.41450646901256));
#60456=CARTESIAN_POINT('Ctrl Pts',(38.0717850838821,2.29581729306574,-7.40059065787178));
#60457=CARTESIAN_POINT('Ctrl Pts',(38.0819070091284,2.29678931554823,-7.39524601580351));
#60458=CARTESIAN_POINT('Ctrl Pts',(38.1023918099541,2.2987399133193,-7.38461580272096));
#60459=CARTESIAN_POINT('Ctrl Pts',(38.112755609307,2.29971832801506,-7.37933276029649));
#60460=CARTESIAN_POINT('Ctrl Pts',(38.1399965904096,2.30226913889562,-7.36569447783877));
#60461=CARTESIAN_POINT('Ctrl Pts',(38.1569347406686,2.30383434213327,-7.35746164993201));
#60462=CARTESIAN_POINT('Ctrl Pts',(38.2340531901071,2.31087482251907,-7.32109146531131));
#60463=CARTESIAN_POINT('Ctrl Pts',(38.2952931544834,2.31623146238172,-7.29525255050626));
#60464=CARTESIAN_POINT('Ctrl Pts',(38.4982529209867,2.33348667942382,-7.21936009742986));
#60465=CARTESIAN_POINT('Ctrl Pts',(38.6435999461897,2.34509428941009,-7.18003779688679));
#60466=CARTESIAN_POINT('Ctrl Pts',(38.8897218326058,2.36480386941585,-7.13764173196709));
#60467=CARTESIAN_POINT('Ctrl Pts',(38.9887132419023,2.37274111869828,-7.12685367396695));
#60468=CARTESIAN_POINT('Ctrl Pts',(39.11823065864,2.38333124367357,-7.1208207591722));
#60469=CARTESIAN_POINT('Ctrl Pts',(39.14840478996,2.38581243819792,-7.11998402973177));
#60470=CARTESIAN_POINT('Ctrl Pts',(39.1987690096886,2.38998192404698,-7.11953562874444));
#60471=CARTESIAN_POINT('Ctrl Pts',(39.218953467677,2.39166043870823,-7.11960999609052));
#60472=CARTESIAN_POINT('Ctrl Pts',(39.2588225720517,2.39499212554522,-7.12025872635879));
#60473=CARTESIAN_POINT('Ctrl Pts',(39.2785058557154,2.39664478799011,-7.12082083248984));
#60474=CARTESIAN_POINT('Ctrl Pts',(39.3267985812795,2.40072008215193,-7.12279362081246));
#60475=CARTESIAN_POINT('Ctrl Pts',(39.3553932072862,2.40315081466832,-7.12447377285064));
#60476=CARTESIAN_POINT('Ctrl Pts',(39.4600942375036,2.41212051185402,-7.13250422627305));
#60477=CARTESIAN_POINT('Ctrl Pts',(39.5359078903738,2.41875212388985,-7.14196658403603));
#60478=CARTESIAN_POINT('Ctrl Pts',(39.80305357098,2.44262454135369,-7.18830992634035));
#60479=CARTESIAN_POINT('Ctrl Pts',(39.990190825163,2.46035041432068,-7.2447852724692));
#60480=CARTESIAN_POINT('Ctrl Pts',(40.2163447588134,2.48223817728373,-7.34425862340657));
#60481=CARTESIAN_POINT('Ctrl Pts',(40.2635356283495,2.48682772379357,-7.36687982703521));
#60482=CARTESIAN_POINT('Ctrl Pts',(40.3250359252064,2.49280761512033,-7.39886828823797));
#60483=CARTESIAN_POINT('Ctrl Pts',(40.3400334274706,2.49426574210177,-7.40687211811031));
#60484=CARTESIAN_POINT('Ctrl Pts',(40.3648150163997,2.49667344143415,-7.42043697755966));
#60485=CARTESIAN_POINT('Ctrl Pts',(40.3746469523872,2.49762822761501,-7.4259087447446));
#60486=CARTESIAN_POINT('Ctrl Pts',(40.3935000903804,2.49945773043525,-7.43657503762299));
#60487=CARTESIAN_POINT('Ctrl Pts',(40.4025264827496,2.50033309791933,-7.44175940893857));
#60488=CARTESIAN_POINT('Ctrl Pts',(40.4274594415575,2.50275036958679,-7.45629588280709));
#60489=CARTESIAN_POINT('Ctrl Pts',(40.4432929704987,2.50428465517369,-7.46577294628098));
#60490=CARTESIAN_POINT('Ctrl Pts',(40.5122530818503,2.51097088709593,-7.50813402627492));
#60491=CARTESIAN_POINT('Ctrl Pts',(40.5642014235235,2.51601821113748,-7.54290192720138));
#60492=CARTESIAN_POINT('Ctrl Pts',(40.7392940991964,2.53329113586009,-7.6702373502469));
#60493=CARTESIAN_POINT('Ctrl Pts',(40.8548647744161,2.54518214365506,-7.77257345385189));
#60494=CARTESIAN_POINT('Ctrl Pts',(41.0282355512723,2.56524862155498,-7.95864511090542));
#60495=CARTESIAN_POINT('Ctrl Pts',(41.0919438911289,2.57324798242957,-8.03622299973057));
#60496=CARTESIAN_POINT('Ctrl Pts',(41.1683185965039,2.5839084075277,-8.14207201957113));
#60497=CARTESIAN_POINT('Ctrl Pts',(41.1855525739471,2.58639471806334,-8.16693199462413));
#60498=CARTESIAN_POINT('Ctrl Pts',(41.2135041870448,2.59057037352914,-8.2089218292393));
#60499=CARTESIAN_POINT('Ctrl Pts',(41.2244833609855,2.59224987823744,-8.22587416624515));
#60500=CARTESIAN_POINT('Ctrl Pts',(41.2457372307492,2.59558167789431,-8.25961489071256));
#60501=CARTESIAN_POINT('Ctrl Pts',(41.2560219212059,2.59723344577654,-8.27639513759813));
#60502=CARTESIAN_POINT('Ctrl Pts',(41.278397678395,2.60091776456405,-8.31392903674394));
#60503=CARTESIAN_POINT('Ctrl Pts',(41.2903859627737,2.60295379484999,-8.33474111037115));
#60504=CARTESIAN_POINT('Ctrl Pts',(41.332040008047,2.61025793229785,-8.40962474668539));
#60505=CARTESIAN_POINT('Ctrl Pts',(41.3599328743526,2.615586018623,-8.46464860386458));
#60506=CARTESIAN_POINT('Ctrl Pts',(41.4645727312524,2.63750160600169,-8.69237352344908));
#60507=CARTESIAN_POINT('Ctrl Pts',(41.5229530311541,2.65462238576592,-8.87275268572227));
#60508=CARTESIAN_POINT('Ctrl Pts',(41.5693200356805,2.67594568030793,-9.10706378998762));
#60509=CARTESIAN_POINT('Ctrl Pts',(41.5774887059025,2.68037746307748,-9.15635889992386));
#60510=CARTESIAN_POINT('Ctrl Pts',(41.5885577597293,2.68769016089283,-9.23905373727676));
#60511=CARTESIAN_POINT('Ctrl Pts',(41.5923060428466,2.6905994974062,-9.27232319646403));
#60512=CARTESIAN_POINT('Ctrl Pts',(41.5966780664796,2.69471888713782,-9.3200695371077));
#60513=CARTESIAN_POINT('Ctrl Pts',(41.5978673365949,2.69595564904236,-9.33448879929634));
#60514=CARTESIAN_POINT('Ctrl Pts',(41.5997151919055,2.69810130478685,-9.35966389271286));
#60515=CARTESIAN_POINT('Ctrl Pts',(41.6004317139652,2.69901319622852,-9.37041463186073));
#60516=CARTESIAN_POINT('Ctrl Pts',(41.6018567727451,2.70102127667839,-9.39420443726168));
#60517=CARTESIAN_POINT('Ctrl Pts',(41.6025314155785,2.70211563172631,-9.40724492536064));
#60518=CARTESIAN_POINT('Ctrl Pts',(41.6042173773803,2.70534560309632,-9.44593810331292));
#60519=CARTESIAN_POINT('Ctrl Pts',(41.6049243095676,2.70746570376653,-9.47160329976444));
#60520=CARTESIAN_POINT('Ctrl Pts',(41.6065738043277,2.7191879357727,-9.61470897702045));
#60521=CARTESIAN_POINT('Ctrl Pts',(41.5993254197737,2.72843606174457,-9.73210064877853));
#60522=CARTESIAN_POINT('Ctrl Pts',(41.5672716671839,2.74712650570054,-9.96826495618314));
#60523=CARTESIAN_POINT('Ctrl Pts',(41.542016023149,2.75654285239867,-10.0866206801527));
#60524=CARTESIAN_POINT('Ctrl Pts',(41.4876540373957,2.77191385547458,-10.2717903554194));
#60525=CARTESIAN_POINT('Ctrl Pts',(41.4642320423748,2.77772352532783,-10.3400510679311));
#60526=CARTESIAN_POINT('Ctrl Pts',(41.427732551305,2.78587483961413,-10.4326405225228));
#60527=CARTESIAN_POINT('Ctrl Pts',(41.4172499502583,2.78813214641582,-10.457955610874));
#60528=CARTESIAN_POINT('Ctrl Pts',(41.3985039748555,2.79203456678415,-10.5011250030674));
#60529=CARTESIAN_POINT('Ctrl Pts',(41.390449581311,2.79367256676652,-10.5190675694235));
#60530=CARTESIAN_POINT('Ctrl Pts',(41.3735301656066,2.79703772304248,-10.5555542055835));
#60531=CARTESIAN_POINT('Ctrl Pts',(41.3646456864253,2.798765428518,-10.5740873879471));
#60532=CARTESIAN_POINT('Ctrl Pts',(41.3413130125291,2.80320631500554,-10.6212011895211));
#60533=CARTESIAN_POINT('Ctrl Pts',(41.3265300194785,2.80593080209062,-10.6496103011514));
#60534=CARTESIAN_POINT('Ctrl Pts',(41.2527059332856,2.81913178153162,-10.7848183858992));
#60535=CARTESIAN_POINT('Ctrl Pts',(41.1861720836507,2.82986548364257,-10.8872975554156));
#60536=CARTESIAN_POINT('Ctrl Pts',(41.042029753559,2.85108603930914,-11.0761751482423));
#60537=CARTESIAN_POINT('Ctrl Pts',(40.965361975656,2.86152767489654,-11.1628993664968));
#60538=CARTESIAN_POINT('Ctrl Pts',(40.8466764265417,2.87635892768922,-11.2790978506833));
#60539=CARTESIAN_POINT('Ctrl Pts',(40.8094902412796,2.88083992556557,-11.3132797330393));
#60540=CARTESIAN_POINT('Ctrl Pts',(40.7457159713271,2.88822367138462,-11.3682993823527));
#60541=CARTESIAN_POINT('Ctrl Pts',(40.7197163408817,2.89115548582568,-11.3897930341245));
#60542=CARTESIAN_POINT('Ctrl Pts',(40.6818967002887,2.89530056596648,-11.4197415729925));
#60543=CARTESIAN_POINT('Ctrl Pts',(40.6704403491649,2.89654097812276,-11.4286461517571));
#60544=CARTESIAN_POINT('Ctrl Pts',(40.6502565080986,2.89869893615567,-11.4440433273165));
#60545=CARTESIAN_POINT('Ctrl Pts',(40.6415645851369,2.89961944309052,-11.4505811584148));
#60546=CARTESIAN_POINT('Ctrl Pts',(40.6223265590673,2.90163745378703,-11.4648481993212));
#60547=CARTESIAN_POINT('Ctrl Pts',(40.6117614069294,2.90273318527324,-11.4725506749406));
#60548=CARTESIAN_POINT('Ctrl Pts',(40.5801969774094,2.9059716038225,-11.4951707299223));
#60549=CARTESIAN_POINT('Ctrl Pts',(40.5590194217999,2.90809865386876,-11.5098382239607));
#60550=CARTESIAN_POINT('Ctrl Pts',(40.4491543157507,2.91892497902682,-11.5833472463935));
#60551=CARTESIAN_POINT('Ctrl Pts',(40.3568563933049,2.92733727483172,-11.6366035236715));
#60552=CARTESIAN_POINT('Ctrl Pts',(40.177775259362,2.94300819869835,-11.7246535937927));
#60553=CARTESIAN_POINT('Ctrl Pts',(40.0919152526067,2.9502657037587,-11.7608460022553));
#60554=CARTESIAN_POINT('Ctrl Pts',(39.9064173005675,2.9657819710479,-11.8266486560817));
#60555=CARTESIAN_POINT('Ctrl Pts',(39.8065320427433,2.97404538974445,-11.8549627137646));
#60556=CARTESIAN_POINT('Ctrl Pts',(39.6753126554853,2.98500421534006,-11.8831479188507));
#60557=CARTESIAN_POINT('Ctrl Pts',(39.6453664732119,2.98751145272322,-11.8889865191699));
#60558=CARTESIAN_POINT('Ctrl Pts',(39.5953744137775,2.99171235742035,-11.8977498843862));
#60559=CARTESIAN_POINT('Ctrl Pts',(39.5753874572403,2.99339592300398,-11.9009939279241));
#60560=CARTESIAN_POINT('Ctrl Pts',(39.5359369224703,2.99672829471215,-11.9068868788602));
#60561=CARTESIAN_POINT('Ctrl Pts',(39.5164771107159,2.99837650361494,-11.9095504626825));
#60562=CARTESIAN_POINT('Ctrl Pts',(39.4733134089651,3.00204339664929,-11.9149208903469));
#60563=CARTESIAN_POINT('Ctrl Pts',(39.4495977867655,3.00406544448532,-11.9175139369221));
#60564=CARTESIAN_POINT('Ctrl Pts',(39.3659498788456,3.01122579609411,-11.9254027429996));
#60565=CARTESIAN_POINT('Ctrl Pts',(39.3058665057279,3.01642082563189,-11.9288019110123));
#60566=CARTESIAN_POINT('Ctrl Pts',(39.054815122709,3.03836252028959,-11.9335750476524));
#60567=CARTESIAN_POINT('Ctrl Pts',(38.8641699521223,3.05566399744824,-11.9144581833829));
#60568=CARTESIAN_POINT('Ctrl Pts',(38.6290865921099,3.07716316068664,-11.8621787236908));
#60569=CARTESIAN_POINT('Ctrl Pts',(38.5806876812645,3.08159348705176,-11.8498224571774));
#60570=CARTESIAN_POINT('Ctrl Pts',(38.5005527119162,3.08890408057551,-11.8266833892455));
#60571=CARTESIAN_POINT('Ctrl Pts',(38.4685948646137,3.09181275017041,-11.8167285602401));
#60572=CARTESIAN_POINT('Ctrl Pts',(38.4231341534709,3.09593137776711,-11.801519639642));
#60573=CARTESIAN_POINT('Ctrl Pts',(38.4094565463419,3.09716803149298,-11.7968061742998));
#60574=CARTESIAN_POINT('Ctrl Pts',(38.385667468893,3.09931357409833,-11.7883673052004));
#60575=CARTESIAN_POINT('Ctrl Pts',(38.3755373527822,3.10022545939116,-11.7846969689809));
#60576=CARTESIAN_POINT('Ctrl Pts',(38.3531844220573,3.10223362180757,-11.7764277338521));
#60577=CARTESIAN_POINT('Ctrl Pts',(38.3409739516825,3.10332806399974,-11.7717972174972));
#60578=CARTESIAN_POINT('Ctrl Pts',(38.3048679932787,3.10655853164049,-11.7577675487794));
#60579=CARTESIAN_POINT('Ctrl Pts',(38.2810835991834,3.10867903469059,-11.7480845791094));
#60580=CARTESIAN_POINT('Ctrl Pts',(38.1496523184013,3.12037993405315,-11.6921070144328));
#60581=CARTESIAN_POINT('Ctrl Pts',(38.0453301959829,3.12960803532082,-11.6383690251287));
#60582=CARTESIAN_POINT('Ctrl Pts',(37.8422994730021,3.14827064970736,-11.5142423013542));
#60583=CARTESIAN_POINT('Ctrl Pts',(37.7441649296903,3.15767913845184,-11.443587449918));
#60584=CARTESIAN_POINT('Ctrl Pts',(37.61410778873,3.17121318323613,-11.3342038262312));
#60585=CARTESIAN_POINT('Ctrl Pts',(37.5774445880302,3.17516038082164,-11.301396906555));
#60586=CARTESIAN_POINT('Ctrl Pts',(37.5135677938224,3.18231110088138,-11.2406106225289));
#60587=CARTESIAN_POINT('Ctrl Pts',(37.4859802322696,3.18549806088249,-11.2130489595003));
#60588=CARTESIAN_POINT('Ctrl Pts',(37.4439103533145,3.19052645065066,-11.1689236983109));
#60589=CARTESIAN_POINT('Ctrl Pts',(37.4289637705724,3.19234799799168,-11.1528103639527));
#60590=CARTESIAN_POINT('Ctrl Pts',(37.4013503441521,3.19578177623449,-11.1222108675222));
#60591=CARTESIAN_POINT('Ctrl Pts',(37.388632370381,3.19739170338147,-11.1077730110408));
#60592=CARTESIAN_POINT('Ctrl Pts',(37.3602800951101,3.20104704679235,-11.0747972902538));
#60593=CARTESIAN_POINT('Ctrl Pts',(37.3447504397159,3.20309649067993,-11.0561727354721));
#60594=CARTESIAN_POINT('Ctrl Pts',(37.2974130739272,3.20949556626997,-10.997623992221));
#60595=CARTESIAN_POINT('Ctrl Pts',(37.2665949206866,3.21388286375077,-10.956922621696));
#60596=CARTESIAN_POINT('Ctrl Pts',(37.0899392284347,3.24043460056447,-10.7075057900208));
#60597=CARTESIAN_POINT('Ctrl Pts',(36.9767368538911,3.2637794990598,-10.4777499316654));
#60598=CARTESIAN_POINT('Ctrl Pts',(36.891414135039,3.28915317443388,-10.2013801046984));
#60599=CARTESIAN_POINT('Ctrl Pts',(36.8818896588773,3.29217342893363,-10.1679802144486));
#60600=CARTESIAN_POINT('Ctrl Pts',(36.8693743213068,3.29641935880466,-10.1201908361976));
#60601=CARTESIAN_POINT('Ctrl Pts',(36.8657872940401,3.29767393292135,-10.1059640805097));
#60602=CARTESIAN_POINT('Ctrl Pts',(36.8597875743348,3.29983908640797,-10.0812151097051));
#60603=CARTESIAN_POINT('Ctrl Pts',(36.8573152090592,3.30075284748551,-10.0707081963452));
#60604=CARTESIAN_POINT('Ctrl Pts',(36.8520394891498,3.30275123796868,-10.0475908892303));
#60605=CARTESIAN_POINT('Ctrl Pts',(36.8492668711495,3.3038341714507,-10.0349740960656));
#60606=CARTESIAN_POINT('Ctrl Pts',(36.8415860633585,3.30693329365437,-9.99862829392094));
#60607=CARTESIAN_POINT('Ctrl Pts',(36.8369344027082,3.30893609846142,-9.97484572570892));
#60608=CARTESIAN_POINT('Ctrl Pts',(36.8074751123295,3.32257738167504,-9.81113353129821));
#60609=CARTESIAN_POINT('Ctrl Pts',(36.7947474293012,3.33367977743677,-9.66929336068567));
#60610=CARTESIAN_POINT('Ctrl Pts',(36.7944892164701,3.35641233410546,-9.37907680549902));
#60611=CARTESIAN_POINT('Ctrl Pts',(36.80802812903,3.36800478182511,-9.23133637198126));
#60612=CARTESIAN_POINT('Ctrl Pts',(36.84198593651,3.3830928610062,-9.04848998766378));
#60613=CARTESIAN_POINT('Ctrl Pts',(36.8497939599075,3.38619426873979,-9.01136260794192));
#60614=CARTESIAN_POINT('Ctrl Pts',(36.8635058466313,3.39113525916292,-8.95304643214434));
#60615=CARTESIAN_POINT('Ctrl Pts',(36.8688282008873,3.39295651163367,-8.9317262103934));
#60616=CARTESIAN_POINT('Ctrl Pts',(36.879310401868,3.39637473771534,-8.8920577326374));
#60617=CARTESIAN_POINT('Ctrl Pts',(36.88439772532,3.39796927828872,-8.87369194248652));
#60618=CARTESIAN_POINT('Ctrl Pts',(36.8964278011807,3.40160129842417,-8.83218566949044));
#60619=CARTESIAN_POINT('Ctrl Pts',(36.9035019326672,3.40364285899994,-8.80908582430155));
#60620=CARTESIAN_POINT('Ctrl Pts',(36.9253278805252,3.40968081381714,-8.74147030742588));
#60621=CARTESIAN_POINT('Ctrl Pts',(36.9410338389479,3.41370727263283,-8.69727835980132));
#60622=CARTESIAN_POINT('Ctrl Pts',(36.9580196850403,3.41777315288062,-8.65357747806631));
#60623=CARTESIAN_POINT('',(36.7973459100127,3.61022481984855,-9.52397861444782));
#60624=CARTESIAN_POINT('Ctrl Pts',(36.958019684865,3.68510631127449,-8.65357747851728));
#60625=CARTESIAN_POINT('Ctrl Pts',(36.9262879380075,3.67770817542144,-8.73521635066666));
#60626=CARTESIAN_POINT('Ctrl Pts',(36.8989808726309,3.67031003956838,-8.81868899500876));
#60627=CARTESIAN_POINT('Ctrl Pts',(36.8762923251079,3.66291190371533,-8.90352145165943));
#60628=CARTESIAN_POINT('Ctrl Pts',(36.8536674274252,3.65553452239341,-8.98811592162024));
#60629=CARTESIAN_POINT('Ctrl Pts',(36.8356353245951,3.6481571410715,-9.0740623070127));
#60630=CARTESIAN_POINT('Ctrl Pts',(36.8223411254775,3.64077975974958,-9.16086922568368));
#60631=CARTESIAN_POINT('Ctrl Pts',(36.8091047566171,3.63343447030892,-9.24729853105196));
#60632=CARTESIAN_POINT('Ctrl Pts',(36.8005652812803,3.62608918086826,-9.33458060440531));
#60633=CARTESIAN_POINT('Ctrl Pts',(36.7968171360163,3.6187438914276,-9.42221348991686));
#60634=CARTESIAN_POINT('Ctrl Pts',(36.7953681022262,3.61590420090125,-9.45609238288551));
#60635=CARTESIAN_POINT('Ctrl Pts',(36.7946346513946,3.6130645103749,-9.49002355151977));
#60636=CARTESIAN_POINT('Ctrl Pts',(36.7946202173455,3.61022481984855,-9.52397745573624));
#60637=CARTESIAN_POINT('Ctrl Pts',(36.79802585967,3.61022481984855,-9.52397890349931));
#60638=CARTESIAN_POINT('Ctrl Pts',(36.7998206443408,3.57126194121243,-9.98919550479405));
#60639=CARTESIAN_POINT('Ctrl Pts',(37.1539181706817,3.46543046208966,-11.2553513949631));
#60640=CARTESIAN_POINT('Ctrl Pts',(39.199922352963,3.29273038248022,-12.3631804573943));
#60641=CARTESIAN_POINT('Ctrl Pts',(41.5765986432995,3.09212458102024,-11.0764707285289));
#60642=CARTESIAN_POINT('Ctrl Pts',(41.7982659728439,2.89151877956026,-8.38294215354648));
#60643=CARTESIAN_POINT('Ctrl Pts',(39.663923518907,2.69091297810028,-6.72499042239298));
#60644=CARTESIAN_POINT('Ctrl Pts',(37.641017118746,2.53208515608523,-7.42250632947195));
#60645=CARTESIAN_POINT('Ctrl Pts',(37.0674493624832,2.44012593455684,-8.37484768228411));
#60646=CARTESIAN_POINT('Ctrl Pts',(36.9607077789649,2.41503531351511,-8.65459504792142));
#60647=CARTESIAN_POINT('Origin',(39.2,8.05522481984854,-9.525));
#60648=CARTESIAN_POINT('',(36.9547201749638,0.879636998740377,-8.65231241759342));
#60649=CARTESIAN_POINT('',(36.9580194911167,1.14613690893122,-8.65357797698964));
#60650=CARTESIAN_POINT('',(36.958019684865,8.05522481984854,-8.65357747851728));
#60651=CARTESIAN_POINT('',(36.7916962852456,2.07477346687626,-9.52369325357238));
#60652=CARTESIAN_POINT('Ctrl Pts',(36.7916962852457,2.07477346687626,-9.52369325357238));
#60653=CARTESIAN_POINT('Ctrl Pts',(36.7964605736323,2.01459014677707,-10.2374555183397));
#60654=CARTESIAN_POINT('Ctrl Pts',(37.5094020732034,1.88753822619121,-11.7525226440311));
#60655=CARTESIAN_POINT('Ctrl Pts',(40.0791495164278,1.69361770511871,-12.2235884022735));
#60656=CARTESIAN_POINT('Ctrl Pts',(41.9403077448524,1.49301190365872,-10.2639158886558));
#60657=CARTESIAN_POINT('Ctrl Pts',(41.3166585082413,1.29240610219874,-7.63422238696309));
#60658=CARTESIAN_POINT('Ctrl Pts',(38.7737033595216,1.09180030073876,-6.7190145399589));
#60659=CARTESIAN_POINT('Ctrl Pts',(37.294687387309,0.954210599585968,-7.83640380397085));
#60660=CARTESIAN_POINT('Ctrl Pts',(36.9710594620979,0.88348949891984,-8.60967633348487));
#60661=CARTESIAN_POINT('Ctrl Pts',(36.9547201749638,0.879636998740377,-8.65231241759342));
#60662=CARTESIAN_POINT('Ctrl Pts',(36.794620288083,2.0764482978049,-9.52382275830541));
#60663=CARTESIAN_POINT('Ctrl Pts',(36.7946428644169,2.08053459401905,-9.47769403564713));
#60664=CARTESIAN_POINT('Ctrl Pts',(36.795992380219,2.08458592142556,-9.43157101659339));
#60665=CARTESIAN_POINT('Ctrl Pts',(36.7995253989188,2.08986157364004,-9.37074928543718));
#60666=CARTESIAN_POINT('Ctrl Pts',(36.8005190234597,2.09113613178648,-9.3559950638613));
#60667=CARTESIAN_POINT('Ctrl Pts',(36.8024798154703,2.09333694017497,-9.33040225457211));
#60668=CARTESIAN_POINT('Ctrl Pts',(36.8033845640459,2.09426620326653,-9.31955953697378));
#60669=CARTESIAN_POINT('Ctrl Pts',(36.8053203262713,2.09609718322561,-9.29811766302057));
#60670=CARTESIAN_POINT('Ctrl Pts',(36.8063482070305,2.09699900452055,-9.28751852994192));
#60671=CARTESIAN_POINT('Ctrl Pts',(36.8087549017492,2.09896655299799,-9.26430713581487));
#60672=CARTESIAN_POINT('Ctrl Pts',(36.8101631450801,2.10003067570489,-9.25169848376381));
#60673=CARTESIAN_POINT('Ctrl Pts',(36.814422852703,2.10302222684463,-9.21611393439659));
#60674=CARTESIAN_POINT('Ctrl Pts',(36.8175064546258,2.10493765608338,-9.19316637618662));
#60675=CARTESIAN_POINT('Ctrl Pts',(36.8354221411912,2.11491213688721,-9.07301214974332));
#60676=CARTESIAN_POINT('Ctrl Pts',(36.8558750695435,2.12271844780597,-8.97672529577101));
#60677=CARTESIAN_POINT('Ctrl Pts',(36.9036373782248,2.1367776473617,-8.80456946622985));
#60678=CARTESIAN_POINT('Ctrl Pts',(36.9289561748562,2.14304029044836,-8.72835153425556));
#60679=CARTESIAN_POINT('Ctrl Pts',(36.9580197803105,2.14933799730903,-8.65357723295689));
#60680=CARTESIAN_POINT('',(36.7950466582253,2.34022481984855,-9.5271366580497));
#60681=CARTESIAN_POINT('Ctrl Pts',(36.9607077789649,2.41503531351511,-8.65459504792142));
#60682=CARTESIAN_POINT('Ctrl Pts',(36.8546204546155,2.39009848229292,-8.93262773711423));
#60683=CARTESIAN_POINT('Ctrl Pts',(36.7976786392064,2.36516165107074,-9.23032286919603));
#60684=CARTESIAN_POINT('Ctrl Pts',(36.7950466582253,2.34022481984855,-9.5271366580497));
#60685=CARTESIAN_POINT('Ctrl Pts',(36.7946209688343,2.34046868728881,-9.52715889521613));
#60686=CARTESIAN_POINT('Ctrl Pts',(36.7947400435394,2.32857689585436,-9.65982851088632));
#60687=CARTESIAN_POINT('Ctrl Pts',(36.8058349123456,2.31658147687662,-9.79226876623499));
#60688=CARTESIAN_POINT('Ctrl Pts',(36.8326453211439,2.30230139713442,-9.95201625881918));
#60689=CARTESIAN_POINT('Ctrl Pts',(36.8380214776574,2.29973526653512,-9.98081653738562));
#60690=CARTESIAN_POINT('Ctrl Pts',(36.8472368487234,2.29576207067078,-10.0256288057932));
#60691=CARTESIAN_POINT('Ctrl Pts',(36.8507163628563,2.29434017072281,-10.0417108301057));
#60692=CARTESIAN_POINT('Ctrl Pts',(36.8575826305807,2.29167626734596,-10.0719418772506));
#60693=CARTESIAN_POINT('Ctrl Pts',(36.8609332432784,2.29043256879513,-10.0860982893243));
#60694=CARTESIAN_POINT('Ctrl Pts',(36.8670133040976,2.28827123833547,-10.1107852223474));
#60695=CARTESIAN_POINT('Ctrl Pts',(36.8696860356687,2.28735060939581,-10.1213288498563));
#60696=CARTESIAN_POINT('Ctrl Pts',(36.8757206103207,2.2853351795214,-10.1444742459952));
#60697=CARTESIAN_POINT('Ctrl Pts',(36.879113528385,2.28424212113316,-10.157067269333));
#60698=CARTESIAN_POINT('Ctrl Pts',(36.8894696904373,2.28101929473666,-10.1942966639199));
#60699=CARTESIAN_POINT('Ctrl Pts',(36.8967242909894,2.27890494375835,-10.2188512116662));
#60700=CARTESIAN_POINT('Ctrl Pts',(36.9401666988732,2.26698823476297,-10.3576922777341));
#60701=CARTESIAN_POINT('Ctrl Pts',(36.9844711293871,2.25755590213781,-10.4692791894704));
#60702=CARTESIAN_POINT('Ctrl Pts',(37.0894571621821,2.23873678258408,-10.6851246198109));
#60703=CARTESIAN_POINT('Ctrl Pts',(37.1500083590448,2.22937425769,-10.7890459768646));
#60704=CARTESIAN_POINT('Ctrl Pts',(37.2454061747055,2.21595826891165,-10.9277629845139));
#60705=CARTESIAN_POINT('Ctrl Pts',(37.2739353778813,2.21208423479084,-10.9666849705437));
#60706=CARTESIAN_POINT('Ctrl Pts',(37.3268187951704,2.20511005077166,-11.0344594979671));
#60707=CARTESIAN_POINT('Ctrl Pts',(37.3507185338563,2.20202651123457,-11.0636466626651));
#60708=CARTESIAN_POINT('Ctrl Pts',(37.376616078177,2.19874870273732,-11.0937983105499));
#60709=CARTESIAN_POINT('Ctrl Pts',(37.377940737037,2.19858121299482,-11.0953366224305));
#60710=CARTESIAN_POINT('Ctrl Pts',(37.3805377062933,2.1982531833163,-11.098344744584));
#60711=CARTESIAN_POINT('Ctrl Pts',(37.3818098545768,2.19809264985278,-11.0998146934072));
#60712=CARTESIAN_POINT('Ctrl Pts',(37.384322461092,2.19777588533278,-11.1027108708453));
#60713=CARTESIAN_POINT('Ctrl Pts',(37.3855628214642,2.1976196582312,-11.1041371828893));
#60714=CARTESIAN_POINT('Ctrl Pts',(37.3880323178237,2.19730890486403,-11.1069701490903));
#60715=CARTESIAN_POINT('Ctrl Pts',(37.3892614138223,2.19715438026564,-11.1083768364957));
#60716=CARTESIAN_POINT('Ctrl Pts',(37.4038685189948,2.19531960547662,-11.1250552630066));
#60717=CARTESIAN_POINT('Ctrl Pts',(37.4174372874199,2.19363176324731,-11.1401579689667));
#60718=CARTESIAN_POINT('Ctrl Pts',(37.4444732105396,2.19029928296955,-11.169494612909));
#60719=CARTESIAN_POINT('Ctrl Pts',(37.4579263597775,2.1886553204599,-11.1837393477971));
#60720=CARTESIAN_POINT('Ctrl Pts',(37.4880158575952,2.18500837523973,-11.2148294922942));
#60721=CARTESIAN_POINT('Ctrl Pts',(37.504729710748,2.18300215677346,-11.2315966064477));
#60722=CARTESIAN_POINT('Ctrl Pts',(37.5639278293328,2.17596113548381,-11.2892555601365));
#60723=CARTESIAN_POINT('Ctrl Pts',(37.6076623265019,2.17087207545387,-11.328826292137));
#60724=CARTESIAN_POINT('Ctrl Pts',(37.7986801406776,2.14908601010405,-11.4892947424074));
#60725=CARTESIAN_POINT('Ctrl Pts',(37.9585879618252,2.13183066697992,-11.5940642144541));
#60726=CARTESIAN_POINT('Ctrl Pts',(38.1749984932429,2.11024416202486,-11.7016597976445));
#60727=CARTESIAN_POINT('Ctrl Pts',(38.2215783796094,2.10569755735421,-11.7229917733082));
#60728=CARTESIAN_POINT('Ctrl Pts',(38.3002127148904,2.09821943068981,-11.7560078408592));
#60729=CARTESIAN_POINT('Ctrl Pts',(38.3318974393323,2.09525797090332,-11.7685265627328));
#60730=CARTESIAN_POINT('Ctrl Pts',(38.3774933685387,2.09107921806147,-11.7854308952045));
#60731=CARTESIAN_POINT('Ctrl Pts',(38.3911932595905,2.08983419461535,-11.7903689943565));
#60732=CARTESIAN_POINT('Ctrl Pts',(38.4152044322017,2.08767142175088,-11.7987781764741));
#60733=CARTESIAN_POINT('Ctrl Pts',(38.4254956018953,2.08675066153383,-11.8023041597437));
#60734=CARTESIAN_POINT('Ctrl Pts',(38.4481667503727,2.08473597486478,-11.8099003285157));
#60735=CARTESIAN_POINT('Ctrl Pts',(38.4605563330619,2.08364378054945,-11.813939893098));
#60736=CARTESIAN_POINT('Ctrl Pts',(38.4965974030559,2.08049039012895,-11.8253677239408));
#60737=CARTESIAN_POINT('Ctrl Pts',(38.5203319403836,2.07844330623803,-11.8324917882686));
#60738=CARTESIAN_POINT('Ctrl Pts',(38.6953177431574,2.06353687657041,-11.8820803705232));
#60739=CARTESIAN_POINT('Ctrl Pts',(38.8503192082428,2.05133023528189,-11.910009688668));
#60740=CARTESIAN_POINT('Ctrl Pts',(39.1023961537837,2.03151271800208,-11.9303053486253));
#60741=CARTESIAN_POINT('Ctrl Pts',(39.198200580388,2.02399169609359,-11.9322837239946));
#60742=CARTESIAN_POINT('Ctrl Pts',(39.3558562700161,2.01136816840761,-11.9261269886454));
#60743=CARTESIAN_POINT('Ctrl Pts',(39.4177273710073,2.00635210580562,-11.921308734444));
#60744=CARTESIAN_POINT('Ctrl Pts',(39.5051753835021,1.9991301002889,-11.9110841569755));
#60745=CARTESIAN_POINT('Ctrl Pts',(39.5309605774057,1.99698425681486,-11.9076444568596));
#60746=CARTESIAN_POINT('Ctrl Pts',(39.5759126191522,1.99321171537021,-11.9009041864067));
#60747=CARTESIAN_POINT('Ctrl Pts',(39.5951050407562,1.99159088401517,-11.8977880141869));
#60748=CARTESIAN_POINT('Ctrl Pts',(39.634978845187,1.98820109927326,-11.8908167445802));
#60749=CARTESIAN_POINT('Ctrl Pts',(39.6556515518141,1.9864310434394,-11.8869223246682));
#60750=CARTESIAN_POINT('Ctrl Pts',(39.7099895429765,1.98174354492301,-11.8759459850876));
#60751=CARTESIAN_POINT('Ctrl Pts',(39.743557288639,1.97881220858396,-11.8684123773041));
#60752=CARTESIAN_POINT('Ctrl Pts',(39.9665430338727,1.95908893346371,-11.8133191295738));
#60753=CARTESIAN_POINT('Ctrl Pts',(40.1496872105402,1.94158340537125,-11.7435701355292));
#60754=CARTESIAN_POINT('Ctrl Pts',(40.4114493899048,1.91500294868688,-11.6054790185491));
#60755=CARTESIAN_POINT('Ctrl Pts',(40.4975245077499,1.90599068977397,-11.5529144923378));
#60756=CARTESIAN_POINT('Ctrl Pts',(40.6009303788976,1.8949959212425,-11.4804785886176));
#60757=CARTESIAN_POINT('Ctrl Pts',(40.6215713004806,1.89279258676314,-11.4655250918808));
#60758=CARTESIAN_POINT('Ctrl Pts',(40.6523918657946,1.88949375288289,-11.4424410805384));
#60759=CARTESIAN_POINT('Ctrl Pts',(40.6627487109272,1.88838367714842,-11.4345519532382));
#60760=CARTESIAN_POINT('Ctrl Pts',(40.6816425666914,1.88635645907412,-11.4199159937446));
#60761=CARTESIAN_POINT('Ctrl Pts',(40.6901982555449,1.8854377494618,-11.4131950344742));
#60762=CARTESIAN_POINT('Ctrl Pts',(40.7099156294973,1.8833184244059,-11.3974884593112));
#60763=CARTESIAN_POINT('Ctrl Pts',(40.7210430674846,1.88212074200149,-11.388460827825));
#60764=CARTESIAN_POINT('Ctrl Pts',(40.7569443769672,1.87824860134461,-11.3587984131553));
#60765=CARTESIAN_POINT('Ctrl Pts',(40.7813855826859,1.875599986479,-11.3377637334425));
#60766=CARTESIAN_POINT('Ctrl Pts',(40.9313434889073,1.85921399351496,-11.2033642007105));
#60767=CARTESIAN_POINT('Ctrl Pts',(41.0450496829803,1.84615659445709,-11.0775024878716));
#60768=CARTESIAN_POINT('Ctrl Pts',(41.1923623961085,1.8264958525073,-10.8751573614344));
#60769=CARTESIAN_POINT('Ctrl Pts',(41.2367538226658,1.82008883345694,-10.8072109784109));
#60770=CARTESIAN_POINT('Ctrl Pts',(41.3057046993631,1.80910655403755,-10.6890297457104));
#60771=CARTESIAN_POINT('Ctrl Pts',(41.3321004271938,1.80458972089338,-10.6399459078541));
#60772=CARTESIAN_POINT('Ctrl Pts',(41.3678497161436,1.79795891390863,-10.5675484016691));
#60773=CARTESIAN_POINT('Ctrl Pts',(41.3785814092291,1.79589195075207,-10.5449326001782));
#60774=CARTESIAN_POINT('Ctrl Pts',(41.3969648497864,1.79220871283113,-10.5045771845527));
#60775=CARTESIAN_POINT('Ctrl Pts',(41.4047596375407,1.79059744226602,-10.4869048323351));
#60776=CARTESIAN_POINT('Ctrl Pts',(41.4207793502108,1.7871772575346,-10.4493669463424));
#60777=CARTESIAN_POINT('Ctrl Pts',(41.4289523786941,1.78536676824761,-10.4294812894409));
#60778=CARTESIAN_POINT('Ctrl Pts',(41.450336383206,1.7804449708229,-10.3754015358862));
#60779=CARTESIAN_POINT('Ctrl Pts',(41.4630334829072,1.77731713565773,-10.3410121004777));
#60780=CARTESIAN_POINT('Ctrl Pts',(41.549789634235,1.75434161588809,-10.0884166133304));
#60781=CARTESIAN_POINT('Ctrl Pts',(41.5929222463608,1.73346997903445,-9.86089314047946));
#60782=CARTESIAN_POINT('Ctrl Pts',(41.6052362710042,1.70847865178618,-9.5811874317746));
#60783=CARTESIAN_POINT('Ctrl Pts',(41.6058837690946,1.70407382780111,-9.5315213236654));
#60784=CARTESIAN_POINT('Ctrl Pts',(41.6043955371354,1.69680023428862,-9.44854006518988));
#60785=CARTESIAN_POINT('Ctrl Pts',(41.6031050839378,1.6939033911853,-9.41522611723576));
#60786=CARTESIAN_POINT('Ctrl Pts',(41.6002635290381,1.68979846725851,-9.36753093260855));
#60787=CARTESIAN_POINT('Ctrl Pts',(41.5992747830038,1.68856391772154,-9.35312195010786));
#60788=CARTESIAN_POINT('Ctrl Pts',(41.5973146181204,1.68641249807119,-9.32788662092796));
#60789=CARTESIAN_POINT('Ctrl Pts',(41.5963995258212,1.6854927261872,-9.31705675260254));
#60790=CARTESIAN_POINT('Ctrl Pts',(41.5942180559602,1.6834719550875,-9.29317056336822));
#60791=CARTESIAN_POINT('Ctrl Pts',(41.5929182561159,1.68237277178815,-9.28011792335826));
#60792=CARTESIAN_POINT('Ctrl Pts',(41.5888108421018,1.6791786552033,-9.24203332268636));
#60793=CARTESIAN_POINT('Ctrl Pts',(41.5857166348505,1.67709839029302,-9.21703300455705));
#60794=CARTESIAN_POINT('Ctrl Pts',(41.5655314131988,1.66515052520939,-9.07259445664102));
#60795=CARTESIAN_POINT('Ctrl Pts',(41.5398635816816,1.6556590586849,-8.95451196636151));
#60796=CARTESIAN_POINT('Ctrl Pts',(41.4706339600697,1.63663195974076,-8.72190661007857));
#60797=CARTESIAN_POINT('Ctrl Pts',(41.4269877301973,1.62712194190069,-8.60779730773873));
#60798=CARTESIAN_POINT('Ctrl Pts',(41.3453788571499,1.61188543873575,-8.43505925195847));
#60799=CARTESIAN_POINT('Ctrl Pts',(41.3132094432504,1.60631773809732,-8.37392855113639));
#60800=CARTESIAN_POINT('Ctrl Pts',(41.2648701004603,1.59844866979959,-8.2909444207743));
#60801=CARTESIAN_POINT('Ctrl Pts',(41.2508909531929,1.59622379619392,-8.26784929972541));
#60802=CARTESIAN_POINT('Ctrl Pts',(41.2260987123891,1.59235970099989,-8.22840408735314));
#60803=CARTESIAN_POINT('Ctrl Pts',(41.215468751679,1.5907272275393,-8.21194150309085));
#60804=CARTESIAN_POINT('Ctrl Pts',(41.1932141706266,1.587357235067,-8.17838292145843));
#60805=CARTESIAN_POINT('Ctrl Pts',(41.1815679505563,1.58561901852911,-8.16130330117273));
#60806=CARTESIAN_POINT('Ctrl Pts',(41.1509760454334,1.58111573552117,-8.11765854293112));
#60807=CARTESIAN_POINT('Ctrl Pts',(41.1317080156562,1.57833872179343,-8.09132590019964));
#60808=CARTESIAN_POINT('Ctrl Pts',(41.0306625536036,1.56406150524204,-7.95896822861512));
#60809=CARTESIAN_POINT('Ctrl Pts',(40.9406851150666,1.55224732558697,-7.8595320174475));
#60810=CARTESIAN_POINT('Ctrl Pts',(40.750125645472,1.52889044449982,-7.68133382446457));
#60811=CARTESIAN_POINT('Ctrl Pts',(40.6505987696114,1.51740312845915,-7.60204421639064));
#60812=CARTESIAN_POINT('Ctrl Pts',(40.5008249878311,1.50138781696076,-7.50099847548984));
#60813=CARTESIAN_POINT('Ctrl Pts',(40.4553818979142,1.49668121011021,-7.47250267337171));
#60814=CARTESIAN_POINT('Ctrl Pts',(40.3942068344256,1.49057579774779,-7.43693472807056));
#60815=CARTESIAN_POINT('Ctrl Pts',(40.3793015829086,1.48910573290188,-7.42848041460376));
#60816=CARTESIAN_POINT('Ctrl Pts',(40.3544395103012,1.48668401037931,-7.41472762135667));
#60817=CARTESIAN_POINT('Ctrl Pts',(40.3445337450035,1.48572701258392,-7.40933872654418));
#60818=CARTESIAN_POINT('Ctrl Pts',(40.3241425892816,1.48377363709274,-7.39843075236286));
#60819=CARTESIAN_POINT('Ctrl Pts',(40.3136536933724,1.48277770722045,-7.39291913943464));
#60820=CARTESIAN_POINT('Ctrl Pts',(40.2854896298321,1.48012590913586,-7.3783842895138));
#60821=CARTESIAN_POINT('Ctrl Pts',(40.2677422823334,1.4784783038809,-7.36950162559412));
#60822=CARTESIAN_POINT('Ctrl Pts',(40.1730821743144,1.46980254836655,-7.3235797439198));
#60823=CARTESIAN_POINT('Ctrl Pts',(40.0943382913222,1.46297378865537,-7.29043000036356));
#60824=CARTESIAN_POINT('Ctrl Pts',(39.8701178196111,1.44413333011074,-7.20979578049084));
#60825=CARTESIAN_POINT('Ctrl Pts',(39.7216439673208,1.43231794383814,-7.1718920591141));
#60826=CARTESIAN_POINT('Ctrl Pts',(39.4914572436794,1.41381968701357,-7.13600072593955));
#60827=CARTESIAN_POINT('Ctrl Pts',(39.4117806685749,1.40738939731695,-7.12762406269919));
#60828=CARTESIAN_POINT('Ctrl Pts',(39.3035473351996,1.39852002183734,-7.12168273460529));
#60829=CARTESIAN_POINT('Ctrl Pts',(39.2752289765789,1.39618728925874,-7.12062973052066));
#60830=CARTESIAN_POINT('Ctrl Pts',(39.2270738331035,1.39219595757192,-7.11969062893248));
#60831=CARTESIAN_POINT('Ctrl Pts',(39.2072444800568,1.39054534688547,-7.11954918338567));
#60832=CARTESIAN_POINT('Ctrl Pts',(39.1671253505563,1.3871902028988,-7.11975906946439));
#60833=CARTESIAN_POINT('Ctrl Pts',(39.1468372859804,1.38548544821828,-7.12012196809199));
#60834=CARTESIAN_POINT('Ctrl Pts',(39.0958297425447,1.38117766932851,-7.12168010022112));
#60835=CARTESIAN_POINT('Ctrl Pts',(39.0651250060043,1.37856465251525,-7.12320764195388));
#60836=CARTESIAN_POINT('Ctrl Pts',(38.935328691325,1.36742857749919,-7.13216157729807));
#60837=CARTESIAN_POINT('Ctrl Pts',(38.8367324454893,1.35874062211037,-7.14513493868336));
#60838=CARTESIAN_POINT('Ctrl Pts',(38.5891036736733,1.33634060039277,-7.19346483389981));
#60839=CARTESIAN_POINT('Ctrl Pts',(38.4421211043393,1.32248009416662,-7.23701700237172));
#60840=CARTESIAN_POINT('Ctrl Pts',(38.2408367716864,1.30316217524171,-7.31819998710583));
#60841=CARTESIAN_POINT('Ctrl Pts',(38.1823746023508,1.29751290078044,-7.34454115449899));
#60842=CARTESIAN_POINT('Ctrl Pts',(38.1088234542154,1.29040976336842,-7.38128480584249));
#60843=CARTESIAN_POINT('Ctrl Pts',(38.0927095441383,1.28885389201232,-7.38956351182441));
#60844=CARTESIAN_POINT('Ctrl Pts',(38.0665414744774,1.2863294944245,-7.40338353292633));
#60845=CARTESIAN_POINT('Ctrl Pts',(38.0564311078605,1.28535471802544,-7.40881596495931));
#60846=CARTESIAN_POINT('Ctrl Pts',(38.0374174653899,1.28352312061498,-7.41920830906761));
#60847=CARTESIAN_POINT('Ctrl Pts',(38.0285061678416,1.28266534038573,-7.42415278788716));
#60848=CARTESIAN_POINT('Ctrl Pts',(38.0045508123893,1.28036045163073,-7.43764436599053));
#60849=CARTESIAN_POINT('Ctrl Pts',(37.9895666910195,1.2789198076572,-7.44629762567028));
#60850=CARTESIAN_POINT('Ctrl Pts',(37.9308171218171,1.27327009498406,-7.48107594702161));
#60851=CARTESIAN_POINT('Ctrl Pts',(37.8877895037524,1.26912945984383,-7.50842980071317));
#60852=CARTESIAN_POINT('Ctrl Pts',(37.7222553254481,1.25305002445776,-7.6212087952406));
#60853=CARTESIAN_POINT('Ctrl Pts',(37.6069383231159,1.24149802493233,-7.71659951976353));
#60854=CARTESIAN_POINT('Ctrl Pts',(37.4460946917407,1.22363652651139,-7.87705317692599));
#60855=CARTESIAN_POINT('Ctrl Pts',(37.3936895317247,1.21747970701409,-7.93466874949074));
#60856=CARTESIAN_POINT('Ctrl Pts',(37.3096939639634,1.20687369954705,-8.03653327829339));
#60857=CARTESIAN_POINT('Ctrl Pts',(37.2766410287909,1.20247743860365,-8.07949679830634));
#60858=CARTESIAN_POINT('Ctrl Pts',(37.2306305190634,1.19599026716638,-8.14367783178097));
#60859=CARTESIAN_POINT('Ctrl Pts',(37.2165043843074,1.19394344969863,-8.16403999542309));
#60860=CARTESIAN_POINT('Ctrl Pts',(37.1919482985418,1.19028258389804,-8.20063098099402));
#60861=CARTESIAN_POINT('Ctrl Pts',(37.1813940562603,1.18867332143248,-8.21677412790836));
#60862=CARTESIAN_POINT('Ctrl Pts',(37.159413160891,1.18524317847799,-8.25129417979092));
#60863=CARTESIAN_POINT('Ctrl Pts',(37.1480381649779,1.18342058771624,-8.26970173809325));
#60864=CARTESIAN_POINT('Ctrl Pts',(37.1177171145653,1.17842825877582,-8.32028224180602));
#60865=CARTESIAN_POINT('Ctrl Pts',(37.0992701728661,1.17524116478516,-8.35274544119012));
#60866=CARTESIAN_POINT('Ctrl Pts',(37.03491536889,1.16354744521854,-8.47239857175206));
#60867=CARTESIAN_POINT('Ctrl Pts',(36.9936571723966,1.15489698158361,-8.56188992607809));
#60868=CARTESIAN_POINT('Ctrl Pts',(36.9580194911167,1.14613690893122,-8.65357797698964));
#60869=CARTESIAN_POINT('Origin',(39.2,8.05522481984854,-9.525));
#60870=CARTESIAN_POINT('',(36.9580196850438,-0.392176638896471,-8.65357747805726));
#60871=CARTESIAN_POINT('',(36.958019684865,-0.127039975641408,-8.65357747851736));
#60872=CARTESIAN_POINT('',(36.958019684865,8.05522481984854,-8.65357747851728));
#60873=CARTESIAN_POINT('',(36.7978958045452,0.804628829011641,-9.52411276591516));
#60874=CARTESIAN_POINT('Ctrl Pts',(36.9580196850438,-0.392176638896471,
-8.65357747805726));
#60875=CARTESIAN_POINT('Ctrl Pts',(36.9824700011476,-0.386309940922915,
-8.59067214107231));
#60876=CARTESIAN_POINT('Ctrl Pts',(37.0095550481929,-0.380366550251713,
-8.52882859886102));
#60877=CARTESIAN_POINT('Ctrl Pts',(37.0798337986663,-0.366146063000361,
-8.38513105426349));
#60878=CARTESIAN_POINT('Ctrl Pts',(37.1252210655968,-0.357829720603997,
-8.30446870225221));
#60879=CARTESIAN_POINT('Ctrl Pts',(37.2323529907576,-0.33999812850501,-8.13739264459349));
#60880=CARTESIAN_POINT('Ctrl Pts',(37.2954118399697,-0.330502896895357,
-8.05203097106307));
#60881=CARTESIAN_POINT('Ctrl Pts',(37.3805242936423,-0.319026760440954,
-7.95146162160763));
#60882=CARTESIAN_POINT('Ctrl Pts',(37.3974598869159,-0.316802027590474,
-7.93208940090425));
#60883=CARTESIAN_POINT('Ctrl Pts',(37.4234620368301,-0.31347777291652,-7.90329207603053));
#60884=CARTESIAN_POINT('Ctrl Pts',(37.4322992181859,-0.312363354983257,
-7.89366383116365));
#60885=CARTESIAN_POINT('Ctrl Pts',(37.4486347512679,-0.31033201845608,-7.87615464087459));
#60886=CARTESIAN_POINT('Ctrl Pts',(37.4561084298851,-0.309413486556029,
-7.86825214501251));
#60887=CARTESIAN_POINT('Ctrl Pts',(37.4736824395626,-0.307278330162745,
-7.84992048601222));
#60888=CARTESIAN_POINT('Ctrl Pts',(37.4838239626568,-0.30606482531752,-7.83953165580069));
#60889=CARTESIAN_POINT('Ctrl Pts',(37.517871957053,-0.302049447567075,-7.80527935389552));
#60890=CARTESIAN_POINT('Ctrl Pts',(37.5421883520759,-0.299276382565353,
-7.78182624570433));
#60891=CARTESIAN_POINT('Ctrl Pts',(37.604144891096,-0.292416607127595,-7.72453900275184));
#60892=CARTESIAN_POINT('Ctrl Pts',(37.6423748838302,-0.288364930964759,
-7.69136478226724));
#60893=CARTESIAN_POINT('Ctrl Pts',(37.8324258291359,-0.268912148770531,
-7.53668458011679));
#60894=CARTESIAN_POINT('Ctrl Pts',(37.9975466935135,-0.25399723009004,-7.43268887387241));
#60895=CARTESIAN_POINT('Ctrl Pts',(38.2248916447087,-0.233846072046994,
-7.32539546500609));
#60896=CARTESIAN_POINT('Ctrl Pts',(38.2772383296457,-0.229235395443278,
-7.30292746624488));
#60897=CARTESIAN_POINT('Ctrl Pts',(38.3521120456911,-0.222647549127527,
-7.273892537794));
#60898=CARTESIAN_POINT('Ctrl Pts',(38.3740159980717,-0.220721217710182,
-7.26576359349363));
#60899=CARTESIAN_POINT('Ctrl Pts',(38.4144336636024,-0.217166047922567,
-7.25143020885292));
#60900=CARTESIAN_POINT('Ctrl Pts',(38.4329113786508,-0.2155404876216,-7.24512959491965));
#60901=CARTESIAN_POINT('Ctrl Pts',(38.4708711083746,-0.212199246849162,
-7.23269961397555));
#60902=CARTESIAN_POINT('Ctrl Pts',(38.4903585290173,-0.210483008232813,
-7.22659208842799));
#60903=CARTESIAN_POINT('Ctrl Pts',(38.5399795687589,-0.20610907898399,-7.21173163143301));
#60904=CARTESIAN_POINT('Ctrl Pts',(38.5702100891409,-0.203440751933646,
-7.20331914704168));
#60905=CARTESIAN_POINT('Ctrl Pts',(38.7141037477106,-0.190715810032737,
-7.16629377441332));
#60906=CARTESIAN_POINT('Ctrl Pts',(38.8295751616615,-0.180422588450311,
-7.14542717721622));
#60907=CARTESIAN_POINT('Ctrl Pts',(39.0970803739772,-0.156427354476174,
-7.11703077089765));
#60908=CARTESIAN_POINT('Ctrl Pts',(39.249247079007,-0.14265958054726,-7.11533550900872));
#60909=CARTESIAN_POINT('Ctrl Pts',(39.4487782514335,-0.124947326710104,
-7.13203034026109));
#60910=CARTESIAN_POINT('Ctrl Pts',(39.4968704293992,-0.120707318125235,
-7.13751947798899));
#60911=CARTESIAN_POINT('Ctrl Pts',(39.5615883129148,-0.115066374116952,
-7.14689241725424));
#60912=CARTESIAN_POINT('Ctrl Pts',(39.5783825476538,-0.11360851904779,-7.14950668664864));
#60913=CARTESIAN_POINT('Ctrl Pts',(39.6051482703157,-0.111296011342877,
-7.1539642359262));
#60914=CARTESIAN_POINT('Ctrl Pts',(39.6151378246616,-0.110435375569327,
-7.15569286195205));
#60915=CARTESIAN_POINT('Ctrl Pts',(39.6364936746104,-0.108601134750289,
-7.15952756702325));
#60916=CARTESIAN_POINT('Ctrl Pts',(39.6478563971483,-0.107628623607068,
-7.16165253841174));
#60917=CARTESIAN_POINT('Ctrl Pts',(39.6773554991746,-0.105111699880287,
-7.16738963757558));
#60918=CARTESIAN_POINT('Ctrl Pts',(39.6954668118991,-0.103574134305051,
-7.17112923115936));
#60919=CARTESIAN_POINT('Ctrl Pts',(39.7807839217993,-0.0963596716489415,
-7.18977377814061));
#60920=CARTESIAN_POINT('Ctrl Pts',(39.8473803774488,-0.0908119398858467,
-7.20735195952669));
#60921=CARTESIAN_POINT('Ctrl Pts',(40.089742885649,-0.0706168713194944,
-7.28258940027681));
#60922=CARTESIAN_POINT('Ctrl Pts',(40.2594373998762,-0.0564204594033885,
-7.35759490718814));
#60923=CARTESIAN_POINT('Ctrl Pts',(40.4781839297072,-0.0361935463108925,
-7.48616878476222));
#60924=CARTESIAN_POINT('Ctrl Pts',(40.535971204172,-0.0306493270394711,
-7.52355896645561));
#60925=CARTESIAN_POINT('Ctrl Pts',(40.6146472762807,-0.0227501733217693,
-7.57939153025153));
#60926=CARTESIAN_POINT('Ctrl Pts',(40.6369431528341,-0.0204700991323039,
-7.5957997819905));
#60927=CARTESIAN_POINT('Ctrl Pts',(40.674469987915,-0.0165570758753307,
-7.62442844014172));
#60928=CARTESIAN_POINT('Ctrl Pts',(40.6898447821298,-0.0149316442030096,
-7.63645651957838));
#60929=CARTESIAN_POINT('Ctrl Pts',(40.7210033522578,-0.0115903008130991,
-7.66144991700499));
#60930=CARTESIAN_POINT('Ctrl Pts',(40.7367717251884,-0.00987382761739585,
-7.67443178483092));
#60931=CARTESIAN_POINT('Ctrl Pts',(40.7763509682222,-0.00549852460097494,
-7.70787150371802));
#60932=CARTESIAN_POINT('Ctrl Pts',(40.7999294223589,-0.00282904475207008,
-7.72859692986818));
#60933=CARTESIAN_POINT('Ctrl Pts',(40.9097713077327,0.00991763226400466,
-7.82902584926393));
#60934=CARTESIAN_POINT('Ctrl Pts',(40.990512393684,0.0202324733536286,-7.9145023387958));
#60935=CARTESIAN_POINT('Ctrl Pts',(41.1611749597574,0.0443321356235607,
-8.12393604805064));
#60936=CARTESIAN_POINT('Ctrl Pts',(41.2461699790002,0.0581845503089543,
-8.25127477728285));
#60937=CARTESIAN_POINT('Ctrl Pts',(41.3409912235909,0.075887375701987,-8.42761140179743));
#60938=CARTESIAN_POINT('Ctrl Pts',(41.3622272930147,0.0800440322162215,
-8.47006913568574));
#60939=CARTESIAN_POINT('Ctrl Pts',(41.389295523635,0.0855937102356448,-8.52844444831731));
#60940=CARTESIAN_POINT('Ctrl Pts',(41.3962350805101,0.087041422994478,-8.54383264497544));
#60941=CARTESIAN_POINT('Ctrl Pts',(41.4074756941205,0.0894272976914303,
-8.56947522406712));
#60942=CARTESIAN_POINT('Ctrl Pts',(41.4118685649977,0.0903706465163295,
-8.57968840545864));
#60943=CARTESIAN_POINT('Ctrl Pts',(41.4208148339292,0.0923143529480128,
-8.60089182727806));
#60944=CARTESIAN_POINT('Ctrl Pts',(41.4253577904836,0.0933141033867259,
-8.61188600670741));
#60945=CARTESIAN_POINT('Ctrl Pts',(41.4373402732732,0.0959870570085815,
-8.64150487203092));
#60946=CARTESIAN_POINT('Ctrl Pts',(41.4446289781568,0.0976517695544874,
-8.66019021114716));
#60947=CARTESIAN_POINT('Ctrl Pts',(41.486120137049,0.107376546012066,-8.77061709439323));
#60948=CARTESIAN_POINT('Ctrl Pts',(41.5149340903055,0.115171272698597,-8.86429986033626));
#60949=CARTESIAN_POINT('Ctrl Pts',(41.5852992690839,0.138756574336345,-9.15520772328607));
#60950=CARTESIAN_POINT('Ctrl Pts',(41.6078737843295,0.154268658548737,-9.35607415626702));
#60951=CARTESIAN_POINT('Ctrl Pts',(41.6046596616596,0.173637730729523,-9.59467472712521));
#60952=CARTESIAN_POINT('Ctrl Pts',(41.6032910858076,0.176686573432366,-9.63193135170431));
#60953=CARTESIAN_POINT('Ctrl Pts',(41.5997490696134,0.181562940191475,-9.69093393179105));
#60954=CARTESIAN_POINT('Ctrl Pts',(41.5981440539688,0.183372951168642,-9.71270907902687));
#60955=CARTESIAN_POINT('Ctrl Pts',(41.5947335376811,0.186636444317341,-9.75172597356677));
#60956=CARTESIAN_POINT('Ctrl Pts',(41.593037622082,0.188086427460028,-9.76897600185936));
#60957=CARTESIAN_POINT('Ctrl Pts',(41.5886036386034,0.191516053599071,-9.80956601547673));
#60958=CARTESIAN_POINT('Ctrl Pts',(41.5857097125691,0.193500403577372,-9.83288673675066));
#60959=CARTESIAN_POINT('Ctrl Pts',(41.5760233404407,0.199473986966623,-9.90257361123265));
#60960=CARTESIAN_POINT('Ctrl Pts',(41.5682176100226,0.203493951617044,-9.94878466795191));
#60961=CARTESIAN_POINT('Ctrl Pts',(41.5467265996124,0.213029429211386,-10.0567152127004));
#60962=CARTESIAN_POINT('Ctrl Pts',(41.5319485023178,0.218574214077954,-10.1181792385115));
#60963=CARTESIAN_POINT('Ctrl Pts',(41.4876280889811,0.233017307224677,-10.2750505902207));
#60964=CARTESIAN_POINT('Ctrl Pts',(41.4545347448964,0.241985899040003,-10.3693273678396));
#60965=CARTESIAN_POINT('Ctrl Pts',(41.3691192749965,0.261705276006662,-10.5714633515747));
#60966=CARTESIAN_POINT('Ctrl Pts',(41.3143933968707,0.27243248852972,-10.6780445073195));
#60967=CARTESIAN_POINT('Ctrl Pts',(41.2411710375347,0.284593398051113,-10.797753290145));
#60968=CARTESIAN_POINT('Ctrl Pts',(41.2301587551715,0.28637319423434,-10.8152463558918));
#60969=CARTESIAN_POINT('Ctrl Pts',(41.2123838781288,0.289167327081202,-10.8426906748621));
#60970=CARTESIAN_POINT('Ctrl Pts',(41.2057701304724,0.290190487643724,-10.8527363408446));
#60971=CARTESIAN_POINT('Ctrl Pts',(41.1928658067752,0.292154745363263,-10.8720203106328));
#60972=CARTESIAN_POINT('Ctrl Pts',(41.1865857964016,0.293096413512395,-10.8812649900538));
#60973=CARTESIAN_POINT('Ctrl Pts',(41.1708198874341,0.295426242104155,-10.9041292074058));
#60974=CARTESIAN_POINT('Ctrl Pts',(41.1612567654965,0.296809408614601,-10.9176953532194));
#60975=CARTESIAN_POINT('Ctrl Pts',(41.1230613070618,0.30222214882506,-10.9707052361892));
#60976=CARTESIAN_POINT('Ctrl Pts',(41.0933709212187,0.306188584640413,-11.0093772795345));
#60977=CARTESIAN_POINT('Ctrl Pts',(40.9149465872621,0.328864566832165,-11.2277033991101));
#60978=CARTESIAN_POINT('Ctrl Pts',(40.7418904270486,0.346557674353927,-11.3858685475675));
#60979=CARTESIAN_POINT('Ctrl Pts',(40.5050211573478,0.369555531288926,-11.5462776182279));
#60980=CARTESIAN_POINT('Ctrl Pts',(40.4603214599847,0.37384323098138,-11.5744468652348));
#60981=CARTESIAN_POINT('Ctrl Pts',(40.3935398772801,0.380201068956179,-11.6135206399911));
#60982=CARTESIAN_POINT('Ctrl Pts',(40.372158094503,0.382229664439735,-11.6255954424682));
#60983=CARTESIAN_POINT('Ctrl Pts',(40.333675384848,0.385870823140411,-11.6465570510323));
#60984=CARTESIAN_POINT('Ctrl Pts',(40.3166451726377,0.387478800552697,-11.6555698091852));
#60985=CARTESIAN_POINT('Ctrl Pts',(40.2801360714548,0.390919999374295,-11.6743332584336));
#60986=CARTESIAN_POINT('Ctrl Pts',(40.2606294615052,0.39275506398798,-11.6840258143623));
#60987=CARTESIAN_POINT('Ctrl Pts',(40.2067160574572,0.397819051268324,-11.7099076725914));
#60988=CARTESIAN_POINT('Ctrl Pts',(40.1720543541811,0.401066183175113,-11.7255473722306));
#60989=CARTESIAN_POINT('Ctrl Pts',(40.0218683204445,0.415108976259383,-11.7890721410653));
#60990=CARTESIAN_POINT('Ctrl Pts',(39.9030946461116,0.426162127174695,-11.8287226728999));
#60991=CARTESIAN_POINT('Ctrl Pts',(39.6430213372514,0.4501628036776,-11.8935524061029));
#60992=CARTESIAN_POINT('Ctrl Pts',(39.5014329263022,0.463111148670782,-11.9157006862557));
#60993=CARTESIAN_POINT('Ctrl Pts',(39.3194317485095,0.479167022081036,-11.9277356497144));
#60994=CARTESIAN_POINT('Ctrl Pts',(39.2800913958472,0.482601360258549,-11.9293686125491));
#60995=CARTESIAN_POINT('Ctrl Pts',(39.2249594707982,0.487349163607097,-11.9303021869398));
#60996=CARTESIAN_POINT('Ctrl Pts',(39.2091904619028,0.488699681721397,-11.9304141353327));
#60997=CARTESIAN_POINT('Ctrl Pts',(39.1823878354658,0.490981278396629,-11.9303408249749));
#60998=CARTESIAN_POINT('Ctrl Pts',(39.1713547688906,0.491916455400143,-11.9302347383789));
#60999=CARTESIAN_POINT('Ctrl Pts',(39.1479670375202,0.493889945139972,-11.9298488945948));
#61000=CARTESIAN_POINT('Ctrl Pts',(39.1356132440575,0.494927221829795,-11.9295498542697));
#61001=CARTESIAN_POINT('Ctrl Pts',(39.1010458726237,0.497816634971966,-11.928446500116));
#61002=CARTESIAN_POINT('Ctrl Pts',(39.0788395460799,0.499657773728774,-11.9274294475609));
#61003=CARTESIAN_POINT('Ctrl Pts',(39.0281202733096,0.503835276764671,-11.9244014067842));
#61004=CARTESIAN_POINT('Ctrl Pts',(38.9996222175465,0.506162513253759,-11.9221897467921));
#61005=CARTESIAN_POINT('Ctrl Pts',(38.9027021559795,0.514030219286462,-11.9129274327818));
#61006=CARTESIAN_POINT('Ctrl Pts',(38.8345418315237,0.51948362721814,-11.9034501952042));
#61007=CARTESIAN_POINT('Ctrl Pts',(38.5965967997216,0.538531406987109,-11.8598927667114));
#61008=CARTESIAN_POINT('Ctrl Pts',(38.430191248427,0.551908901786091,-11.810434407625));
#61009=CARTESIAN_POINT('Ctrl Pts',(38.221578067747,0.57008933036705,-11.7230357771963));
#61010=CARTESIAN_POINT('Ctrl Pts',(38.1733143215142,0.574397474585507,-11.7009104915031));
#61011=CARTESIAN_POINT('Ctrl Pts',(38.1038153656843,0.580779744308204,-11.6662233178907));
#61012=CARTESIAN_POINT('Ctrl Pts',(38.0819762340619,0.582811853122353,-11.6549015979669));
#61013=CARTESIAN_POINT('Ctrl Pts',(38.0433436712948,0.586456862575836,-11.6341160474144));
#61014=CARTESIAN_POINT('Ctrl Pts',(38.0264828563667,0.588065139428848,-11.6247813772293));
#61015=CARTESIAN_POINT('Ctrl Pts',(37.9908315759203,0.591504347642001,-11.6044802122961));
#61016=CARTESIAN_POINT('Ctrl Pts',(37.9720742208278,0.593337096927028,-11.5934594376596));
#61017=CARTESIAN_POINT('Ctrl Pts',(37.9210618495814,0.59838751319231,-11.5625490249103));
#61018=CARTESIAN_POINT('Ctrl Pts',(37.8891247562829,0.60162322527827,-11.5421501102595));
#61019=CARTESIAN_POINT('Ctrl Pts',(37.7547637053739,0.615565577340072,-11.4517922430212));
#61020=CARTESIAN_POINT('Ctrl Pts',(37.6573679612897,0.626525287533903,-11.3747332061649));
#61021=CARTESIAN_POINT('Ctrl Pts',(37.4629229628616,0.650242182224442,-11.1948132043292));
#61022=CARTESIAN_POINT('Ctrl Pts',(37.3680944350712,0.66299928217291,-11.0901956551537));
#61023=CARTESIAN_POINT('Ctrl Pts',(37.2577079335957,0.679110347746528,-10.9445434203887));
#61024=CARTESIAN_POINT('Ctrl Pts',(37.2333185744732,0.682763709147642,-10.9105564821617));
#61025=CARTESIAN_POINT('Ctrl Pts',(37.2007516761759,0.687759552711926,-10.8625799532121));
#61026=CARTESIAN_POINT('Ctrl Pts',(37.1918118811615,0.689144059206279,-10.8491202797258));
#61027=CARTESIAN_POINT('Ctrl Pts',(37.17702136369,0.691455775454915,-10.8263574110851));
#61028=CARTESIAN_POINT('Ctrl Pts',(37.171097670997,0.692387515470001,-10.8171025642644));
#61029=CARTESIAN_POINT('Ctrl Pts',(37.1587568771471,0.694340720973326,-10.7975278438001));
#61030=CARTESIAN_POINT('Ctrl Pts',(37.1523542336184,0.69536128154118,-10.7871994435548));
#61031=CARTESIAN_POINT('Ctrl Pts',(37.1349689942243,0.698153793312059,-10.7586740270223));
#61032=CARTESIAN_POINT('Ctrl Pts',(37.1241485069163,0.699915902906804,-10.7403786790968));
#61033=CARTESIAN_POINT('Ctrl Pts',(37.1001631665927,0.703883551118638,-10.6985690279299));
#61034=CARTESIAN_POINT('Ctrl Pts',(37.0871478758857,0.706081234605045,-10.6749717612468));
#61035=CARTESIAN_POINT('Ctrl Pts',(36.9856066340711,0.723639599210348,-10.483326841681));
#61036=CARTESIAN_POINT('Ctrl Pts',(36.9168640608305,0.738199076413479,-10.3055353225338));
#61037=CARTESIAN_POINT('Ctrl Pts',(36.8463076368886,0.760677509060627,-10.0298996586911));
#61038=CARTESIAN_POINT('Ctrl Pts',(36.8282856007341,0.768228739507843,-9.93701768949147));
#61039=CARTESIAN_POINT('Ctrl Pts',(36.8117639586395,0.778424370763315,-9.81327213209202));
#61040=CARTESIAN_POINT('Ctrl Pts',(36.8083202880956,0.780916403195077,-9.78314763349859));
#61041=CARTESIAN_POINT('Ctrl Pts',(36.803722874488,0.784931877966725,-9.7348567409574));
#61042=CARTESIAN_POINT('Ctrl Pts',(36.8022042626951,0.78644397149213,-9.71672761464688));
#61043=CARTESIAN_POINT('Ctrl Pts',(36.7995672211515,0.78949419751867,-9.68028090056927));
#61044=CARTESIAN_POINT('Ctrl Pts',(36.7984524928712,0.791032339025779,-9.66196428390763));
#61045=CARTESIAN_POINT('Ctrl Pts',(36.7965860796382,0.794217919156763,-9.62416865368595));
#61046=CARTESIAN_POINT('Ctrl Pts',(36.7958614032487,0.795866078219987,-9.60468973575619));
#61047=CARTESIAN_POINT('Ctrl Pts',(36.7948625149559,0.79925576469566,-9.56479334059602));
#61048=CARTESIAN_POINT('Ctrl Pts',(36.7946114035323,0.800997857916507,-9.54437702317166));
#61049=CARTESIAN_POINT('Ctrl Pts',(36.794620224509,0.802747783846628,-9.52396074128696));
#61050=CARTESIAN_POINT('Ctrl Pts',(36.9547201749638,0.879636998740377,-8.65231241759342));
#61051=CARTESIAN_POINT('Ctrl Pts',(36.8488865264236,0.85468339172866,-8.92847699586774));
#61052=CARTESIAN_POINT('Ctrl Pts',(36.797182863997,0.829729784716943,-9.22613963971494));
#61053=CARTESIAN_POINT('Ctrl Pts',(36.7981523919191,0.804776177705222,-9.52412467452362));
#61054=CARTESIAN_POINT('Ctrl Pts',(36.9580194911167,1.14613690893122,-8.65357797698964));
#61055=CARTESIAN_POINT('Ctrl Pts',(36.931497086075,1.13961745573623,-8.72181439239125));
#61056=CARTESIAN_POINT('Ctrl Pts',(36.9080875735724,1.13303884220261,-8.79126758483645));
#61057=CARTESIAN_POINT('Ctrl Pts',(36.8537945688819,1.11534357173267,-8.98052894869805));
#61058=CARTESIAN_POINT('Ctrl Pts',(36.8289170938238,1.10424056888671,-9.10179610595467));
#61059=CARTESIAN_POINT('Ctrl Pts',(36.8106549506259,1.09154891176514,-9.2468077204081));
#61060=CARTESIAN_POINT('Ctrl Pts',(36.8081535430804,1.08960531823904,-9.26920448033023));
#61061=CARTESIAN_POINT('Ctrl Pts',(36.8047622553276,1.08661506383349,-9.30399474367018));
#61062=CARTESIAN_POINT('Ctrl Pts',(36.8036530847002,1.08555749068718,-9.3163647688518));
#61063=CARTESIAN_POINT('Ctrl Pts',(36.8017415028711,1.08357241212548,-9.33971556002907));
#61064=CARTESIAN_POINT('Ctrl Pts',(36.8009186294136,1.08264394199766,-9.3506935807053));
#61065=CARTESIAN_POINT('Ctrl Pts',(36.7991103191695,1.08040760889664,-9.37726454413118));
#61066=CARTESIAN_POINT('Ctrl Pts',(36.7982013707649,1.07910387186094,-9.39286215799357));
#61067=CARTESIAN_POINT('Ctrl Pts',(36.7955819084487,1.07461743869307,-9.44686803163611));
#61068=CARTESIAN_POINT('Ctrl Pts',(36.7946401158394,1.07147232060647,-9.48531022708832));
#61069=CARTESIAN_POINT('Ctrl Pts',(36.7945880042618,1.06327879496806,-9.5865254092814));
#61070=CARTESIAN_POINT('Ctrl Pts',(36.7970122625023,1.05828745084736,-9.64927173968473));
#61071=CARTESIAN_POINT('Ctrl Pts',(36.8182794592562,1.03668275355598,-9.9222148897046));
#61072=CARTESIAN_POINT('Ctrl Pts',(36.8622730995552,1.02046588534418,-10.1294824763955));
#61073=CARTESIAN_POINT('Ctrl Pts',(36.944649832248,1.00041379659953,-10.3619712761099));
#61074=CARTESIAN_POINT('Ctrl Pts',(36.9573086736758,0.997492653788696,-10.3953221510601));
#61075=CARTESIAN_POINT('Ctrl Pts',(36.9787022358353,0.992788718018505,-10.4481157897272));
#61076=CARTESIAN_POINT('Ctrl Pts',(36.9869622719098,0.99102167626982,-10.4677462394215));
#61077=CARTESIAN_POINT('Ctrl Pts',(37.0032280064555,0.987631200569094,-10.5050105651657));
#61078=CARTESIAN_POINT('Ctrl Pts',(37.011188175541,0.98600941231694,-10.5226625932093));
#61079=CARTESIAN_POINT('Ctrl Pts',(37.0300934318465,0.982240755306312,-10.563270256354));
#61080=CARTESIAN_POINT('Ctrl Pts',(37.0411909849412,0.980088835354502,-10.5861518126627));
#61081=CARTESIAN_POINT('Ctrl Pts',(37.078878893681,0.972969568630612,-10.6608199056665));
#61082=CARTESIAN_POINT('Ctrl Pts',(37.1069842886146,0.967951156116989,-10.7118132157487));
#61083=CARTESIAN_POINT('Ctrl Pts',(37.1814726844309,0.955313878702441,-10.8360731726929));
#61084=CARTESIAN_POINT('Ctrl Pts',(37.2300172231052,0.9476310280052,-10.9079425935613));
#61085=CARTESIAN_POINT('Ctrl Pts',(37.3620071422727,0.928074053871764,-11.0822595598534));
#61086=CARTESIAN_POINT('Ctrl Pts',(37.4502121535132,0.916132655189497,-11.1807531457853));
#61087=CARTESIAN_POINT('Ctrl Pts',(37.5846427592641,0.899718576544822,-11.3080587770194));
#61088=CARTESIAN_POINT('Ctrl Pts',(37.6244371430778,0.895051909162368,-11.3433180219806));
#61089=CARTESIAN_POINT('Ctrl Pts',(37.6788849975739,0.888947786310866,-11.3884296576259));
#61090=CARTESIAN_POINT('Ctrl Pts',(37.6925217464467,0.887441386799851,-11.399478676957));
#61091=CARTESIAN_POINT('Ctrl Pts',(37.7143020319535,0.885072099187608,-11.4167344606176));
#61092=CARTESIAN_POINT('Ctrl Pts',(37.7223659751232,0.884202708591631,-11.42303988959));
#61093=CARTESIAN_POINT('Ctrl Pts',(37.7395108808127,0.882371148720978,-11.4362704899073));
#61094=CARTESIAN_POINT('Ctrl Pts',(37.748601407989,0.881409921539475,-11.4431828624648));
#61095=CARTESIAN_POINT('Ctrl Pts',(37.7720198548643,0.878957876791219,-11.4607282809352));
#61096=CARTESIAN_POINT('Ctrl Pts',(37.7864178834406,0.877473255002006,-11.4712674355299));
#61097=CARTESIAN_POINT('Ctrl Pts',(37.8504876459113,0.870960520825029,-11.517079466595));
#61098=CARTESIAN_POINT('Ctrl Pts',(37.9013767640468,0.866032843728939,-11.5506217745362));
#61099=CARTESIAN_POINT('Ctrl Pts',(38.0699645791256,0.850287557906748,-11.6527734637443));
#61100=CARTESIAN_POINT('Ctrl Pts',(38.1922289829027,0.83973084262256,-11.7133332450156));
#61101=CARTESIAN_POINT('Ctrl Pts',(38.4282320924356,0.819797415686219,-11.806231135488));
#61102=CARTESIAN_POINT('Ctrl Pts',(38.5404832272685,0.810487041138136,-11.8411763419449));
#61103=CARTESIAN_POINT('Ctrl Pts',(38.6858968992707,0.798311590755273,-11.875014599526));
#61104=CARTESIAN_POINT('Ctrl Pts',(38.7171069230509,0.795692590205841,-11.8816257021449));
#61105=CARTESIAN_POINT('Ctrl Pts',(38.7685971577293,0.791356630002007,-11.89146694032));
#61106=CARTESIAN_POINT('Ctrl Pts',(38.7888043833915,0.789651208671667,-11.8950616663796));
#61107=CARTESIAN_POINT('Ctrl Pts',(38.8284688122384,0.78629480625426,-11.9015951829009));
#61108=CARTESIAN_POINT('Ctrl Pts',(38.8479210047945,0.784644614771989,-11.9045546681911));
#61109=CARTESIAN_POINT('Ctrl Pts',(38.894612694088,0.78067238914831,-11.9110733706935));
#61110=CARTESIAN_POINT('Ctrl Pts',(38.9218804886875,0.778343491570431,-11.9144051435304));
#61111=CARTESIAN_POINT('Ctrl Pts',(39.0215358530242,0.769794833078296,-11.924852859251));
#61112=CARTESIAN_POINT('Ctrl Pts',(39.0941715674575,0.763490941589336,-11.9291508291074));
#61113=CARTESIAN_POINT('Ctrl Pts',(39.2874950089218,0.746504737494365,-11.9318127549201));
#61114=CARTESIAN_POINT('Ctrl Pts',(39.4080491253668,0.735688967729816,-11.9243983943415));
#61115=CARTESIAN_POINT('Ctrl Pts',(39.6433356995204,0.714344709284184,-11.8920597535195));
#61116=CARTESIAN_POINT('Ctrl Pts',(39.7578444580982,0.703846678325236,-11.8677193155008));
#61117=CARTESIAN_POINT('Ctrl Pts',(39.8948022764581,0.691425745187621,-11.827989836002));
#61118=CARTESIAN_POINT('Ctrl Pts',(39.9193505607167,0.689205273583825,-11.8204405502506));
#61119=CARTESIAN_POINT('Ctrl Pts',(39.9561917559453,0.685886206390024,-11.8084617265558));
#61120=CARTESIAN_POINT('Ctrl Pts',(39.9685761930975,0.684772777451614,-11.8043231645117));
#61121=CARTESIAN_POINT('Ctrl Pts',(39.991212882229,0.682742581488666,-11.7965530788199));
#61122=CARTESIAN_POINT('Ctrl Pts',(40.0014746956405,0.681824209814641,-11.7929527194456));
#61123=CARTESIAN_POINT('Ctrl Pts',(40.0253850803141,0.679688613981469,-11.7843811937629));
#61124=CARTESIAN_POINT('Ctrl Pts',(40.0390135735113,0.678474517842431,-11.7793558205919));
#61125=CARTESIAN_POINT('Ctrl Pts',(40.0842337468289,0.67445387157678,-11.7622144246559));
#61126=CARTESIAN_POINT('Ctrl Pts',(40.1156171058574,0.671676237836499,-11.7495546435479));
#61127=CARTESIAN_POINT('Ctrl Pts',(40.1933565295819,0.664801978521204,-11.7162710525721));
#61128=CARTESIAN_POINT('Ctrl Pts',(40.2393482880734,0.660740582615042,-11.6948345430988));
#61129=CARTESIAN_POINT('Ctrl Pts',(40.4470362875822,0.642269918515834,-11.5899117401693));
#61130=CARTESIAN_POINT('Ctrl Pts',(40.5996065638879,0.628285018782427,-11.4897046267061));
#61131=CARTESIAN_POINT('Ctrl Pts',(40.7900920616115,0.608497383711214,-11.3310478186682));
#61132=CARTESIAN_POINT('Ctrl Pts',(40.839000286265,0.603177589844435,-11.2867826504993));
#61133=CARTESIAN_POINT('Ctrl Pts',(40.9054510360189,0.595545403892491,-11.2214762248616));
#61134=CARTESIAN_POINT('Ctrl Pts',(40.9245507798935,0.593301084920462,-11.2020567381452));
#61135=CARTESIAN_POINT('Ctrl Pts',(40.9567115186256,0.5894303392864,-11.168227183308));
#61136=CARTESIAN_POINT('Ctrl Pts',(40.969935390187,0.587811022602961,-11.1539750162615));
#61137=CARTESIAN_POINT('Ctrl Pts',(40.9967765133129,0.584465175529347,-11.1243340146422));
#61138=CARTESIAN_POINT('Ctrl Pts',(41.0103721882208,0.582737928504908,-11.1089279065688));
#61139=CARTESIAN_POINT('Ctrl Pts',(41.0446417329438,0.578298383789974,-11.0690772919074));
#61140=CARTESIAN_POINT('Ctrl Pts',(41.0650272926808,0.575574788170089,-11.044391586039));
#61141=CARTESIAN_POINT('Ctrl Pts',(41.1660983478821,0.56163317071988,-10.9169010003618));
#61142=CARTESIAN_POINT('Ctrl Pts',(41.2387876780221,0.550116091301752,-10.8080682098474));
#61143=CARTESIAN_POINT('Ctrl Pts',(41.3671108956774,0.526493088775805,-10.5772768944705));
#61144=CARTESIAN_POINT('Ctrl Pts',(41.4221355103943,0.514420389180119,-10.4554682798378));
#61145=CARTESIAN_POINT('Ctrl Pts',(41.4839277549893,0.498059328967464,-10.2814095348409));
#61146=CARTESIAN_POINT('Ctrl Pts',(41.4995323106832,0.493561301659272,-10.232554629738));
#61147=CARTESIAN_POINT('Ctrl Pts',(41.5183088518674,0.487639593660438,-10.1665587078539));
#61148=CARTESIAN_POINT('Ctrl Pts',(41.5228728702454,0.486151842494649,-10.149832130141));
#61149=CARTESIAN_POINT('Ctrl Pts',(41.5298335486495,0.483804465048132,-10.1231910728997));
#61150=CARTESIAN_POINT('Ctrl Pts',(41.5323485765599,0.482938537249089,-10.1133086380542));
#61151=CARTESIAN_POINT('Ctrl Pts',(41.5375585471286,0.481106435461196,-10.0922781605082));
#61152=CARTESIAN_POINT('Ctrl Pts',(41.5402367708715,0.480141259110742,-10.0811261945271));
#61153=CARTESIAN_POINT('Ctrl Pts',(41.5469302725944,0.477666016140122,-10.0523499350229));
#61154=CARTESIAN_POINT('Ctrl Pts',(41.5508269567604,0.476162377851029,-10.0346982815993));
#61155=CARTESIAN_POINT('Ctrl Pts',(41.567536756906,0.469409647644259,-9.95473212708788));
#61156=CARTESIAN_POINT('Ctrl Pts',(41.5780750841111,0.464270379605273,-9.8919615525581));
#61157=CARTESIAN_POINT('Ctrl Pts',(41.6050938043786,0.447207772394857,-9.6797784097128));
#61158=CARTESIAN_POINT('Ctrl Pts',(41.6100663027085,0.435596808906464,-9.5292592531869));
#61159=CARTESIAN_POINT('Ctrl Pts',(41.5947911571082,0.415720391052272,-9.2776243602733));
#61160=CARTESIAN_POINT('Ctrl Pts',(41.5821764409379,0.407608865056097,-9.17650255170654));
#61161=CARTESIAN_POINT('Ctrl Pts',(41.5573949042475,0.396762706005806,-9.04592787262659));
#61162=CARTESIAN_POINT('Ctrl Pts',(41.5510017888084,0.394207114800862,-9.01547939421215));
#61163=CARTESIAN_POINT('Ctrl Pts',(41.5394497731286,0.389948026440219,-8.96531934443248));
#61164=CARTESIAN_POINT('Ctrl Pts',(41.5346275994517,0.388255246085189,-8.94553335221888));
#61165=CARTESIAN_POINT('Ctrl Pts',(41.5246284642194,0.384902662719987,-8.90665820935601));
#61166=CARTESIAN_POINT('Ctrl Pts',(41.5194661256437,0.38324344755222,-8.88756693776711));
#61167=CARTESIAN_POINT('Ctrl Pts',(41.5064155079617,0.379212868604969,-8.84156241715001));
#61168=CARTESIAN_POINT('Ctrl Pts',(41.4982909982984,0.376834113934977,-8.81471993612044));
#61169=CARTESIAN_POINT('Ctrl Pts',(41.4659547714421,0.367824455153892,-8.7142546247587));
#61170=CARTESIAN_POINT('Ctrl Pts',(41.4386617536935,0.361096822711199,-8.64168247565026));
#61171=CARTESIAN_POINT('Ctrl Pts',(41.3513717925894,0.341729295698674,-8.43975316925643));
#61172=CARTESIAN_POINT('Ctrl Pts',(41.2833176047823,0.328885492880572,-8.31423943031549));
#61173=CARTESIAN_POINT('Ctrl Pts',(41.1503174577058,0.307297902265517,-8.11370695861565));
#61174=CARTESIAN_POINT('Ctrl Pts',(41.0911058448527,0.298547611843039,-8.03529875912544));
#61175=CARTESIAN_POINT('Ctrl Pts',(41.0140577857044,0.288284610935066,-7.94529766504272));
#61176=CARTESIAN_POINT('Ctrl Pts',(41.0006594516044,0.286536993946662,-7.93004208831295));
#61177=CARTESIAN_POINT('Ctrl Pts',(40.9790724930371,0.283781694225559,-7.90608161793796));
#61178=CARTESIAN_POINT('Ctrl Pts',(40.9710098137012,0.282765576183815,-7.89726540179209));
#61179=CARTESIAN_POINT('Ctrl Pts',(40.955250996482,0.280805100121044,-7.88028948614087));
#61180=CARTESIAN_POINT('Ctrl Pts',(40.9475629732705,0.279860258803079,-7.87212299345442));
#61181=CARTESIAN_POINT('Ctrl Pts',(40.9282028452735,0.27750881054963,-7.85184405988391));
#61182=CARTESIAN_POINT('Ctrl Pts',(40.9164599475162,0.276107409992372,-7.83979936731374));
#61183=CARTESIAN_POINT('Ctrl Pts',(40.8688081342409,0.270514288907428,-7.79193782578148));
#61184=CARTESIAN_POINT('Ctrl Pts',(40.8318937219044,0.26639119406009,-7.75713433582304));
#61185=CARTESIAN_POINT('Ctrl Pts',(40.6356944470844,0.245348286152978,-7.58354222953039));
#61186=CARTESIAN_POINT('Ctrl Pts',(40.4597301492004,0.229241347136703,-7.46500715640543));
#61187=CARTESIAN_POINT('Ctrl Pts',(40.2119203975778,0.207147685941844,-7.34184771826776));
#61188=CARTESIAN_POINT('Ctrl Pts',(40.1521497673295,0.201866458749272,-7.31512530147421));
#61189=CARTESIAN_POINT('Ctrl Pts',(40.0661634733594,0.194281990729688,-7.28081858676874));
#61190=CARTESIAN_POINT('Ctrl Pts',(40.0407909482435,0.192045716922526,-7.27118992851656));
#61191=CARTESIAN_POINT('Ctrl Pts',(39.9968036298373,0.188168282405154,-7.25534323093124));
#61192=CARTESIAN_POINT('Ctrl Pts',(39.9782652062557,0.186533998757501,-7.24891979606678));
#61193=CARTESIAN_POINT('Ctrl Pts',(39.9400801356731,0.183166165369478,-7.23620997399349));
#61194=CARTESIAN_POINT('Ctrl Pts',(39.9204271161451,0.18143197211041,-7.22994812609138));
#61195=CARTESIAN_POINT('Ctrl Pts',(39.8696992266563,0.176952038417327,-7.21450095748407));
#61196=CARTESIAN_POINT('Ctrl Pts',(39.8385159451596,0.174194589989077,-7.20568974745903));
#61197=CARTESIAN_POINT('Ctrl Pts',(39.6692608333936,0.159200137456038,-7.16153661189935));
#61198=CARTESIAN_POINT('Ctrl Pts',(39.5284590780057,0.146602489050096,-7.13789619750786));
#61199=CARTESIAN_POINT('Ctrl Pts',(39.2316565917541,0.119918833242445,-7.11482422195453));
#61200=CARTESIAN_POINT('Ctrl Pts',(39.0760825424865,0.105859956512213,-7.11780230178375));
#61201=CARTESIAN_POINT('Ctrl Pts',(38.8952221482782,0.0899841896783604,
-7.13885599581126));
#61202=CARTESIAN_POINT('Ctrl Pts',(38.8686250107536,0.087662376952385,-7.14240403222418));
#61203=CARTESIAN_POINT('Ctrl Pts',(38.8289587467098,0.0842239900019295,
-7.14837262108122));
#61204=CARTESIAN_POINT('Ctrl Pts',(38.8158424248945,0.0830910239869222,
-7.15045745605491));
#61205=CARTESIAN_POINT('Ctrl Pts',(38.7931119884368,0.0811352851711953,
-7.15426373059113));
#61206=CARTESIAN_POINT('Ctrl Pts',(38.7834904289672,0.080309892642764,-7.15593518445652));
#61207=CARTESIAN_POINT('Ctrl Pts',(38.7604869363426,0.078342252599258,-7.16007582335779));
#61208=CARTESIAN_POINT('Ctrl Pts',(38.747115371639,0.0772030533942414,-7.16260002641951));
#61209=CARTESIAN_POINT('Ctrl Pts',(38.7057430978238,0.0736903687322396,
-7.17077423232197));
#61210=CARTESIAN_POINT('Ctrl Pts',(38.6778197155968,0.0713367144824334,
-7.1768098846533));
#61211=CARTESIAN_POINT('Ctrl Pts',(38.6110495141226,0.0657350235790357,
-7.19249237627467));
#61212=CARTESIAN_POINT('Ctrl Pts',(38.5723220729515,0.0625075765481499,
-7.20261429749493));
#61213=CARTESIAN_POINT('Ctrl Pts',(38.4118897982779,0.0491577277687317,
-7.24885228531607));
#61214=CARTESIAN_POINT('Ctrl Pts',(38.2928827228701,0.0392953291842206,
-7.29360830832483));
#61215=CARTESIAN_POINT('Ctrl Pts',(38.0620097516238,0.0192826051881944,
-7.40197459379847));
#61216=CARTESIAN_POINT('Ctrl Pts',(37.9506102434301,0.00916016733974761,
-7.46556396654334));
#61217=CARTESIAN_POINT('Ctrl Pts',(37.8180708158714,-0.00391720617964832,
-7.55594635420535));
#61218=CARTESIAN_POINT('Ctrl Pts',(37.7917022806951,-0.00657355479567719,
-7.57471851691715));
#61219=CARTESIAN_POINT('Ctrl Pts',(37.74916931706,-0.0109548781684845,-7.60631075595678));
#61220=CARTESIAN_POINT('Ctrl Pts',(37.732776213449,-0.0126678208351297,
-7.61881732490205));
#61221=CARTESIAN_POINT('Ctrl Pts',(37.7021860981284,-0.0159118838279119,
-7.64278341897208));
#61222=CARTESIAN_POINT('Ctrl Pts',(37.6879546520026,-0.0174411100794713,
-7.65419681178444));
#61223=CARTESIAN_POINT('Ctrl Pts',(37.6721906704758,-0.0191580517055498,
-7.66713664863116));
#61224=CARTESIAN_POINT('Ctrl Pts',(37.6705283701373,-0.0193393915737116,
-7.66850488470314));
#61225=CARTESIAN_POINT('Ctrl Pts',(37.6674937781192,-0.0196709654131965,
-7.67100949332569));
#61226=CARTESIAN_POINT('Ctrl Pts',(37.6661209059832,-0.0198211711323544,
-7.67214516385033));
#61227=CARTESIAN_POINT('Ctrl Pts',(37.6635148027179,-0.0201066840401274,
-7.67430587224538));
#61228=CARTESIAN_POINT('Ctrl Pts',(37.6622813316036,-0.0202419795431571,
-7.67533062067546));
#61229=CARTESIAN_POINT('Ctrl Pts',(37.6598686792253,-0.0205069335144982,
-7.67733909567683));
#61230=CARTESIAN_POINT('Ctrl Pts',(37.6586894131674,-0.0206365878128918,
-7.67832271972343));
#61231=CARTESIAN_POINT('Ctrl Pts',(37.6563243952665,-0.0208969092564838,
-7.68029922112771));
#61232=CARTESIAN_POINT('Ctrl Pts',(37.6551386574814,-0.0210275769871849,
-7.68129211408394));
#61233=CARTESIAN_POINT('Ctrl Pts',(37.6375881172503,-0.0229638888616028,
-7.69601710492904));
#61234=CARTESIAN_POINT('Ctrl Pts',(37.6214065876006,-0.0247781902902664,
-7.70996498740579));
#61235=CARTESIAN_POINT('Ctrl Pts',(37.5818338529958,-0.0292890038655323,
-7.74500472350681));
#61236=CARTESIAN_POINT('Ctrl Pts',(37.5586677400258,-0.0319953373275242,
-7.76634338810736));
#61237=CARTESIAN_POINT('Ctrl Pts',(37.4684631894485,-0.0428021174569438,
-7.85276713110247));
#61238=CARTESIAN_POINT('Ctrl Pts',(37.4048302304242,-0.0510375769064575,
-7.92127191653282));
#61239=CARTESIAN_POINT('Ctrl Pts',(37.249159825575,-0.0728423739289821,
-8.1097639877308));
#61240=CARTESIAN_POINT('Ctrl Pts',(37.1641577386255,-0.086537618455635,
-8.23503236025419));
#61241=CARTESIAN_POINT('Ctrl Pts',(37.0677904145058,-0.104258679145249,
-8.41056944947567));
#61242=CARTESIAN_POINT('Ctrl Pts',(37.0454418929366,-0.108570958311494,
-8.45441443371193));
#61243=CARTESIAN_POINT('Ctrl Pts',(37.017161210074,-0.11429063109198,-8.51437648914323));
#61244=CARTESIAN_POINT('Ctrl Pts',(37.0100349983504,-0.115756911868296,
-8.52991286469083));
#61245=CARTESIAN_POINT('Ctrl Pts',(36.9989403949401,-0.11807912908377,-8.55479762854446));
#61246=CARTESIAN_POINT('Ctrl Pts',(36.9948647301536,-0.118941137877828,
-8.56409704952668));
#61247=CARTESIAN_POINT('Ctrl Pts',(36.9862867939414,-0.120774321060462,
-8.58401130839614));
#61248=CARTESIAN_POINT('Ctrl Pts',(36.9818016782924,-0.121744432152582,
-8.59463335223591));
#61249=CARTESIAN_POINT('Ctrl Pts',(36.9707615799654,-0.124162937434917,
-8.62131321394616));
#61250=CARTESIAN_POINT('Ctrl Pts',(36.9643034256454,-0.125605804264154,
-8.63741078235361));
#61251=CARTESIAN_POINT('Ctrl Pts',(36.958019684865,-0.127039975641411,-8.65357747851736));
#61252=CARTESIAN_POINT('Origin',(39.2,8.05522481984854,-9.525));
#61253=CARTESIAN_POINT('',(36.9580197773588,-1.66076081124402,-8.65357724055094));
#61254=CARTESIAN_POINT('',(36.9580196842388,-1.39337735599387,-8.65357748012833));
#61255=CARTESIAN_POINT('',(36.958019684865,8.05522481984854,-8.65357747851728));
#61256=CARTESIAN_POINT('Ctrl Pts',(36.9580197773588,-1.66076081124402,-8.65357724055094));
#61257=CARTESIAN_POINT('Ctrl Pts',(36.9766488117873,-1.65672078778712,-8.60564880822258));
#61258=CARTESIAN_POINT('Ctrl Pts',(36.9968186458683,-1.6526640807411,-8.5583076754036));
#61259=CARTESIAN_POINT('Ctrl Pts',(37.0508280242562,-1.6424719350196,-8.44204107296676));
#61260=CARTESIAN_POINT('Ctrl Pts',(37.0864609765807,-1.63630295383903,-8.37404785157304));
#61261=CARTESIAN_POINT('Ctrl Pts',(37.1394253456699,-1.62773492932436,-8.2837640407794));
#61262=CARTESIAN_POINT('Ctrl Pts',(37.1539909881947,-1.62543263236425,-8.25989857947043));
#61263=CARTESIAN_POINT('Ctrl Pts',(37.1795579860137,-1.62147711970216,-8.21960440162423));
#61264=CARTESIAN_POINT('Ctrl Pts',(37.190352247854,-1.61983153500462,-8.20304710237475));
#61265=CARTESIAN_POINT('Ctrl Pts',(37.2126966282331,-1.61647248174447,-8.16967930526093));
#61266=CARTESIAN_POINT('Ctrl Pts',(37.2242589418237,-1.61475866209417,-8.15287898010722));
#61267=CARTESIAN_POINT('Ctrl Pts',(37.2540704193083,-1.61039891078306,-8.11072032099696));
#61268=CARTESIAN_POINT('Ctrl Pts',(37.2726020115671,-1.60774248286012,-8.08556756311285));
#61269=CARTESIAN_POINT('Ctrl Pts',(37.3548060377018,-1.59617842274454,-7.97842712010962));
#61270=CARTESIAN_POINT('Ctrl Pts',(37.423249407921,-1.58708985601911,-7.90026018662994));
#61271=CARTESIAN_POINT('Ctrl Pts',(37.6012974123963,-1.56466771010006,-7.72166160899465));
#61272=CARTESIAN_POINT('Ctrl Pts',(37.7155753632623,-1.55122298613764,-7.62648481102988));
#61273=CARTESIAN_POINT('Ctrl Pts',(37.8732631973737,-1.53419916170227,-7.51814570967567));
#61274=CARTESIAN_POINT('Ctrl Pts',(37.9092813482138,-1.53040540932297,-7.49479297976078));
#61275=CARTESIAN_POINT('Ctrl Pts',(37.971549393283,-1.52402605819973,-7.45674832044312));
#61276=CARTESIAN_POINT('Ctrl Pts',(37.9974844834706,-1.52141988073497,-7.44156231588705));
#61277=CARTESIAN_POINT('Ctrl Pts',(38.035805085137,-1.51764951415879,-7.42007820455439));
#61278=CARTESIAN_POINT('Ctrl Pts',(38.0479700605679,-1.51646421217904,-7.41339572543235));
#61279=CARTESIAN_POINT('Ctrl Pts',(38.0688104796859,-1.51445414223008,-7.40218135838208));
#61280=CARTESIAN_POINT('Ctrl Pts',(38.0774565761698,-1.51362622209264,-7.39759665534387));
#61281=CARTESIAN_POINT('Ctrl Pts',(38.0977023927963,-1.51170154169669,-7.38701885458659));
#61282=CARTESIAN_POINT('Ctrl Pts',(38.1093232671032,-1.51060732096031,-7.3810672394568));
#61283=CARTESIAN_POINT('Ctrl Pts',(38.1439288064997,-1.50737817668478,-7.36369826652627));
#61284=CARTESIAN_POINT('Ctrl Pts',(38.1670493450435,-1.50525875690302,-7.35255330232061));
#61285=CARTESIAN_POINT('Ctrl Pts',(38.297321213849,-1.49350260381528,-7.29230760790032));
#61286=CARTESIAN_POINT('Ctrl Pts',(38.4078048335977,-1.48422260090457,-7.25075745143956));
#61287=CARTESIAN_POINT('Ctrl Pts',(38.6369965082939,-1.46548734462016,-7.1833073124018));
#61288=CARTESIAN_POINT('Ctrl Pts',(38.7554949949892,-1.45605799133323,-7.15795316794812));
#61289=CARTESIAN_POINT('Ctrl Pts',(38.946442035062,-1.44070609476772,-7.13194698285513));
#61290=CARTESIAN_POINT('Ctrl Pts',(39.0178800615771,-1.43493045182367,-7.12545318927569));
#61291=CARTESIAN_POINT('Ctrl Pts',(39.1168104360454,-1.42681871763883,-7.12090347068267));
#61292=CARTESIAN_POINT('Ctrl Pts',(39.1441435869574,-1.42456583577932,-7.12011319119244));
#61293=CARTESIAN_POINT('Ctrl Pts',(39.1911397853741,-1.42066861417859,-7.11955599150702));
#61294=CARTESIAN_POINT('Ctrl Pts',(39.2107978927907,-1.41903133753692,-7.11956391921353));
#61295=CARTESIAN_POINT('Ctrl Pts',(39.24856677444,-1.41587080542725,-7.12004212700813));
#61296=CARTESIAN_POINT('Ctrl Pts',(39.2666767424749,-1.41434878359187,-7.12047608120949));
#61297=CARTESIAN_POINT('Ctrl Pts',(39.3146419236564,-1.41029915895054,-7.12216770379771));
#61298=CARTESIAN_POINT('Ctrl Pts',(39.344480562112,-1.40776091913265,-7.12377718470187));
#61299=CARTESIAN_POINT('Ctrl Pts',(39.46315474601,-1.39758477488507,-7.13239829563719));
#61300=CARTESIAN_POINT('Ctrl Pts',(39.5515892562966,-1.38981672839708,-7.14378724075549));
#61301=CARTESIAN_POINT('Ctrl Pts',(39.799559249943,-1.36750168420545,-7.18983598010339));
#61302=CARTESIAN_POINT('Ctrl Pts',(39.9564914263345,-1.3527127722752,-7.23585687535715));
#61303=CARTESIAN_POINT('Ctrl Pts',(40.1684505844484,-1.33232977448233,-7.32221033155718));
#61304=CARTESIAN_POINT('Ctrl Pts',(40.2283249637459,-1.326528564027,-7.34951647222082));
#61305=CARTESIAN_POINT('Ctrl Pts',(40.3032950888115,-1.31926664362761,-7.38749535137323));
#61306=CARTESIAN_POINT('Ctrl Pts',(40.3194857285393,-1.317698520319,-7.39593026376321));
#61307=CARTESIAN_POINT('Ctrl Pts',(40.3457246639721,-1.31515922787757,-7.40998217938844));
#61308=CARTESIAN_POINT('Ctrl Pts',(40.3558310438408,-1.31418167787483,-7.4154882073428));
#61309=CARTESIAN_POINT('Ctrl Pts',(40.3747953825199,-1.31234880729299,-7.42599732488529));
#61310=CARTESIAN_POINT('Ctrl Pts',(40.3836617978339,-1.31149249314473,-7.43098443624007));
#61311=CARTESIAN_POINT('Ctrl Pts',(40.4074259078356,-1.30919825212118,-7.44455025554639));
#61312=CARTESIAN_POINT('Ctrl Pts',(40.4222641254231,-1.3077666801506,-7.4532328986108));
#61313=CARTESIAN_POINT('Ctrl Pts',(40.4798920833177,-1.30220518078551,-7.4877888112491));
#61314=CARTESIAN_POINT('Ctrl Pts',(40.5219675957105,-1.29814099102921,-7.51483686261072));
#61315=CARTESIAN_POINT('Ctrl Pts',(40.6869677085935,-1.28205523210234,-7.62833036786038));
#61316=CARTESIAN_POINT('Ctrl Pts',(40.8025216512016,-1.27043253054818,-7.7248997682733));
#61317=CARTESIAN_POINT('Ctrl Pts',(40.9905344433623,-1.24943710216797,-7.91457186834187));
#61318=CARTESIAN_POINT('Ctrl Pts',(41.0665915785064,-1.24017176125122,-8.00338169173194));
#61319=CARTESIAN_POINT('Ctrl Pts',(41.1545022838283,-1.22808684187491,-8.12258890456953));
#61320=CARTESIAN_POINT('Ctrl Pts',(41.1726158571275,-1.2255116862948,-8.14818390656078));
#61321=CARTESIAN_POINT('Ctrl Pts',(41.2016896353693,-1.22122862236032,-8.19101783612297));
#61322=CARTESIAN_POINT('Ctrl Pts',(41.2129401670582,-1.21953167951824,-8.2080559464638));
#61323=CARTESIAN_POINT('Ctrl Pts',(41.2345226787362,-1.21619606606693,-8.24166386036473));
#61324=CARTESIAN_POINT('Ctrl Pts',(41.2448724917561,-1.2145582120095,-8.25822037352323));
#61325=CARTESIAN_POINT('Ctrl Pts',(41.2671678639451,-1.21094310288419,-8.29487139297771));
#61326=CARTESIAN_POINT('Ctrl Pts',(41.2790242017547,-1.20896282708215,-8.31501749882002));
#61327=CARTESIAN_POINT('Ctrl Pts',(41.3193171015431,-1.20202413738088,-8.38582359597382));
#61328=CARTESIAN_POINT('Ctrl Pts',(41.3462082035547,-1.19701304880252,-8.43733415735116));
#61329=CARTESIAN_POINT('Ctrl Pts',(41.4543816984186,-1.17507832928614,-8.6642068304185));
#61330=CARTESIAN_POINT('Ctrl Pts',(41.5162214034485,-1.15757111050607,-8.84802263022129));
#61331=CARTESIAN_POINT('Ctrl Pts',(41.5656647877552,-1.13579929414333,-9.08677098868994));
#61332=CARTESIAN_POINT('Ctrl Pts',(41.5743624743452,-1.13130748550425,-9.13664691923469));
#61333=CARTESIAN_POINT('Ctrl Pts',(41.5862308485587,-1.12390814916167,-9.22021062556128));
#61334=CARTESIAN_POINT('Ctrl Pts',(41.5902764816189,-1.1209714126182,-9.25375673613673));
#61335=CARTESIAN_POINT('Ctrl Pts',(41.595048507954,-1.11682070853175,-9.30182659587809));
#61336=CARTESIAN_POINT('Ctrl Pts',(41.5963519511122,-1.11557949832043,-9.31628707989927));
#61337=CARTESIAN_POINT('Ctrl Pts',(41.5984027586263,-1.1134206729372,-9.34160028372474));
#61338=CARTESIAN_POINT('Ctrl Pts',(41.5992075576521,-1.11250008842168,-9.35244750587373));
#61339=CARTESIAN_POINT('Ctrl Pts',(41.6008172606843,-1.11048253215298,-9.37633867575441));
#61340=CARTESIAN_POINT('Ctrl Pts',(41.6015894919113,-1.10938732634205,-9.3893841994733));
#61341=CARTESIAN_POINT('Ctrl Pts',(41.6035661750105,-1.10615214223569,-9.42812715203864));
#61342=CARTESIAN_POINT('Ctrl Pts',(41.6044648137248,-1.10402775436498,-9.45383942144602));
#61343=CARTESIAN_POINT('Ctrl Pts',(41.60695111997,-1.09324755761583,-9.58543716331371));
#61344=CARTESIAN_POINT('Ctrl Pts',(41.6019580386535,-1.08487582065179,-9.691343368924));
#61345=CARTESIAN_POINT('Ctrl Pts',(41.5795849289382,-1.06931382989583,-9.88822827717988));
#61346=CARTESIAN_POINT('Ctrl Pts',(41.5639095814976,-1.06212387074988,-9.97919216090846));
#61347=CARTESIAN_POINT('Ctrl Pts',(41.5193049728559,-1.04658145069881,-10.1712968150664));
#61348=CARTESIAN_POINT('Ctrl Pts',(41.4888932636008,-1.03822097813879,-10.271885571013));
#61349=CARTESIAN_POINT('Ctrl Pts',(41.4412610993584,-1.02715265863564,-10.3988066243859));
#61350=CARTESIAN_POINT('Ctrl Pts',(41.4299640774878,-1.02463805584239,-10.4272468479339));
#61351=CARTESIAN_POINT('Ctrl Pts',(41.4102884945814,-1.02042825487334,-10.4741514359711));
#61352=CARTESIAN_POINT('Ctrl Pts',(41.4022132483537,-1.01874325094457,-10.4927398586336));
#61353=CARTESIAN_POINT('Ctrl Pts',(41.3858568728235,-1.01541062257731,-10.5291254501065));
#61354=CARTESIAN_POINT('Ctrl Pts',(41.3775908493757,-1.01376361973527,-10.5469277038824));
#61355=CARTESIAN_POINT('Ctrl Pts',(41.3588209290888,-1.01010267730889,-10.5860898421337));
#61356=CARTESIAN_POINT('Ctrl Pts',(41.3482161034861,-1.00808541351048,-10.6073986983403));
#61357=CARTESIAN_POINT('Ctrl Pts',(41.3098746085859,-1.00096362995335,-10.6816567535784));
#61358=CARTESIAN_POINT('Ctrl Pts',(41.2804846055716,-0.995803201024133,
-10.7337217191006));
#61359=CARTESIAN_POINT('Ctrl Pts',(41.1489059759915,-0.973851654072483,
-10.9477756001797));
#61360=CARTESIAN_POINT('Ctrl Pts',(41.0295074101418,-0.956499724058424,
-11.098342645472));
#61361=CARTESIAN_POINT('Ctrl Pts',(40.8580982236152,-0.934951438980654,
-11.2682889457144));
#61362=CARTESIAN_POINT('Ctrl Pts',(40.8215519556371,-0.930521510929797,
-11.3023339647333));
#61363=CARTESIAN_POINT('Ctrl Pts',(40.7587857770584,-0.923211493610641,
-11.3572553577535));
#61364=CARTESIAN_POINT('Ctrl Pts',(40.7331425864996,-0.920303007053459,
-11.3787656100313));
#61365=CARTESIAN_POINT('Ctrl Pts',(40.6957824768088,-0.916184589791054,
-11.4087985521356));
#61366=CARTESIAN_POINT('Ctrl Pts',(40.6844259905158,-0.914947966871668,
-11.4177603425062));
#61367=CARTESIAN_POINT('Ctrl Pts',(40.664471159105,-0.912802462096916,-11.4332172968114));
#61368=CARTESIAN_POINT('Ctrl Pts',(40.6559090716544,-0.911890584082797,
-11.4397579015594));
#61369=CARTESIAN_POINT('Ctrl Pts',(40.6368726519571,-0.909882422397098,
-11.4540983510461));
#61370=CARTESIAN_POINT('Ctrl Pts',(40.6263783841342,-0.908787973804472,
-11.4618707224961));
#61371=CARTESIAN_POINT('Ctrl Pts',(40.5950627594769,-0.905557433024289,
-11.4846714457539));
#61372=CARTESIAN_POINT('Ctrl Pts',(40.5740626014759,-0.903436864613035,
-11.4994529385751));
#61373=CARTESIAN_POINT('Ctrl Pts',(40.4559784833714,-0.891739579041574,
-11.5797726455348));
#61374=CARTESIAN_POINT('Ctrl Pts',(40.3544314217979,-0.882514873260403,
-11.6384967681672));
#61375=CARTESIAN_POINT('Ctrl Pts',(40.1403425388874,-0.863857246839099,
-11.7422475800258));
#61376=CARTESIAN_POINT('Ctrl Pts',(40.0278851281187,-0.85445035687532,-11.7866443225055));
#61377=CARTESIAN_POINT('Ctrl Pts',(39.8433689980804,-0.839065197000954,
-11.8438745786727));
#61378=CARTESIAN_POINT('Ctrl Pts',(39.7732366405281,-0.833230515409785,
-11.8621993639853));
#61379=CARTESIAN_POINT('Ctrl Pts',(39.6755562385137,-0.825050117861934,
-11.8830610912064));
#61380=CARTESIAN_POINT('Ctrl Pts',(39.6486274099998,-0.822789573756093,
-11.8883322169841));
#61381=CARTESIAN_POINT('Ctrl Pts',(39.6022457284012,-0.818883344256368,
-11.896589845375));
#61382=CARTESIAN_POINT('Ctrl Pts',(39.5828350998348,-0.81724480938281,-11.8998004671481));
#61383=CARTESIAN_POINT('Ctrl Pts',(39.5430830818689,-0.813880157117593,
-11.9058756492042));
#61384=CARTESIAN_POINT('Ctrl Pts',(39.5227400764741,-0.812153505219321,
-11.908718449196));
#61385=CARTESIAN_POINT('Ctrl Pts',(39.4706528571842,-0.807718762567634,
-11.915318327187));
#61386=CARTESIAN_POINT('Ctrl Pts',(39.4388666646208,-0.804999427771179,
-11.9187036532854));
#61387=CARTESIAN_POINT('Ctrl Pts',(39.2879351167644,-0.792018143778195,
-11.9317422740328));
#61388=CARTESIAN_POINT('Ctrl Pts',(39.1682663773695,-0.781510328802102,
-11.9331371720131));
#61389=CARTESIAN_POINT('Ctrl Pts',(38.9316588599438,-0.760347580343208,
-11.9182553937519));
#61390=CARTESIAN_POINT('Ctrl Pts',(38.8150118849167,-0.749726470199695,
-11.9022802890558));
#61391=CARTESIAN_POINT('Ctrl Pts',(38.6502345517776,-0.734682243548663,
-11.8672637779487));
#61392=CARTESIAN_POINT('Ctrl Pts',(38.6008110087779,-0.73016617352328,-11.8551104984827));
#61393=CARTESIAN_POINT('Ctrl Pts',(38.5191540891722,-0.722731874027611,
-11.8322606021942));
#61394=CARTESIAN_POINT('Ctrl Pts',(38.4866955948103,-0.719784115191778,
-11.8224333093868));
#61395=CARTESIAN_POINT('Ctrl Pts',(38.4406307911765,-0.71562082447408,-11.8074159831629));
#61396=CARTESIAN_POINT('Ctrl Pts',(38.4268487619857,-0.71437783381426,-11.8027843426559));
#61397=CARTESIAN_POINT('Ctrl Pts',(38.4028291182034,-0.712217075456797,
-11.7944690725746));
#61398=CARTESIAN_POINT('Ctrl Pts',(38.3925733104857,-0.711296319885992,
-11.7908405607466));
#61399=CARTESIAN_POINT('Ctrl Pts',(38.3700658375248,-0.70927978409319,-11.7827051661761));
#61400=CARTESIAN_POINT('Ctrl Pts',(38.3578257878058,-0.708185755673206,
-11.7781679813425));
#61401=CARTESIAN_POINT('Ctrl Pts',(38.3216441983335,-0.704957789828243,
-11.7644200185411));
#61402=CARTESIAN_POINT('Ctrl Pts',(38.2978113614097,-0.702839339278392,
-11.7549252801234));
#61403=CARTESIAN_POINT('Ctrl Pts',(38.1776224562475,-0.692172910258089,
-11.7048008008837));
#61404=CARTESIAN_POINT('Ctrl Pts',(38.0838249194648,-0.683901816976493,
-11.6582947693905));
#61405=CARTESIAN_POINT('Ctrl Pts',(37.9167866956374,-0.668733845661413,
-11.5614302098471));
#61406=CARTESIAN_POINT('Ctrl Pts',(37.842740648434,-0.661833368137556,-11.5128459108845));
#61407=CARTESIAN_POINT('Ctrl Pts',(37.683433909221,-0.646244850846359,-11.3952599248691));
#61408=CARTESIAN_POINT('Ctrl Pts',(37.599882706456,-0.637536988788356,-11.3242955190626));
#61409=CARTESIAN_POINT('Ctrl Pts',(37.4993221124513,-0.626077509836954,
-11.2263239470278));
#61410=CARTESIAN_POINT('Ctrl Pts',(37.4776003240274,-0.623537950713253,
-11.2043295180832));
#61411=CARTESIAN_POINT('Ctrl Pts',(37.4423063224035,-0.619297982495971,
-11.1671872987514));
#61412=CARTESIAN_POINT('Ctrl Pts',(37.4284911242284,-0.617608083252113,
-11.1522745430868));
#61413=CARTESIAN_POINT('Ctrl Pts',(37.4017413189407,-0.614274413073817,
-11.1226552113002));
#61414=CARTESIAN_POINT('Ctrl Pts',(37.3887940170948,-0.612631345239832,
-11.1079621907212));
#61415=CARTESIAN_POINT('Ctrl Pts',(37.3577461479169,-0.608617170194724,
-11.0718484420184));
#61416=CARTESIAN_POINT('Ctrl Pts',(37.3398384696034,-0.606238524660221,
-11.0502666310931));
#61417=CARTESIAN_POINT('Ctrl Pts',(37.2776769512682,-0.597748231625329,
-10.972628203479));
#61418=CARTESIAN_POINT('Ctrl Pts',(37.2355511506408,-0.591556756191932,
-10.9149251180755));
#61419=CARTESIAN_POINT('Ctrl Pts',(37.0954417969937,-0.569301551086183,
-10.7038889284044));
#61420=CARTESIAN_POINT('Ctrl Pts',(37.0123487271616,-0.552802870997992,
-10.5414212515693));
#61421=CARTESIAN_POINT('Ctrl Pts',(36.9320531266636,-0.532457693614852,
-10.3277584322718));
#61422=CARTESIAN_POINT('Ctrl Pts',(36.9169950902045,-0.528349990465802,
-10.2838763381606));
#61423=CARTESIAN_POINT('Ctrl Pts',(36.8937773224602,-0.521508468361763,
-10.2092507123473));
#61424=CARTESIAN_POINT('Ctrl Pts',(36.8849412486945,-0.518750335067983,
-10.178731858202));
#61425=CARTESIAN_POINT('Ctrl Pts',(36.873038928146,-0.514804431214643,-10.1343489801836));
#61426=CARTESIAN_POINT('Ctrl Pts',(36.8694871069858,-0.513592814716964,
-10.1206204293313));
#61427=CARTESIAN_POINT('Ctrl Pts',(36.8636825334453,-0.511553911240571,
-10.0973372897143));
#61428=CARTESIAN_POINT('Ctrl Pts',(36.8613665767668,-0.510723209795483,
-10.0877992572794));
#61429=CARTESIAN_POINT('Ctrl Pts',(36.8561579064997,-0.508814332869713,
-10.0657603925521));
#61430=CARTESIAN_POINT('Ctrl Pts',(36.8533067302849,-0.507738480842667,
-10.0532502082991));
#61431=CARTESIAN_POINT('Ctrl Pts',(36.8454483200985,-0.50468006837751,-10.017449790817));
#61432=CARTESIAN_POINT('Ctrl Pts',(36.8406865762645,-0.502710359357819,
-9.99410628726866));
#61433=CARTESIAN_POINT('Ctrl Pts',(36.8087011117947,-0.488547564514565,
-9.82447233019233));
#61434=CARTESIAN_POINT('Ctrl Pts',(36.7947531159001,-0.476947183049444,
-9.67598271019004));
#61435=CARTESIAN_POINT('Ctrl Pts',(36.794494922637,-0.45416971615562,-9.38520611973058));
#61436=CARTESIAN_POINT('Ctrl Pts',(36.8069304179357,-0.443038497416284,
-9.24356173204293));
#61437=CARTESIAN_POINT('Ctrl Pts',(36.8384305508979,-0.428442930832616,
-9.06642904939711));
#61438=CARTESIAN_POINT('Ctrl Pts',(36.8459709416617,-0.425335770726453,
-9.0291729571566));
#61439=CARTESIAN_POINT('Ctrl Pts',(36.8592619787915,-0.420387694474125,
-8.97066976464539));
#61440=CARTESIAN_POINT('Ctrl Pts',(36.8644272279409,-0.418565198507036,
-8.94929499398913));
#61441=CARTESIAN_POINT('Ctrl Pts',(36.8746141487335,-0.415145883826236,
-8.90953537515891));
#61442=CARTESIAN_POINT('Ctrl Pts',(36.8795627175104,-0.413551512429558,
-8.89113342465414));
#61443=CARTESIAN_POINT('Ctrl Pts',(36.8912736753095,-0.409921562622533,
-8.84956069051287));
#61444=CARTESIAN_POINT('Ctrl Pts',(36.8981671433941,-0.407881922372731,
-8.82642937929033));
#61445=CARTESIAN_POINT('Ctrl Pts',(36.9205263324678,-0.40154826374691,-8.75532945902034));
#61446=CARTESIAN_POINT('Ctrl Pts',(36.9371513812334,-0.39721769157694,-8.70774345322431));
#61447=CARTESIAN_POINT('Ctrl Pts',(36.9561742884834,-0.392620226322211,
-8.65833649288737));
#61448=CARTESIAN_POINT('Ctrl Pts',(36.9570951029448,-0.392398486495653,
-8.65595622638362));
#61449=CARTESIAN_POINT('Ctrl Pts',(36.9580196850438,-0.392176638896471,
-8.65357747805726));
#61450=CARTESIAN_POINT('',(36.7946201876944,-0.197865522983575,-9.52404976188649));
#61451=CARTESIAN_POINT('Ctrl Pts',(36.958019684865,-0.127039975641411,-8.65357747851736));
#61452=CARTESIAN_POINT('Ctrl Pts',(36.9576505343558,-0.127124228813632,
-8.65452722236091));
#61453=CARTESIAN_POINT('Ctrl Pts',(36.957281985783,-0.127208451975847,-8.65547720477834));
#61454=CARTESIAN_POINT('Ctrl Pts',(36.9326587191942,-0.132842740466077,
-8.71906671381011));
#61455=CARTESIAN_POINT('Ctrl Pts',(36.9110349057488,-0.138260333134959,
-8.78270226913262));
#61456=CARTESIAN_POINT('Ctrl Pts',(36.8275328646549,-0.161858681809033,
-9.0670115969281));
#61457=CARTESIAN_POINT('Ctrl Pts',(36.7947106993761,-0.179316343464792,
-9.29493353410961));
#61458=CARTESIAN_POINT('Ctrl Pts',(36.7946201876944,-0.197865522983575,
-9.52404976188649));
#61459=CARTESIAN_POINT('Ctrl Pts',(36.7946201867286,-0.197865721158756,
-9.52405220971134));
#61460=CARTESIAN_POINT('Ctrl Pts',(36.7946053573966,-0.200912647768918,
-9.56168730295258));
#61461=CARTESIAN_POINT('Ctrl Pts',(36.7954737972968,-0.203982368590893,
-9.59931586672318));
#61462=CARTESIAN_POINT('Ctrl Pts',(36.7981130034701,-0.208649764404742,
-9.65598270848096));
#61463=CARTESIAN_POINT('Ctrl Pts',(36.799228538166,-0.210227559088422,-9.67504652365907));
#61464=CARTESIAN_POINT('Ctrl Pts',(36.8018618542569,-0.213336360028488,
-9.71241294165262));
#61465=CARTESIAN_POINT('Ctrl Pts',(36.8033625044052,-0.214866737667036,
-9.73071546403343));
#61466=CARTESIAN_POINT('Ctrl Pts',(36.806768924481,-0.217928317746531,-9.76713592921464));
#61467=CARTESIAN_POINT('Ctrl Pts',(36.8086712600725,-0.21945931457882,-9.78525296839222));
#61468=CARTESIAN_POINT('Ctrl Pts',(36.8143052509201,-0.223568639754768,
-9.8336130752302));
#61469=CARTESIAN_POINT('Ctrl Pts',(36.8184060107029,-0.226158207996919,
-9.86380872622567));
#61470=CARTESIAN_POINT('Ctrl Pts',(36.8378881747162,-0.237028004862082,
-9.98933175290926));
#61471=CARTESIAN_POINT('Ctrl Pts',(36.8584267388163,-0.245463278208587,
-10.0837537458843));
#61472=CARTESIAN_POINT('Ctrl Pts',(36.9352444489017,-0.27061354709357,-10.3566897523803));
#61473=CARTESIAN_POINT('Ctrl Pts',(37.0067255259323,-0.287644922256015,
-10.5301709218145));
#61474=CARTESIAN_POINT('Ctrl Pts',(37.102620144272,-0.305013488540014,-10.7026920129553));
#61475=CARTESIAN_POINT('Ctrl Pts',(37.1077230256865,-0.305924935593701,
-10.7117340930467));
#61476=CARTESIAN_POINT('Ctrl Pts',(37.1288018071162,-0.309637505508219,
-10.7485261570884));
#61477=CARTESIAN_POINT('Ctrl Pts',(37.1452735711858,-0.312418034000643,
-10.775990730988));
#61478=CARTESIAN_POINT('Ctrl Pts',(37.169846521585,-0.316389535127212,-10.8151674456714));
#61479=CARTESIAN_POINT('Ctrl Pts',(37.1775100073349,-0.317604770564152,
-10.827148011701));
#61480=CARTESIAN_POINT('Ctrl Pts',(37.1906428809246,-0.319647519920078,
-10.8472833641629));
#61481=CARTESIAN_POINT('Ctrl Pts',(37.1960565391385,-0.320478485633885,
-10.8554735801572));
#61482=CARTESIAN_POINT('Ctrl Pts',(37.2086415065548,-0.322384763966443,
-10.8742620293065));
#61483=CARTESIAN_POINT('Ctrl Pts',(37.2158474516946,-0.323457784807811,
-10.8848365200646));
#61484=CARTESIAN_POINT('Ctrl Pts',(37.2366213090029,-0.32650071958759,-10.9148047430386));
#61485=CARTESIAN_POINT('Ctrl Pts',(37.2503920499149,-0.328457978449773,
-10.9340571588975));
#61486=CARTESIAN_POINT('Ctrl Pts',(37.3539473428187,-0.342770627150016,
-11.0744088952655));
#61487=CARTESIAN_POINT('Ctrl Pts',(37.4546696463228,-0.354515939781619,
-11.1870514656135));
#61488=CARTESIAN_POINT('Ctrl Pts',(37.6705368546013,-0.377567625247281,
-11.3870360840493));
#61489=CARTESIAN_POINT('Ctrl Pts',(37.7842793401836,-0.388825747650711,
-11.4749135738255));
#61490=CARTESIAN_POINT('Ctrl Pts',(37.9360640296467,-0.403456676568694,
-11.5718666985317));
#61491=CARTESIAN_POINT('Ctrl Pts',(37.9674106723213,-0.40645763295396,-11.5908946444739));
#61492=CARTESIAN_POINT('Ctrl Pts',(38.0178090738067,-0.411258939073821,
-11.6199319525411));
#61493=CARTESIAN_POINT('Ctrl Pts',(38.0365822569716,-0.413042339281843,
-11.6304154850886));
#61494=CARTESIAN_POINT('Ctrl Pts',(38.0724808193418,-0.416444752873385,
-11.649835638358));
#61495=CARTESIAN_POINT('Ctrl Pts',(38.0895783333149,-0.41806191553107,-11.6588204396461));
#61496=CARTESIAN_POINT('Ctrl Pts',(38.1287045597515,-0.421756382498635,
-11.6787838233279));
#61497=CARTESIAN_POINT('Ctrl Pts',(38.1507969293118,-0.423837996102882,
-11.6896319543115));
#61498=CARTESIAN_POINT('Ctrl Pts',(38.2225815847382,-0.430590315132939,
-11.7235236679048));
#61499=CARTESIAN_POINT('Ctrl Pts',(38.2728918989524,-0.435305675767486,
-11.7452077867128));
#61500=CARTESIAN_POINT('Ctrl Pts',(38.4834671916888,-0.454990944258609,
-11.8275620359684));
#61501=CARTESIAN_POINT('Ctrl Pts',(38.6492302437649,-0.470415778572469,
-11.8727320550079));
#61502=CARTESIAN_POINT('Ctrl Pts',(38.9175154726389,-0.49479893497931,-11.915845696525));
#61503=CARTESIAN_POINT('Ctrl Pts',(39.0175946853595,-0.503757827397114,
-11.9255570379214));
#61504=CARTESIAN_POINT('Ctrl Pts',(39.1381264955444,-0.514203001909242,
-11.929668414367));
#61505=CARTESIAN_POINT('Ctrl Pts',(39.1582623957683,-0.515936293450766,
-11.9301021948969));
#61506=CARTESIAN_POINT('Ctrl Pts',(39.1903133701821,-0.518674362851683,
-11.9303899885594));
#61507=CARTESIAN_POINT('Ctrl Pts',(39.2022254061207,-0.519687404601256,
-11.9304084672761));
#61508=CARTESIAN_POINT('Ctrl Pts',(39.2252407626419,-0.521635254040958,
-11.9302731935022));
#61509=CARTESIAN_POINT('Ctrl Pts',(39.2363436250541,-0.522570609573691,
-11.9301310529033));
#61510=CARTESIAN_POINT('Ctrl Pts',(39.2642566712128,-0.524912165465525,
-11.9295803698446));
#61511=CARTESIAN_POINT('Ctrl Pts',(39.2810647851144,-0.526313082427744,
-11.9290724250489));
#61512=CARTESIAN_POINT('Ctrl Pts',(39.3447909552646,-0.531594927491448,
-11.9264774701724));
#61513=CARTESIAN_POINT('Ctrl Pts',(39.3916534784455,-0.535418245935625,
-11.9231927032467));
#61514=CARTESIAN_POINT('Ctrl Pts',(39.5745100014636,-0.5502063709147,-11.9049803670079));
#61515=CARTESIAN_POINT('Ctrl Pts',(39.7092341211597,-0.560829435828447,
-11.8798358654208));
#61516=CARTESIAN_POINT('Ctrl Pts',(39.9609430511587,-0.581313284455666,
-11.8102306586759));
#61517=CARTESIAN_POINT('Ctrl Pts',(40.0780204781558,-0.591124493440695,
-11.767852498431));
#61518=CARTESIAN_POINT('Ctrl Pts',(40.2244078901485,-0.604179258208205,
-11.7016402381282));
#61519=CARTESIAN_POINT('Ctrl Pts',(40.2571817054246,-0.607154820870015,
-11.6859120330034));
#61520=CARTESIAN_POINT('Ctrl Pts',(40.3086962757693,-0.611925147577697,
-11.6597377002693));
#61521=CARTESIAN_POINT('Ctrl Pts',(40.3276763228127,-0.613703347318205,
-11.6497725831843));
#61522=CARTESIAN_POINT('Ctrl Pts',(40.3635120359704,-0.617101868061932,
-11.6303423229333));
#61523=CARTESIAN_POINT('Ctrl Pts',(40.3803918338899,-0.618720402820227,
-11.6209250050183));
#61524=CARTESIAN_POINT('Ctrl Pts',(40.4186056635731,-0.622426442660438,
-11.5989972931124));
#61525=CARTESIAN_POINT('Ctrl Pts',(40.4398635495797,-0.624518357516609,
-11.5863594580735));
#61526=CARTESIAN_POINT('Ctrl Pts',(40.5081912624154,-0.631344201179292,
-11.5442992857618));
#61527=CARTESIAN_POINT('Ctrl Pts',(40.5544347895556,-0.636124172988199,
-11.5135772087535));
#61528=CARTESIAN_POINT('Ctrl Pts',(40.7619700160412,-0.658349672976315,
-11.3651018753242));
#61529=CARTESIAN_POINT('Ctrl Pts',(40.9092524343812,-0.67644388810793,-11.2291585271754));
#61530=CARTESIAN_POINT('Ctrl Pts',(41.0701860122219,-0.698715351924136,
-11.0385203742085));
#61531=CARTESIAN_POINT('Ctrl Pts',(41.1011629268085,-0.703139428860597,
-10.9994218754691));
#61532=CARTESIAN_POINT('Ctrl Pts',(41.1508404815142,-0.710440860098934,
-10.9325482556356));
#61533=CARTESIAN_POINT('Ctrl Pts',(41.1702168998764,-0.713346538475557,
-10.9052957565473));
#61534=CARTESIAN_POINT('Ctrl Pts',(41.1971508153015,-0.717461569454214,
-10.8656903497441));
#61535=CARTESIAN_POINT('Ctrl Pts',(41.2051737986094,-0.718697561762455,
-10.8536610037202));
#61536=CARTESIAN_POINT('Ctrl Pts',(41.2190374425463,-0.720850539350313,
-10.8324627705233));
#61537=CARTESIAN_POINT('Ctrl Pts',(41.224925099825,-0.721770441437652,-10.8233256332378));
#61538=CARTESIAN_POINT('Ctrl Pts',(41.2377742678239,-0.723790347913513,
-10.8030847798643));
#61539=CARTESIAN_POINT('Ctrl Pts',(41.2447072421128,-0.724888548124252,
-10.7919636892401));
#61540=CARTESIAN_POINT('Ctrl Pts',(41.2646689946504,-0.728076920661878,
-10.7593526273752));
#61541=CARTESIAN_POINT('Ctrl Pts',(41.2774528568608,-0.730152503672205,
-10.7377135873744));
#61542=CARTESIAN_POINT('Ctrl Pts',(41.3499770859726,-0.742153955825786,
-10.6104392256674));
#61543=CARTESIAN_POINT('Ctrl Pts',(41.4020020328193,-0.751698734821834,
-10.5005898186922));
#61544=CARTESIAN_POINT('Ctrl Pts',(41.4893446289732,-0.770800223097494,
-10.2731322296154));
#61545=CARTESIAN_POINT('Ctrl Pts',(41.5244039337821,-0.780331317865127,
-10.1558284251204));
#61546=CARTESIAN_POINT('Ctrl Pts',(41.5649356343947,-0.795540738594206,
-9.96953473797695));
#61547=CARTESIAN_POINT('Ctrl Pts',(41.576618492484,-0.801057260919085,-9.90211354609797));
#61548=CARTESIAN_POINT('Ctrl Pts',(41.5888722589813,-0.808866554803386,
-9.80760635322329));
#61549=CARTESIAN_POINT('Ctrl Pts',(41.5918840865321,-0.811084440338512,
-9.78086601767553));
#61550=CARTESIAN_POINT('Ctrl Pts',(41.5963115129302,-0.814940373396231,
-9.73458895123191));
#61551=CARTESIAN_POINT('Ctrl Pts',(41.5979382776531,-0.816571751584984,
-9.71507462851267));
#61552=CARTESIAN_POINT('Ctrl Pts',(41.6007942883378,-0.819943145534581,
-9.67489418340964));
#61553=CARTESIAN_POINT('Ctrl Pts',(41.6019953383351,-0.82168389241997,-9.65422777706805));
#61554=CARTESIAN_POINT('Ctrl Pts',(41.6044082540926,-0.826201848283641,
-9.60081356017237));
#61555=CARTESIAN_POINT('Ctrl Pts',(41.6052178610343,-0.828991155719367,
-9.56805301227879));
#61556=CARTESIAN_POINT('Ctrl Pts',(41.605941310765,-0.843495569729395,-9.39890608698164));
#61557=CARTESIAN_POINT('Ctrl Pts',(41.5949246430416,-0.85553726854043,-9.2627482777573));
#61558=CARTESIAN_POINT('Ctrl Pts',(41.5526758034803,-0.878480180511616,
-9.01009392742088));
#61559=CARTESIAN_POINT('Ctrl Pts',(41.5241086247796,-0.889307105895066,
-8.89354782693177));
#61560=CARTESIAN_POINT('Ctrl Pts',(41.4692227238634,-0.905031672464801,
-8.72514823451885));
#61561=CARTESIAN_POINT('Ctrl Pts',(41.4495288153869,-0.910067874675566,
-8.67132786937599));
#61562=CARTESIAN_POINT('Ctrl Pts',(41.421331086298,-0.916525026755497,-8.60204412674338));
#61563=CARTESIAN_POINT('Ctrl Pts',(41.4145555721029,-0.918027428613019,
-8.5859030868021));
#61564=CARTESIAN_POINT('Ctrl Pts',(41.4030971195696,-0.920487709156965,
-8.55941994165993));
#61565=CARTESIAN_POINT('Ctrl Pts',(41.3985162347687,-0.921451268390977,
-8.54903475772972));
#61566=CARTESIAN_POINT('Ctrl Pts',(41.3896391063731,-0.923280448040879,
-8.52928940986313));
#61567=CARTESIAN_POINT('Ctrl Pts',(41.3853560029217,-0.924146866066089,
-8.5199238096804));
#61568=CARTESIAN_POINT('Ctrl Pts',(41.3734715017932,-0.926508209634124,
-8.49437187352784));
#61569=CARTESIAN_POINT('Ctrl Pts',(41.3657493326646,-0.927996095842519,
-8.47824186606038));
#61570=CARTESIAN_POINT('Ctrl Pts',(41.3329967440013,-0.934125112776471,
-8.41174298324939));
#61571=CARTESIAN_POINT('Ctrl Pts',(41.3063811123615,-0.938682184443969,
-8.36216886040706));
#61572=CARTESIAN_POINT('Ctrl Pts',(41.205358581952,-0.954736419501301,-8.18887819950842));
#61573=CARTESIAN_POINT('Ctrl Pts',(41.1215883563601,-0.965908567940397,
-8.07097498289049));
#61574=CARTESIAN_POINT('Ctrl Pts',(40.9528513914953,-0.986319857665062,
-7.87374664616077));
#61575=CARTESIAN_POINT('Ctrl Pts',(40.8717742230785,-0.995464373094813,
-7.79171098901711));
#61576=CARTESIAN_POINT('Ctrl Pts',(40.7616287364414,-1.00741361345873,-7.69520607401032));
#61577=CARTESIAN_POINT('Ctrl Pts',(40.7377186189714,-1.00998115489312,-7.67506719327893));
#61578=CARTESIAN_POINT('Ctrl Pts',(40.6975718811212,-1.0142547146104,-7.64256876468201));
#61579=CARTESIAN_POINT('Ctrl Pts',(40.6815577889091,-1.0159498628641,-7.62993922009585));
#61580=CARTESIAN_POINT('Ctrl Pts',(40.6498969706008,-1.01928424301281,-7.60561645421251));
#61581=CARTESIAN_POINT('Ctrl Pts',(40.6342645473025,-1.02092268072654,-7.59390715357581));
#61582=CARTESIAN_POINT('Ctrl Pts',(40.5995804165374,-1.02454188416313,-7.56858083986925));
#61583=CARTESIAN_POINT('Ctrl Pts',(40.5804691861955,-1.02652570207412,-7.55504923535757));
#61584=CARTESIAN_POINT('Ctrl Pts',(40.5130158612209,-1.03349413892013,-7.50875283754199));
#61585=CARTESIAN_POINT('Ctrl Pts',(40.4636847893441,-1.0385320505671,-7.47747398344665));
#61586=CARTESIAN_POINT('Ctrl Pts',(40.2457495452007,-1.06056219493239,-7.3501667855864));
#61587=CARTESIAN_POINT('Ctrl Pts',(40.0670215108104,-1.07814177149365,-7.2729468234314));
#61588=CARTESIAN_POINT('Ctrl Pts',(39.8331383965522,-1.0999115758875,-7.20390549084329));
#61589=CARTESIAN_POINT('Ctrl Pts',(39.7848388150505,-1.10433957284662,-7.19126732271379));
#61590=CARTESIAN_POINT('Ctrl Pts',(39.703566695604,-1.1116466695497,-7.17268356400458));
#61591=CARTESIAN_POINT('Ctrl Pts',(39.6708011300013,-1.11455414447533,-7.16590723786521));
#61592=CARTESIAN_POINT('Ctrl Pts',(39.6236823162561,-1.11867123011215,-7.15718341403897));
#61593=CARTESIAN_POINT('Ctrl Pts',(39.6094381139956,-1.11990751535879,-7.15467880801584));
#61594=CARTESIAN_POINT('Ctrl Pts',(39.5845464694439,-1.12205245815724,-7.15053311603004));
#61595=CARTESIAN_POINT('Ctrl Pts',(39.5739093965699,-1.12296411012867,-7.14883486428573));
#61596=CARTESIAN_POINT('Ctrl Pts',(39.550355274989,-1.12497176329352,-7.14523644896894));
#61597=CARTESIAN_POINT('Ctrl Pts',(39.537433703855,-1.12606593042892,-7.14336990751086));
#61598=CARTESIAN_POINT('Ctrl Pts',(39.4990620529146,-1.12929555090181,-7.13814563339019));
#61599=CARTESIAN_POINT('Ctrl Pts',(39.473571627328,-1.13141548994492,-7.13508983333882));
#61600=CARTESIAN_POINT('Ctrl Pts',(39.3436302962096,-1.14211574274377,-7.12161885937475));
#61601=CARTESIAN_POINT('Ctrl Pts',(39.2386134845332,-1.15041701082927,-7.1176392808032));
#61602=CARTESIAN_POINT('Ctrl Pts',(39.0440595157305,-1.16570462074215,-7.12300711738369));
#61603=CARTESIAN_POINT('Ctrl Pts',(38.9546683189064,-1.17269337024186,-7.13048553867086));
#61604=CARTESIAN_POINT('Ctrl Pts',(38.7588125346317,-1.18826846636985,-7.15795529539105));
#61605=CARTESIAN_POINT('Ctrl Pts',(38.6528703029104,-1.19687127925715,-7.18017781563946));
#61606=CARTESIAN_POINT('Ctrl Pts',(38.5191269931278,-1.20821225126242,-7.21779075354095));
#61607=CARTESIAN_POINT('Ctrl Pts',(38.4896264740927,-1.21074414275716,-7.22670240442171));
#61608=CARTESIAN_POINT('Ctrl Pts',(38.4409845819695,-1.21497455657757,-7.24242231831666));
#61609=CARTESIAN_POINT('Ctrl Pts',(38.4217430439486,-1.2166626638189,-7.248910956196));
#61610=CARTESIAN_POINT('Ctrl Pts',(38.3841035401946,-1.21999520008425,-7.26213683279161));
#61611=CARTESIAN_POINT('Ctrl Pts',(38.3657011508643,-1.22163894915328,-7.26885680231301));
#61612=CARTESIAN_POINT('Ctrl Pts',(38.3252554976667,-1.22528483647101,-7.28418876108049));
#61613=CARTESIAN_POINT('Ctrl Pts',(38.3032533988015,-1.22729020349183,-7.29290269027924));
#61614=CARTESIAN_POINT('Ctrl Pts',(38.2269475550794,-1.23432485861037,-7.32443388244236));
#61615=CARTESIAN_POINT('Ctrl Pts',(38.1733608057895,-1.23940827397468,-7.34891797104746));
#61616=CARTESIAN_POINT('Ctrl Pts',(37.9484489849288,-1.26138498917086,-7.4618383863218));
#61617=CARTESIAN_POINT('Ctrl Pts',(37.7872063104668,-1.27885290517371,-7.56872582852436));
#61618=CARTESIAN_POINT('Ctrl Pts',(37.6024725410414,-1.3005139505713,-7.7260417104039));
#61619=CARTESIAN_POINT('Ctrl Pts',(37.565480506542,-1.30494282118066,-7.75958457165736));
#61620=CARTESIAN_POINT('Ctrl Pts',(37.5054832969046,-1.31225118042522,-7.81749144157899));
#61621=CARTESIAN_POINT('Ctrl Pts',(37.4818953403318,-1.31515905563696,-7.84122773360221));
#61622=CARTESIAN_POINT('Ctrl Pts',(37.4488304221853,-1.31927659904696,-7.87591927996711));
#61623=CARTESIAN_POINT('Ctrl Pts',(37.4389464305759,-1.32051294954357,-7.88647857213508));
#61624=CARTESIAN_POINT('Ctrl Pts',(37.4218015959474,-1.32266631420537,-7.90512916143797));
#61625=CARTESIAN_POINT('Ctrl Pts',(37.4144995258508,-1.32358624891081,-7.9131814079284));
#61626=CARTESIAN_POINT('Ctrl Pts',(37.3985167688542,-1.32560594205811,-7.93104806818547));
#61627=CARTESIAN_POINT('Ctrl Pts',(37.3898613553141,-1.32670389922644,-7.94088425147982));
#61628=CARTESIAN_POINT('Ctrl Pts',(37.3648493224462,-1.32989085242544,-7.96978112858113));
#61629=CARTESIAN_POINT('Ctrl Pts',(37.3487096585906,-1.33196527864428,-7.98902865579706));
#61630=CARTESIAN_POINT('Ctrl Pts',(37.2561180866606,-1.34399791499374,-8.10303011362031));
#61631=CARTESIAN_POINT('Ctrl Pts',(37.1866365644862,-1.35357236251748,-8.20323918168507));
#61632=CARTESIAN_POINT('Ctrl Pts',(37.0631122753071,-1.3727165111079,-8.41389676733031));
#61633=CARTESIAN_POINT('Ctrl Pts',(37.0093448284768,-1.3822605754664,-8.52406698298727));
#61634=CARTESIAN_POINT('Ctrl Pts',(36.9621199005609,-1.39247710230569,-8.6430831418719));
#61635=CARTESIAN_POINT('Ctrl Pts',(36.9600605302133,-1.39292702021548,-8.64832682800744));
#61636=CARTESIAN_POINT('Ctrl Pts',(36.9580196842388,-1.39337735599387,-8.65357748012833));
#61637=CARTESIAN_POINT('Origin',(39.2,8.05522481984854,-9.525));
#61638=CARTESIAN_POINT('',(36.9580196848651,-2.92826949524753,-8.65357747851701));
#61639=CARTESIAN_POINT('',(36.9580195936563,-2.66377399804174,-8.65357771317761));
#61640=CARTESIAN_POINT('',(36.958019684865,8.05522481984854,-8.65357747851728));
#61641=CARTESIAN_POINT('',(36.7946202453594,-1.73347969461058,-9.5239135539112));
#61642=CARTESIAN_POINT('Ctrl Pts',(36.9580196848651,-2.92826949524753,-8.65357747851701));
#61643=CARTESIAN_POINT('Ctrl Pts',(36.9664653728173,-2.92624276699562,-8.63184856324372));
#61644=CARTESIAN_POINT('Ctrl Pts',(36.9752269914618,-2.92422984141651,-8.61024232509335));
#61645=CARTESIAN_POINT('Ctrl Pts',(36.9892742616844,-2.92113977904251,-8.57699796488788));
#61646=CARTESIAN_POINT('Ctrl Pts',(36.9943405140941,-2.92005102057367,-8.56526961916314));
#61647=CARTESIAN_POINT('Ctrl Pts',(37.0034676301304,-2.91813485665858,-8.54459446895908));
#61648=CARTESIAN_POINT('Ctrl Pts',(37.0074900351129,-2.91730531288517,-8.5356317579994));
#61649=CARTESIAN_POINT('Ctrl Pts',(37.017485748034,-2.91527966775965,-8.51371970917388));
#61650=CARTESIAN_POINT('Ctrl Pts',(37.0235194860318,-2.91408718298861,-8.50079841331756));
#61651=CARTESIAN_POINT('Ctrl Pts',(37.0435661262645,-2.9102194960717,-8.45884569215036));
#61652=CARTESIAN_POINT('Ctrl Pts',(37.0580485277825,-2.9075702850619,-8.43004052439141));
#61653=CARTESIAN_POINT('Ctrl Pts',(37.095221097092,-2.90109180436795,-8.35966720667705));
#61654=CARTESIAN_POINT('Ctrl Pts',(37.1185685129722,-2.89729274726006,-8.31846016148965));
#61655=CARTESIAN_POINT('Ctrl Pts',(37.2435567488603,-2.87811586658396,-8.1123021849734));
#61656=CARTESIAN_POINT('Ctrl Pts',(37.3636391382386,-2.86326336563732,-7.95937922375053));
#61657=CARTESIAN_POINT('Ctrl Pts',(37.5441880177366,-2.84286010390754,-7.77917553621361));
#61658=CARTESIAN_POINT('Ctrl Pts',(37.5892465045135,-2.83790254744708,-7.73751898765698));
#61659=CARTESIAN_POINT('Ctrl Pts',(37.6540693593975,-2.83090830098266,-7.68203312371446));
#61660=CARTESIAN_POINT('Ctrl Pts',(37.672526041737,-2.82893163471598,-7.66670732234453));
#61661=CARTESIAN_POINT('Ctrl Pts',(37.7065307022072,-2.82531383602521,-7.63931989059333));
#61662=CARTESIAN_POINT('Ctrl Pts',(37.7220035478372,-2.82367643426488,-7.62716795851445));
#61663=CARTESIAN_POINT('Ctrl Pts',(37.7536658787209,-2.82034210491862,-7.60292330453891));
#61664=CARTESIAN_POINT('Ctrl Pts',(37.7698621260741,-2.81864490211231,-7.59084208972367));
#61665=CARTESIAN_POINT('Ctrl Pts',(37.8107157083519,-2.81438325135221,-7.56116198944534));
#61666=CARTESIAN_POINT('Ctrl Pts',(37.8355561856122,-2.81180926190135,-7.54382270553107));
#61667=CARTESIAN_POINT('Ctrl Pts',(37.9445028502849,-2.80058784207084,-7.47079596702018));
#61668=CARTESIAN_POINT('Ctrl Pts',(38.0317257077326,-2.79176908765631,-7.41996873533486));
#61669=CARTESIAN_POINT('Ctrl Pts',(38.2619070864816,-2.76890460173019,-7.30455504405558));
#61670=CARTESIAN_POINT('Ctrl Pts',(38.4084608139233,-2.75470114299569,-7.24819170548262));
#61671=CARTESIAN_POINT('Ctrl Pts',(38.6169736417083,-2.73547180093228,-7.19058466916527));
#61672=CARTESIAN_POINT('Ctrl Pts',(38.6750767191795,-2.73021770336873,-7.17683651840131));
#61673=CARTESIAN_POINT('Ctrl Pts',(38.7514989067389,-2.72348681315844,-7.16173293385599));
#61674=CARTESIAN_POINT('Ctrl Pts',(38.7694012363258,-2.72192282034742,-7.15840556429335));
#61675=CARTESIAN_POINT('Ctrl Pts',(38.7975485828191,-2.71948545994758,-7.15350402334867));
#61676=CARTESIAN_POINT('Ctrl Pts',(38.8077684023428,-2.71860495829989,-7.15179231906073));
#61677=CARTESIAN_POINT('Ctrl Pts',(38.8291490599112,-2.71677262092749,-7.1483531900643));
#61678=CARTESIAN_POINT('Ctrl Pts',(38.8403115577687,-2.71582156509879,-7.14663822891784));
#61679=CARTESIAN_POINT('Ctrl Pts',(38.8685144605889,-2.71343177425542,-7.14250834868005));
#61680=CARTESIAN_POINT('Ctrl Pts',(38.8855699726061,-2.71199861653465,-7.1401975045989));
#61681=CARTESIAN_POINT('Ctrl Pts',(38.9565513242016,-2.70607844864992,-7.13135504436753));
#61682=CARTESIAN_POINT('Ctrl Pts',(39.0106708441463,-2.7016706182777,-7.12646729269734));
#61683=CARTESIAN_POINT('Ctrl Pts',(39.1887397394359,-2.68737452911187,-7.11645121725453));
#61684=CARTESIAN_POINT('Ctrl Pts',(39.3129275007018,-2.67772471675513,-7.11907267182811));
#61685=CARTESIAN_POINT('Ctrl Pts',(39.5712985918954,-2.65736934076381,-7.1445852796714));
#61686=CARTESIAN_POINT('Ctrl Pts',(39.7048426646519,-2.64668031436939,-7.16929143069441));
#61687=CARTESIAN_POINT('Ctrl Pts',(39.8672748190431,-2.63295702023391,-7.21379316767112));
#61688=CARTESIAN_POINT('Ctrl Pts',(39.8987838047482,-2.63026109697771,-7.22312387587738));
#61689=CARTESIAN_POINT('Ctrl Pts',(39.9498356927374,-2.62583137524336,-7.23938655451934));
#61690=CARTESIAN_POINT('Ctrl Pts',(39.9694983159628,-2.62411013766482,-7.24593118267668));
#61691=CARTESIAN_POINT('Ctrl Pts',(40.0075684337532,-2.62074647802022,-7.25915148570652));
#61692=CARTESIAN_POINT('Ctrl Pts',(40.0259838635023,-2.61910507676171,-7.26579950561746));
#61693=CARTESIAN_POINT('Ctrl Pts',(40.0694717464178,-2.61519353128294,-7.28210152035425));
#61694=CARTESIAN_POINT('Ctrl Pts',(40.0944670806706,-2.61291707238434,-7.29195203284477));
#61695=CARTESIAN_POINT('Ctrl Pts',(40.1821788643497,-2.60482458605003,-7.32822760537779));
#61696=CARTESIAN_POINT('Ctrl Pts',(40.2439273765639,-2.59893596088992,-7.35689068994492));
#61697=CARTESIAN_POINT('Ctrl Pts',(40.4131363967936,-2.58223816940257,-7.44434085920711));
#61698=CARTESIAN_POINT('Ctrl Pts',(40.517438459337,-2.57127273776156,-7.50876795016922));
#61699=CARTESIAN_POINT('Ctrl Pts',(40.7147154683156,-2.54933728009476,-7.65248977998178));
#61700=CARTESIAN_POINT('Ctrl Pts',(40.807491256365,-2.53839960018896,-7.73150186352585));
#61701=CARTESIAN_POINT('Ctrl Pts',(40.9117321389102,-2.52561446213817,-7.83489435834114));
#61702=CARTESIAN_POINT('Ctrl Pts',(40.9292904688979,-2.52344255234437,-7.85286405449222));
#61703=CARTESIAN_POINT('Ctrl Pts',(40.9555753484473,-2.5201669920687,-7.88062173948637));
#61704=CARTESIAN_POINT('Ctrl Pts',(40.9645080515691,-2.51904942333253,-7.89021070825897));
#61705=CARTESIAN_POINT('Ctrl Pts',(40.9807081918234,-2.51701525817689,-7.90788853235642));
#61706=CARTESIAN_POINT('Ctrl Pts',(40.9879995196439,-2.51609701343918,-7.91595404300137));
#61707=CARTESIAN_POINT('Ctrl Pts',(41.0048652849821,-2.51396627634168,-7.93486681390024));
#61708=CARTESIAN_POINT('Ctrl Pts',(41.0143969252349,-2.51275685806353,-7.94575142024874));
#61709=CARTESIAN_POINT('Ctrl Pts',(41.0456542870581,-2.50877054488772,-7.98210218902052));
#61710=CARTESIAN_POINT('Ctrl Pts',(41.0669479077926,-2.5060218916989,-8.00793729603912));
#61711=CARTESIAN_POINT('Ctrl Pts',(41.1186546487436,-2.49923795336438,-8.073410419126));
#61712=CARTESIAN_POINT('Ctrl Pts',(41.1483863159832,-2.49523671239902,-8.11356828170441));
#61713=CARTESIAN_POINT('Ctrl Pts',(41.2845579303251,-2.4762548398736,-8.31000410456368));
#61714=CARTESIAN_POINT('Ctrl Pts',(41.3735731068426,-2.46174208633795,-8.47753651898351));
#61715=CARTESIAN_POINT('Ctrl Pts',(41.4643539576898,-2.44169702180377,-8.71115438372618));
#61716=CARTESIAN_POINT('Ctrl Pts',(41.4844404553355,-2.43672199061006,-8.769371691334));
#61717=CARTESIAN_POINT('Ctrl Pts',(41.5092245938589,-2.42970823274468,-8.85127071592052));
#61718=CARTESIAN_POINT('Ctrl Pts',(41.5158339833155,-2.42773002566563,-8.87435243718446));
#61719=CARTESIAN_POINT('Ctrl Pts',(41.5272300326589,-2.4241102978097,-8.91652602202451));
#61720=CARTESIAN_POINT('Ctrl Pts',(41.5321300329015,-2.4224725216615,-8.93558531726609));
#61721=CARTESIAN_POINT('Ctrl Pts',(41.5415846756019,-2.4191383403646,-8.97432570660355));
#61722=CARTESIAN_POINT('Ctrl Pts',(41.5461263243038,-2.41744166828029,-8.99400829800271));
#61723=CARTESIAN_POINT('Ctrl Pts',(41.5568514513319,-2.41318317526516,-9.04331549837358));
#61724=CARTESIAN_POINT('Ctrl Pts',(41.5627245618393,-2.41061184314709,-9.07300311041458));
#61725=CARTESIAN_POINT('Ctrl Pts',(41.585671952114,-2.39942692152061,-9.20170807812199));
#61726=CARTESIAN_POINT('Ctrl Pts',(41.5970903521582,-2.39064343958362,-9.30161606706494));
#61727=CARTESIAN_POINT('Ctrl Pts',(41.6101511949565,-2.36797890325715,-9.55655650687202));
#61728=CARTESIAN_POINT('Ctrl Pts',(41.6031251808397,-2.35394546735695,-9.71157448205063));
#61729=CARTESIAN_POINT('Ctrl Pts',(41.5725456807447,-2.33469187519421,-9.92584653321972));
#61730=CARTESIAN_POINT('Ctrl Pts',(41.5614963006179,-2.32926228636641,-9.98650603050376));
#61731=CARTESIAN_POINT('Ctrl Pts',(41.5441425361879,-2.3223471705312,-10.0646168257901));
#61732=CARTESIAN_POINT('Ctrl Pts',(41.5399519925439,-2.32076858925726,-10.0825081027486));
#61733=CARTESIAN_POINT('Ctrl Pts',(41.5330705031569,-2.31831396969641,-10.110442571015));
#61734=CARTESIAN_POINT('Ctrl Pts',(41.530518902818,-2.31743063422273,-10.120518793134));
#61735=CARTESIAN_POINT('Ctrl Pts',(41.5250660502517,-2.31559780037572,-10.1414800844415));
#61736=CARTESIAN_POINT('Ctrl Pts',(41.5221535172115,-2.31464904203977,-10.152361845463));
#61737=CARTESIAN_POINT('Ctrl Pts',(41.5146369025587,-2.31227357597721,-10.1796756005211));
#61738=CARTESIAN_POINT('Ctrl Pts',(41.5099340742804,-2.31085230544626,-10.1960802907195));
#61739=CARTESIAN_POINT('Ctrl Pts',(41.4899306766198,-2.3050580412098,-10.2631542951848));
#61740=CARTESIAN_POINT('Ctrl Pts',(41.4731329754585,-2.30076006393799,-10.3133666062595));
#61741=CARTESIAN_POINT('Ctrl Pts',(41.4094935063357,-2.28610593610075,-10.4845948003884));
#61742=CARTESIAN_POINT('Ctrl Pts',(41.3545290712239,-2.27602299799529,-10.6023549900762));
#61743=CARTESIAN_POINT('Ctrl Pts',(41.224796689076,-2.25545787020721,-10.8302182485688));
#61744=CARTESIAN_POINT('Ctrl Pts',(41.1498779020061,-2.24500363664712,-10.9396960260322));
#61745=CARTESIAN_POINT('Ctrl Pts',(41.0458839470394,-2.23156636100812,-11.0676006297233));
#61746=CARTESIAN_POINT('Ctrl Pts',(41.0249237004292,-2.22890540409381,-11.0923409121332));
#61747=CARTESIAN_POINT('Ctrl Pts',(40.9898172083265,-2.22451820304751,-11.1321194935414));
#61748=CARTESIAN_POINT('Ctrl Pts',(40.9759655788389,-2.22280404991682,-11.1474132991636));
#61749=CARTESIAN_POINT('Ctrl Pts',(40.9485604466947,-2.2194435690897,-11.1769002307601));
#61750=CARTESIAN_POINT('Ctrl Pts',(40.9350265830803,-2.21779815786197,-11.1911094548241));
#61751=CARTESIAN_POINT('Ctrl Pts',(40.9023663495596,-2.21385938040228,-11.2245699815404));
#61752=CARTESIAN_POINT('Ctrl Pts',(40.8830855038397,-2.21155945620201,-11.2436658684604));
#61753=CARTESIAN_POINT('Ctrl Pts',(40.8128577232127,-2.2032676124161,-11.310904792846));
#61754=CARTESIAN_POINT('Ctrl Pts',(40.7601401834865,-2.197198175024,-11.3571371331581));
#61755=CARTESIAN_POINT('Ctrl Pts',(40.6106240806905,-2.18037584143536,-11.4771235659106));
#61756=CARTESIAN_POINT('Ctrl Pts',(40.5101357256124,-2.16947669416102,-11.5459366131396));
#61757=CARTESIAN_POINT('Ctrl Pts',(40.301652213206,-2.14782815261958,-11.6665982058393));
#61758=CARTESIAN_POINT('Ctrl Pts',(40.1941041194259,-2.13711040178768,-11.7185914528014));
#61759=CARTESIAN_POINT('Ctrl Pts',(40.0592039390597,-2.12447776094982,-11.7718385071051));
#61760=CARTESIAN_POINT('Ctrl Pts',(40.0351246759671,-2.12225335079219,-11.7808992936535));
#61761=CARTESIAN_POINT('Ctrl Pts',(39.9986006098808,-2.11892947689036,-11.7939779135871));
#61762=CARTESIAN_POINT('Ctrl Pts',(39.9862618326821,-2.11781512190141,-11.7982831019128));
#61763=CARTESIAN_POINT('Ctrl Pts',(39.963589417827,-2.11578384163529,-11.8059871669111));
#61764=CARTESIAN_POINT('Ctrl Pts',(39.9532673270887,-2.11486530375233,-11.8094166868403));
#61765=CARTESIAN_POINT('Ctrl Pts',(39.9291130923358,-2.11273005798033,-11.8172604183601));
#61766=CARTESIAN_POINT('Ctrl Pts',(39.9152637173031,-2.11151647065862,-11.8216195972571));
#61767=CARTESIAN_POINT('Ctrl Pts',(39.8690597536677,-2.10750050452594,-11.8357040735817));
#61768=CARTESIAN_POINT('Ctrl Pts',(39.8365379253333,-2.10472694514075,-11.844873721473));
#61769=CARTESIAN_POINT('Ctrl Pts',(39.754838541676,-2.09786563033089,-11.8660614816636));
#61770=CARTESIAN_POINT('Ctrl Pts',(39.7054531441479,-2.09381292943713,-11.8772186485999));
#61771=CARTESIAN_POINT('Ctrl Pts',(39.4661579753392,-2.07446602569077,-11.9233944656592));
#61772=CARTESIAN_POINT('Ctrl Pts',(39.2728558584254,-2.05965121769397,-11.937017957914));
#61773=CARTESIAN_POINT('Ctrl Pts',(39.0218807210343,-2.03951784346619,-11.9244817984788));
#61774=CARTESIAN_POINT('Ctrl Pts',(38.9638894331802,-2.03480822620075,-11.9194707450422));
#61775=CARTESIAN_POINT('Ctrl Pts',(38.8829261398952,-2.02811658586329,-11.9095050237585));
#61776=CARTESIAN_POINT('Ctrl Pts',(38.8597550139834,-2.02618810323699,-11.9063091594301));
#61777=CARTESIAN_POINT('Ctrl Pts',(38.8173305032682,-2.02263027375656,-11.8998259655057));
#61778=CARTESIAN_POINT('Ctrl Pts',(38.7980632795936,-2.02100422417672,-11.8966410216942));
#61779=CARTESIAN_POINT('Ctrl Pts',(38.7587410099753,-2.01766336751817,-11.8896479848832));
#61780=CARTESIAN_POINT('Ctrl Pts',(38.738691453329,-2.01594801491461,-11.8858184933378));
#61781=CARTESIAN_POINT('Ctrl Pts',(38.6879995138643,-2.01157927621064,-11.8754658846545));
#61782=CARTESIAN_POINT('Ctrl Pts',(38.6574323365234,-2.00891530506851,-11.8685986227104));
#61783=CARTESIAN_POINT('Ctrl Pts',(38.5140423517725,-1.99627151080999,-11.8334289772844));
#61784=CARTESIAN_POINT('Ctrl Pts',(38.4032537273423,-1.98605892900503,-11.7975687999894));
#61785=CARTESIAN_POINT('Ctrl Pts',(38.1579448335647,-1.96244969054331,-11.6980196570026));
#61786=CARTESIAN_POINT('Ctrl Pts',(38.025847369609,-1.94899394759567,-11.6295803707578));
#61787=CARTESIAN_POINT('Ctrl Pts',(37.8572415864665,-1.93124302197841,-11.5213827466607));
#61788=CARTESIAN_POINT('Ctrl Pts',(37.8144940996683,-1.926690331076,-11.4919567071594));
#61789=CARTESIAN_POINT('Ctrl Pts',(37.7587147158962,-1.92070918204399,-11.4508381951773));
#61790=CARTESIAN_POINT('Ctrl Pts',(37.7448134211079,-1.91921509494791,-11.4403558675428));
#61791=CARTESIAN_POINT('Ctrl Pts',(37.7229401471301,-1.91686013758172,-11.4234866127209));
#61792=CARTESIAN_POINT('Ctrl Pts',(37.7148933041467,-1.91599289866046,-11.417198547114));
#61793=CARTESIAN_POINT('Ctrl Pts',(37.6981944043813,-1.91419174307319,-11.4039773311442));
#61794=CARTESIAN_POINT('Ctrl Pts',(37.689549736058,-1.91325851486829,-11.397035221777));
#61795=CARTESIAN_POINT('Ctrl Pts',(37.6808576116197,-1.91231897341353,-11.3899555928775));
#61796=CARTESIAN_POINT('Ctrl Pts',(37.6807620905259,-1.91230864828542,-11.3898777799084));
#61797=CARTESIAN_POINT('Ctrl Pts',(37.6805720138282,-1.91228810209954,-11.389722916177));
#61798=CARTESIAN_POINT('Ctrl Pts',(37.680477458109,-1.91227788103222,-11.3896458655634));
#61799=CARTESIAN_POINT('Ctrl Pts',(37.6802891539906,-1.91225752587798,-11.389492398362));
#61800=CARTESIAN_POINT('Ctrl Pts',(37.6801954054617,-1.91224739177946,-11.389415981869));
#61801=CARTESIAN_POINT('Ctrl Pts',(37.6800085642005,-1.91222719418937,-11.3892636599806));
#61802=CARTESIAN_POINT('Ctrl Pts',(37.6799154714304,-1.91221713069567,-11.3891877547155));
#61803=CARTESIAN_POINT('Ctrl Pts',(37.6797297960113,-1.91219705857215,-11.3890363369682));
#61804=CARTESIAN_POINT('Ctrl Pts',(37.679637213312,-1.9121870499384,-11.388960824569));
#61805=CARTESIAN_POINT('Ctrl Pts',(37.6794524171043,-1.91216707230296,-11.3888100779622));
#61806=CARTESIAN_POINT('Ctrl Pts',(37.6793602035171,-1.91215710329381,-11.388734843779));
#61807=CARTESIAN_POINT('Ctrl Pts',(37.6791760082763,-1.9121371900711,-11.388584541869));
#61808=CARTESIAN_POINT('Ctrl Pts',(37.6790840265824,-1.91212724585386,-11.388509474164));
#61809=CARTESIAN_POINT('Ctrl Pts',(37.6789001608187,-1.91210736769551,-11.3883593957452));
#61810=CARTESIAN_POINT('Ctrl Pts',(37.6788082767311,-1.91209743375276,-11.3882843850383));
#61811=CARTESIAN_POINT('Ctrl Pts',(37.6786244737886,-1.91207756182977,-11.3881343125841));
#61812=CARTESIAN_POINT('Ctrl Pts',(37.6785325550223,-1.91206762385897,-11.3880592508979));
#61813=CARTESIAN_POINT('Ctrl Pts',(37.6783485518263,-1.91204772972628,-11.3879089695442));
#61814=CARTESIAN_POINT('Ctrl Pts',(37.678256467438,-1.91203777356833,-11.3878337498669));
#61815=CARTESIAN_POINT('Ctrl Pts',(37.678072002762,-1.91201782897752,-11.3876830459998));
#61816=CARTESIAN_POINT('Ctrl Pts',(37.6779796224312,-1.91200784053904,-11.3876075616987));
#61817=CARTESIAN_POINT('Ctrl Pts',(37.6777944352413,-1.91198781725927,-11.3874562216022));
#61818=CARTESIAN_POINT('Ctrl Pts',(37.6777016284151,-1.91197778242016,-11.3873803657248));
#61819=CARTESIAN_POINT('Ctrl Pts',(37.6775154567291,-1.91195765211476,-11.3872281746459));
#61820=CARTESIAN_POINT('Ctrl Pts',(37.6774220919557,-1.91194755665603,-11.3871518393728));
#61821=CARTESIAN_POINT('Ctrl Pts',(37.6772346713447,-1.91192729072041,-11.3869985802919));
#61822=CARTESIAN_POINT('Ctrl Pts',(37.6771406155851,-1.91191712024974,-11.386921656371));
#61823=CARTESIAN_POINT('Ctrl Pts',(37.6769516777556,-1.91189668965792,-11.3867671088341));
#61824=CARTESIAN_POINT('Ctrl Pts',(37.6768567957277,-1.91188642953864,-11.3866894850396));
#61825=CARTESIAN_POINT('Ctrl Pts',(37.6766660667654,-1.9118658046532,-11.3865334237115));
#61826=CARTESIAN_POINT('Ctrl Pts',(37.6765702200224,-1.91185543990459,-11.3864549860839));
#61827=CARTESIAN_POINT('Ctrl Pts',(37.6763774194694,-1.91183459037666,-11.3862971799787));
#61828=CARTESIAN_POINT('Ctrl Pts',(37.6762804658257,-1.91182410561168,-11.386217811347));
#61829=CARTESIAN_POINT('Ctrl Pts',(37.6760853047773,-1.91180300017491,-11.3860580222541));
#61830=CARTESIAN_POINT('Ctrl Pts',(37.6759870975043,-1.91179237951316,-11.3859776015683));
#61831=CARTESIAN_POINT('Ctrl Pts',(37.6757892770115,-1.91177098581065,-11.3858155827238));
#61832=CARTESIAN_POINT('Ctrl Pts',(37.6756896639658,-1.91176021278392,-11.38573398433));
#61833=CARTESIAN_POINT('Ctrl Pts',(37.6754888735132,-1.91173849720324,-11.3855694791457));
#61834=CARTESIAN_POINT('Ctrl Pts',(37.6753876963203,-1.91172755466701,-11.3854865721039));
#61835=CARTESIAN_POINT('Ctrl Pts',(37.6751836118604,-1.91170548212725,-11.3853193125284));
#61836=CARTESIAN_POINT('Ctrl Pts',(37.6750807048995,-1.9116943521507,-11.3852349597659));
#61837=CARTESIAN_POINT('Ctrl Pts',(37.674872987354,-1.91167188593989,-11.3850646650235));
#61838=CARTESIAN_POINT('Ctrl Pts',(37.6747681769798,-1.91166054972149,-11.3849787226788));
#61839=CARTESIAN_POINT('Ctrl Pts',(37.6745564695882,-1.91163765120927,-11.3848050970572));
#61840=CARTESIAN_POINT('Ctrl Pts',(37.6744495728697,-1.91162608894006,-11.3847174134254));
#61841=CARTESIAN_POINT('Ctrl Pts',(37.6742334994584,-1.91160271738989,-11.3845401448127));
#61842=CARTESIAN_POINT('Ctrl Pts',(37.6741243231037,-1.91159090813684,-11.3844505594398));
#61843=CARTESIAN_POINT('Ctrl Pts',(37.6739034856184,-1.91156702043832,-11.3842693172484));
#61844=CARTESIAN_POINT('Ctrl Pts',(37.6737918248025,-1.9115549420172,-11.3841776599426));
#61845=CARTESIAN_POINT('Ctrl Pts',(37.6735658003481,-1.91153049236507,-11.383992092622));
#61846=CARTESIAN_POINT('Ctrl Pts',(37.6734514371607,-1.91151812117205,-11.3838981821476));
#61847=CARTESIAN_POINT('Ctrl Pts',(37.6732197757027,-1.91149306081659,-11.3837079152298));
#61848=CARTESIAN_POINT('Ctrl Pts',(37.6731024778537,-1.91148037168769,-11.3836115582087));
#61849=CARTESIAN_POINT('Ctrl Pts',(37.6728646984584,-1.91145464852692,-11.3834161911434));
#61850=CARTESIAN_POINT('Ctrl Pts',(37.6727442174409,-1.91144161453875,-11.3833171805046));
#61851=CARTESIAN_POINT('Ctrl Pts',(37.6724998052689,-1.91141517279187,-11.3831162840996));
#61852=CARTESIAN_POINT('Ctrl Pts',(37.6723758746551,-1.91140176507653,-11.383014397631));
#61853=CARTESIAN_POINT('Ctrl Pts',(37.672124276753,-1.91137454482717,-11.3828075104909));
#61854=CARTESIAN_POINT('Ctrl Pts',(37.6719966100824,-1.91136073234305,-11.3827025090483));
#61855=CARTESIAN_POINT('Ctrl Pts',(37.6717372312687,-1.91133266909251,-11.3824891340739));
#61856=CARTESIAN_POINT('Ctrl Pts',(37.6716055198197,-1.91131841838221,-11.3823807596848));
#61857=CARTESIAN_POINT('Ctrl Pts',(37.6713377177761,-1.91128944251635,-11.382160359898));
#61858=CARTESIAN_POINT('Ctrl Pts',(37.6712016279954,-1.91127471742755,-11.3820483335731));
#61859=CARTESIAN_POINT('Ctrl Pts',(37.6709247080476,-1.91124475364979,-11.3818203276637));
#61860=CARTESIAN_POINT('Ctrl Pts',(37.6707838787709,-1.91122951503322,-11.3817043470239));
#61861=CARTESIAN_POINT('Ctrl Pts',(37.6704970877951,-1.91119848170252,-11.3814681041495));
#61862=CARTESIAN_POINT('Ctrl Pts',(37.670351127072,-1.91118268706699,-11.3813478407125));
#61863=CARTESIAN_POINT('Ctrl Pts',(37.6598043104844,-1.91004137149638,-11.3726557677545));
#61864=CARTESIAN_POINT('Ctrl Pts',(37.6494753144209,-1.90892164225766,-11.3639964171444));
#61865=CARTESIAN_POINT('Ctrl Pts',(37.6228578172749,-1.90602923860117,-11.3412978423569));
#61866=CARTESIAN_POINT('Ctrl Pts',(37.6066833820632,-1.90426482305452,-11.3271258444942));
#61867=CARTESIAN_POINT('Ctrl Pts',(37.5580263708135,-1.89892789937115,-11.2833254106963));
#61868=CARTESIAN_POINT('Ctrl Pts',(37.5261624223116,-1.89539244610117,-11.2530202457781));
#61869=CARTESIAN_POINT('Ctrl Pts',(37.3841109016649,-1.87933886847407,-11.1102991313864));
#61870=CARTESIAN_POINT('Ctrl Pts',(37.2842900034165,-1.86719485430491,-10.98810867134));
#61871=CARTESIAN_POINT('Ctrl Pts',(37.1450319382862,-1.8473294967471,-10.7787169325692));
#61872=CARTESIAN_POINT('Ctrl Pts',(37.0975896976733,-1.83981856266237,-10.6974193935182));
#61873=CARTESIAN_POINT('Ctrl Pts',(37.041125139902,-1.8296328697583,-10.586158143817));
#61874=CARTESIAN_POINT('Ctrl Pts',(37.0277453371089,-1.82710787684022,-10.5584925129879));
#61875=CARTESIAN_POINT('Ctrl Pts',(37.0064165061389,-1.82288552130397,-10.5121454682452));
#61876=CARTESIAN_POINT('Ctrl Pts',(36.998167129205,-1.82119848394521,-10.493605531908));
#61877=CARTESIAN_POINT('Ctrl Pts',(36.9823190822093,-1.81784636247049,-10.4567391357089));
#61878=CARTESIAN_POINT('Ctrl Pts',(36.9747106167337,-1.81618176325454,-10.4384186228191));
#61879=CARTESIAN_POINT('Ctrl Pts',(36.9567774487533,-1.81211867296545,-10.3936828127058));
#61880=CARTESIAN_POINT('Ctrl Pts',(36.9466919244674,-1.80971249992294,-10.3671756422357));
#61881=CARTESIAN_POINT('Ctrl Pts',(36.9098711324064,-1.80043818132898,-10.2650017162407));
#61882=CARTESIAN_POINT('Ctrl Pts',(36.88646303448,-1.79346564706005,-10.1882016251892));
#61883=CARTESIAN_POINT('Ctrl Pts',(36.8188134371045,-1.76896488256168,-9.91858272938146));
#61884=CARTESIAN_POINT('Ctrl Pts',(36.79453095014,-1.75095276175637,-9.72161219272226));
#61885=CARTESIAN_POINT('Ctrl Pts',(36.7946202453594,-1.73347969461058,-9.5239135539112));
#61886=CARTESIAN_POINT('Ctrl Pts',(36.7946202468458,-1.73347940418795,-9.52391026792988));
#61887=CARTESIAN_POINT('Ctrl Pts',(36.7946344625094,-1.73070610749909,-9.49253184906575));
#61888=CARTESIAN_POINT('Ctrl Pts',(36.795262680684,-1.72795021806407,-9.46115461872356));
#61889=CARTESIAN_POINT('Ctrl Pts',(36.7973688972366,-1.72331785970742,-9.40798124892672));
#61890=CARTESIAN_POINT('Ctrl Pts',(36.7985300327825,-1.72142919267939,-9.38617745568329));
#61891=CARTESIAN_POINT('Ctrl Pts',(36.8007365148464,-1.71859228728138,-9.35320547625162));
#61892=CARTESIAN_POINT('Ctrl Pts',(36.8015632918785,-1.71763362666677,-9.34202458687445));
#61893=CARTESIAN_POINT('Ctrl Pts',(36.803298813536,-1.71580295378608,-9.3205929167618));
#61894=CARTESIAN_POINT('Ctrl Pts',(36.8041952284393,-1.71493031388628,-9.31034132242188));
#61895=CARTESIAN_POINT('Ctrl Pts',(36.8062797047938,-1.71304789857974,-9.28814528731163));
#61896=CARTESIAN_POINT('Ctrl Pts',(36.807491421384,-1.71203943054874,-9.27620344206196));
#61897=CARTESIAN_POINT('Ctrl Pts',(36.8110206344547,-1.70931649849967,-9.2438362211175));
#61898=CARTESIAN_POINT('Ctrl Pts',(36.8135107129493,-1.70761107990901,-9.22343002628025));
#61899=CARTESIAN_POINT('Ctrl Pts',(36.8290603689129,-1.69803963448877,-9.10829682506911));
#61900=CARTESIAN_POINT('Ctrl Pts',(36.8474995805345,-1.6904238516734,-9.01436967149383));
#61901=CARTESIAN_POINT('Ctrl Pts',(36.8950757831786,-1.67546929328564,-8.8307195249898));
#61902=CARTESIAN_POINT('Ctrl Pts',(36.9239747888601,-1.66814404694808,-8.74116755198875));
#61903=CARTESIAN_POINT('Ctrl Pts',(36.9580197773588,-1.66076081124402,-8.65357724055094));
#61904=CARTESIAN_POINT('Ctrl Pts',(36.9580196842388,-1.39337735599387,-8.65357748012833));
#61905=CARTESIAN_POINT('Ctrl Pts',(36.9354256370871,-1.39836298839272,-8.71170704163551));
#61906=CARTESIAN_POINT('Ctrl Pts',(36.9151020359567,-1.40340071692287,-8.77069031601384));
#61907=CARTESIAN_POINT('Ctrl Pts',(36.8893389379021,-1.41071202753157,-8.85610567809243));
#61908=CARTESIAN_POINT('Ctrl Pts',(36.8820153155817,-1.41292563059602,-8.88194398141236));
#61909=CARTESIAN_POINT('Ctrl Pts',(36.8701045771221,-1.41677656756617,-8.92681660418947));
#61910=CARTESIAN_POINT('Ctrl Pts',(36.8653143095039,-1.41840728033982,-8.94579473795547));
#61911=CARTESIAN_POINT('Ctrl Pts',(36.8559311967046,-1.42177956399955,-8.98497808214362));
#61912=CARTESIAN_POINT('Ctrl Pts',(36.8513667805432,-1.42352188679338,-9.00518833288039));
#61913=CARTESIAN_POINT('Ctrl Pts',(36.8402404833912,-1.42804897583517,-9.05759488245969));
#61914=CARTESIAN_POINT('Ctrl Pts',(36.8340764540001,-1.43084593498062,-9.08987005912552));
#61915=CARTESIAN_POINT('Ctrl Pts',(36.8058539071643,-1.4453010036866,-9.25605067704835));
#61916=CARTESIAN_POINT('Ctrl Pts',(36.7944993087424,-1.45728194703566,-9.39149864706067));
#61917=CARTESIAN_POINT('Ctrl Pts',(36.7947506351827,-1.4823801582391,-9.67174675506811));
#61918=CARTESIAN_POINT('Ctrl Pts',(36.8079169078777,-1.49547128377747,-9.81603466411999));
#61919=CARTESIAN_POINT('Ctrl Pts',(36.8407188207255,-1.51148310714002,-9.99516141886595));
#61920=CARTESIAN_POINT('Ctrl Pts',(36.8483365229027,-1.51475187508347,-10.0318912923841));
#61921=CARTESIAN_POINT('Ctrl Pts',(36.8599675980825,-1.51918286360673,-10.0820426839337));
#61922=CARTESIAN_POINT('Ctrl Pts',(36.8632431253265,-1.52037981282759,-10.0956273137069));
#61923=CARTESIAN_POINT('Ctrl Pts',(36.8693283278617,-1.52251462448257,-10.1199330256061));
#61924=CARTESIAN_POINT('Ctrl Pts',(36.8720940520591,-1.5234548102879,-10.1306646499237));
#61925=CARTESIAN_POINT('Ctrl Pts',(36.8779960483429,-1.52539982215356,-10.1529278494931));
#61926=CARTESIAN_POINT('Ctrl Pts',(36.8811442408619,-1.52640397280442,-10.1644558023411));
#61927=CARTESIAN_POINT('Ctrl Pts',(36.8898764202107,-1.52910285820684,-10.1955182602469));
#61928=CARTESIAN_POINT('Ctrl Pts',(36.8956223641844,-1.53078881324802,-10.2150068743711));
#61929=CARTESIAN_POINT('Ctrl Pts',(36.9329782404033,-1.5412269056329,-10.3360325445979));
#61930=CARTESIAN_POINT('Ctrl Pts',(36.9710505007605,-1.54966505044021,-10.435468295947));
#61931=CARTESIAN_POINT('Ctrl Pts',(37.0942065879777,-1.57280177115797,-10.7026033335539));
#61932=CARTESIAN_POINT('Ctrl Pts',(37.1925163442957,-1.58731497773826,-10.8633264326893));
#61933=CARTESIAN_POINT('Ctrl Pts',(37.3331441732392,-1.60575739049916,-11.0423305949706));
#61934=CARTESIAN_POINT('Ctrl Pts',(37.3585510134031,-1.60901349930625,-11.0730659161128));
#61935=CARTESIAN_POINT('Ctrl Pts',(37.3993924418764,-1.61414428746227,-11.1200442834265));
#61936=CARTESIAN_POINT('Ctrl Pts',(37.4143108253912,-1.61599813701964,-11.1367282483374));
#61937=CARTESIAN_POINT('Ctrl Pts',(37.4424540770675,-1.61946018151433,-11.1673318225476));
#61938=CARTESIAN_POINT('Ctrl Pts',(37.4556171176741,-1.62106569745999,-11.1813060710724));
#61939=CARTESIAN_POINT('Ctrl Pts',(37.4853891562887,-1.62466795420364,-11.2121643279134));
#61940=CARTESIAN_POINT('Ctrl Pts',(37.502082858152,-1.62666823785331,-11.2289633528868));
#61941=CARTESIAN_POINT('Ctrl Pts',(37.5532685898059,-1.6327456209977,-11.2789729436592));
#61942=CARTESIAN_POINT('Ctrl Pts',(37.5885045820825,-1.63685508614768,-11.3114006400929));
#61943=CARTESIAN_POINT('Ctrl Pts',(37.651450254769,-1.64407698332831,-11.36595119996));
#61944=CARTESIAN_POINT('Ctrl Pts',(37.6787262022231,-1.64716977918694,-11.3885539734979));
#61945=CARTESIAN_POINT('Ctrl Pts',(37.8009510669318,-1.66087046116954,-11.4853663294297));
#61946=CARTESIAN_POINT('Ctrl Pts',(37.9008917329016,-1.67167630738012,-11.5529758131937));
#61947=CARTESIAN_POINT('Ctrl Pts',(38.1066492551813,-1.69298065015975,-11.6706996522756));
#61948=CARTESIAN_POINT('Ctrl Pts',(38.2119196680619,-1.7034488563966,-11.7211661802767));
#61949=CARTESIAN_POINT('Ctrl Pts',(38.3443515980746,-1.71584211478487,-11.7731944917434));
#61950=CARTESIAN_POINT('Ctrl Pts',(38.3684081827518,-1.71806305358278,-11.7822035510426));
#61951=CARTESIAN_POINT('Ctrl Pts',(38.4049063010458,-1.7213826721538,-11.79520912374));
#61952=CARTESIAN_POINT('Ctrl Pts',(38.4172426366712,-1.72249619230846,-11.7994921169922));
#61953=CARTESIAN_POINT('Ctrl Pts',(38.4399159224885,-1.72452646966998,-11.8071576210448));
#61954=CARTESIAN_POINT('Ctrl Pts',(38.450241414443,-1.72544483254174,-11.8105706696711));
#61955=CARTESIAN_POINT('Ctrl Pts',(38.4744103819586,-1.72758029826213,-11.818378201045));
#61956=CARTESIAN_POINT('Ctrl Pts',(38.4882710398223,-1.72879427442747,-11.8227175167785));
#61957=CARTESIAN_POINT('Ctrl Pts',(38.5345412352799,-1.73281406386245,-11.8367443038493));
#61958=CARTESIAN_POINT('Ctrl Pts',(38.5671176333956,-1.73559097755429,-11.8458742640354));
#61959=CARTESIAN_POINT('Ctrl Pts',(38.6489809543544,-1.74246299308248,-11.8669654306159));
#61960=CARTESIAN_POINT('Ctrl Pts',(38.6984752944038,-1.746522894857,-11.8780613726533));
#61961=CARTESIAN_POINT('Ctrl Pts',(38.9288038499066,-1.76513775701105,-11.9220988967067));
#61962=CARTESIAN_POINT('Ctrl Pts',(39.1126792892105,-1.77925943271524,-11.9358107217498));
#61963=CARTESIAN_POINT('Ctrl Pts',(39.3610149520364,-1.79910932381833,-11.9258578691793));
#61964=CARTESIAN_POINT('Ctrl Pts',(39.4255669656827,-1.80433491048928,-11.9206549194566));
#61965=CARTESIAN_POINT('Ctrl Pts',(39.5139569544387,-1.81163058072937,-11.9099265974573));
#61966=CARTESIAN_POINT('Ctrl Pts',(39.5380415866579,-1.81363284598129,-11.9066321385393));
#61967=CARTESIAN_POINT('Ctrl Pts',(39.5798244948633,-1.81713393019966,-11.9002702542273));
#61968=CARTESIAN_POINT('Ctrl Pts',(39.5975463563447,-1.81862752589069,-11.8973684969909));
#61969=CARTESIAN_POINT('Ctrl Pts',(39.6347244610432,-1.82178011856938,-11.8908527322555));
#61970=CARTESIAN_POINT('Ctrl Pts',(39.6541718153818,-1.82344032822295,-11.8871965244019));
#61971=CARTESIAN_POINT('Ctrl Pts',(39.7011274850626,-1.82747723417374,-11.8777673398156));
#61972=CARTESIAN_POINT('Ctrl Pts',(39.7285833194806,-1.82986137889642,-11.8717514657487));
#61973=CARTESIAN_POINT('Ctrl Pts',(39.8318503485237,-1.83892281442052,-11.8472204549441));
#61974=CARTESIAN_POINT('Ctrl Pts',(39.9068420736578,-1.84569830953144,-11.8255030185572));
#61975=CARTESIAN_POINT('Ctrl Pts',(40.1173958753497,-1.86530042950953,-11.7532599267183));
#61976=CARTESIAN_POINT('Ctrl Pts',(40.2496336645344,-1.87833784048335,-11.6941054946587));
#61977=CARTESIAN_POINT('Ctrl Pts',(40.4590725505517,-1.89986802355464,-11.5767584324833));
#61978=CARTESIAN_POINT('Ctrl Pts',(40.5395569030974,-1.90837720178088,-11.5251420582463));
#61979=CARTESIAN_POINT('Ctrl Pts',(40.6331192346114,-1.9184055121647,-11.4569502238248));
#61980=CARTESIAN_POINT('Ctrl Pts',(40.6493217785344,-1.92014726594701,-11.4448252194433));
#61981=CARTESIAN_POINT('Ctrl Pts',(40.6748325410936,-1.92289551425998,-11.425227432942));
#61982=CARTESIAN_POINT('Ctrl Pts',(40.6842410042701,-1.92391037378258,-11.4178877361122));
#61983=CARTESIAN_POINT('Ctrl Pts',(40.7023928297122,-1.92587027855501,-11.4035086394899));
#61984=CARTESIAN_POINT('Ctrl Pts',(40.7111421295302,-1.92681579067688,-11.3964775972933));
#61985=CARTESIAN_POINT('Ctrl Pts',(40.7329136821619,-1.92917154631027,-11.3787294847783));
#61986=CARTESIAN_POINT('Ctrl Pts',(40.7458734189018,-1.93057654161082,-11.3679359137715));
#61987=CARTESIAN_POINT('Ctrl Pts',(40.7976477931776,-1.93620573199632,-11.3238849187817));
#61988=CARTESIAN_POINT('Ctrl Pts',(40.8355148700228,-1.94036017627709,-11.2895275830551));
#61989=CARTESIAN_POINT('Ctrl Pts',(41.0211343156769,-1.96109816410334,-11.1099979059487));
#61990=CARTESIAN_POINT('Ctrl Pts',(41.1507942656646,-1.97690506165441,-10.9473795008363));
#61991=CARTESIAN_POINT('Ctrl Pts',(41.2932414433865,-1.99884887525265,-10.7119380842193));
#61992=CARTESIAN_POINT('Ctrl Pts',(41.3259712167862,-2.00433281922097,-10.6522650865879));
#61993=CARTESIAN_POINT('Ctrl Pts',(41.3683466101453,-2.01216068958093,-10.5665785765661));
#61994=CARTESIAN_POINT('Ctrl Pts',(41.3801411820427,-2.01443161730616,-10.5416598509604));
#61995=CARTESIAN_POINT('Ctrl Pts',(41.3995417128316,-2.01833358070243,-10.4987809584939));
#61996=CARTESIAN_POINT('Ctrl Pts',(41.4073624753316,-2.01995720175415,-10.4809204763705));
#61997=CARTESIAN_POINT('Ctrl Pts',(41.4229392324247,-2.02329890525174,-10.4441367132439));
#61998=CARTESIAN_POINT('Ctrl Pts',(41.4306727149896,-2.02501758605054,-10.4252057053825));
#61999=CARTESIAN_POINT('Ctrl Pts',(41.4497147799718,-2.02940715560897,-10.3768395313447));
#62000=CARTESIAN_POINT('Ctrl Pts',(41.4606872815429,-2.03208884147254,-10.3472773198119));
#62001=CARTESIAN_POINT('Ctrl Pts',(41.5106577153121,-2.04507996463358,-10.2040782653042));
#62002=CARTESIAN_POINT('Ctrl Pts',(41.5416796829331,-2.05563892933301,-10.0878615881593));
#62003=CARTESIAN_POINT('Ctrl Pts',(41.5941176475927,-2.080948976505,-9.80920087827473));
#62004=CARTESIAN_POINT('Ctrl Pts',(41.6078939154356,-2.09578973691369,-9.64590621584614));
#62005=CARTESIAN_POINT('Ctrl Pts',(41.6043494751469,-2.11341254458692,-9.44545540700976));
#62006=CARTESIAN_POINT('Ctrl Pts',(41.6028402356556,-2.11663885183464,-9.40845397303233));
#62007=CARTESIAN_POINT('Ctrl Pts',(41.5995880797562,-2.12102470331362,-9.3575960468872));
#62008=CARTESIAN_POINT('Ctrl Pts',(41.5985782165692,-2.12221802162794,-9.34370023849328));
#62009=CARTESIAN_POINT('Ctrl Pts',(41.5965492504183,-2.12434829859078,-9.31877874167206));
#62010=CARTESIAN_POINT('Ctrl Pts',(41.5955746539301,-2.12528755123094,-9.30774987464945));
#62011=CARTESIAN_POINT('Ctrl Pts',(41.5933880483643,-2.12723320957397,-9.28481289772041));
#62012=CARTESIAN_POINT('Ctrl Pts',(41.5921632596322,-2.12823891720237,-9.27290646049651));
#62013=CARTESIAN_POINT('Ctrl Pts',(41.5886100828805,-2.13094673076198,-9.24072687975029));
#62014=CARTESIAN_POINT('Ctrl Pts',(41.5861124432792,-2.13263995759401,-9.22047277969937));
#62015=CARTESIAN_POINT('Ctrl Pts',(41.5685248427174,-2.14337434136815,-9.09139570734533));
#62016=CARTESIAN_POINT('Ctrl Pts',(41.5462496757756,-2.15207996590962,-8.98366592118261));
#62017=CARTESIAN_POINT('Ctrl Pts',(41.4642866789329,-2.1760245993849,-8.69026564864504));
#62018=CARTESIAN_POINT('Ctrl Pts',(41.3893173865677,-2.19108400072141,-8.50978802863563));
#62019=CARTESIAN_POINT('Ctrl Pts',(41.2764386195138,-2.20973427371325,-8.31032128866595));
#62020=CARTESIAN_POINT('Ctrl Pts',(41.2588153264992,-2.21255997117743,-8.2806845562019));
#62021=CARTESIAN_POINT('Ctrl Pts',(41.2294156768879,-2.21714749667915,-8.23357901947776));
#62022=CARTESIAN_POINT('Ctrl Pts',(41.2180357110752,-2.21889495896355,-8.21586748230387));
#62023=CARTESIAN_POINT('Ctrl Pts',(41.1957039674352,-2.22227247162443,-8.18209402412461));
#62024=CARTESIAN_POINT('Ctrl Pts',(41.1847870216604,-2.22390113145698,-8.16601095770644));
#62025=CARTESIAN_POINT('Ctrl Pts',(41.1588293177958,-2.22772342382359,-8.12874954503866));
#62026=CARTESIAN_POINT('Ctrl Pts',(41.1436383406724,-2.22992258341988,-8.10767945891436));
#62027=CARTESIAN_POINT('Ctrl Pts',(41.0911707992034,-2.23739692539579,-8.03733637333358));
#62028=CARTESIAN_POINT('Ctrl Pts',(41.0523413229925,-2.24273056479687,-7.98925906429054));
#62029=CARTESIAN_POINT('Ctrl Pts',(40.9491417263286,-2.25644126994007,-7.87109465461216));
#62030=CARTESIAN_POINT('Ctrl Pts',(40.8823881354727,-2.26489818720462,-7.80323750689409));
#62031=CARTESIAN_POINT('Ctrl Pts',(40.6966582791728,-2.28732542619751,-7.6355745287832));
#62032=CARTESIAN_POINT('Ctrl Pts',(40.5717246510495,-2.3013741157912,-7.54300783761762));
#62033=CARTESIAN_POINT('Ctrl Pts',(40.4156489836125,-2.31725091756192,-7.44924084858929));
#62034=CARTESIAN_POINT('Ctrl Pts',(40.3923264097295,-2.31958217706309,-7.4357569738719));
#62035=CARTESIAN_POINT('Ctrl Pts',(40.3571557353439,-2.32303165796025,-7.41620402605447));
#62036=CARTESIAN_POINT('Ctrl Pts',(40.3454768364831,-2.3241664197728,-7.40983742979284));
#62037=CARTESIAN_POINT('Ctrl Pts',(40.3251334747504,-2.32612386422545,-7.39896543916571));
#62038=CARTESIAN_POINT('Ctrl Pts',(40.3164937971642,-2.32694918579274,-7.39441559640595));
#62039=CARTESIAN_POINT('Ctrl Pts',(40.2957681838185,-2.3289148945865,-7.38366173423172));
#62040=CARTESIAN_POINT('Ctrl Pts',(40.2836570399592,-2.33005225329119,-7.37750729265034));
#62041=CARTESIAN_POINT('Ctrl Pts',(40.2460296137541,-2.33355307338476,-7.35878580301019));
#62042=CARTESIAN_POINT('Ctrl Pts',(40.2203408611949,-2.33589689503679,-7.3465678479241));
#62043=CARTESIAN_POINT('Ctrl Pts',(40.1582137255434,-2.341470158285,-7.31835950666183));
#62044=CARTESIAN_POINT('Ctrl Pts',(40.1215826676185,-2.34467928882815,-7.30281152178092));
#62045=CARTESIAN_POINT('Ctrl Pts',(39.9679886953997,-2.35788810388624,-7.24207077879041));
#62046=CARTESIAN_POINT('Ctrl Pts',(39.8479625707221,-2.36763325367105,-7.20514624656529));
#62047=CARTESIAN_POINT('Ctrl Pts',(39.5984317758117,-2.38769407506172,-7.14927127095438));
#62048=CARTESIAN_POINT('Ctrl Pts',(39.4691803748756,-2.39798716371336,-7.13118100414007));
#62049=CARTESIAN_POINT('Ctrl Pts',(39.3069221817447,-2.41123768163434,-7.12178127007212));
#62050=CARTESIAN_POINT('Ctrl Pts',(39.2746995679688,-2.41388420389332,-7.12056401769166));
#62051=CARTESIAN_POINT('Ctrl Pts',(39.2218729167627,-2.41825358681938,-7.11963128956889));
#62052=CARTESIAN_POINT('Ctrl Pts',(39.2012789840869,-2.41996454602607,-7.11953219375207));
#62053=CARTESIAN_POINT('Ctrl Pts',(39.1610507722784,-2.4233230595095,-7.11985520035455));
#62054=CARTESIAN_POINT('Ctrl Pts',(39.1414178785351,-2.424969739521,-7.12025331149883));
#62055=CARTESIAN_POINT('Ctrl Pts',(39.0945670538021,-2.42891871644202,-7.12177740173451));
#62056=CARTESIAN_POINT('Ctrl Pts',(39.0673596977489,-2.43122766808379,-7.12312544414426));
#62057=CARTESIAN_POINT('Ctrl Pts',(38.9694148568078,-2.43960023071285,-7.12964748534889));
#62058=CARTESIAN_POINT('Ctrl Pts',(38.8988988122134,-2.44574341489144,-7.13748684132852));
#62059=CARTESIAN_POINT('Ctrl Pts',(38.7090014954281,-2.46261534773028,-7.16714403137755));
#62060=CARTESIAN_POINT('Ctrl Pts',(38.5907635621021,-2.47348623060971,-7.19489504817484));
#62061=CARTESIAN_POINT('Ctrl Pts',(38.3624381580267,-2.49500663398945,-7.26705569780629));
#62062=CARTESIAN_POINT('Ctrl Pts',(38.2525068895249,-2.50562488060572,-7.3109347388435));
#62063=CARTESIAN_POINT('Ctrl Pts',(38.1229257724841,-2.51818335390956,-7.37408471277485));
#62064=CARTESIAN_POINT('Ctrl Pts',(38.099797539035,-2.52042615344324,-7.38582254720096));
#62065=CARTESIAN_POINT('Ctrl Pts',(38.0652721476315,-2.52377155811467,-7.40405270471365));
#62066=CARTESIAN_POINT('Ctrl Pts',(38.0537317984729,-2.52488933430596,-7.41026740148545));
#62067=CARTESIAN_POINT('Ctrl Pts',(38.0327147843226,-2.52692343195401,-7.42180806478828));
#62068=CARTESIAN_POINT('Ctrl Pts',(38.0232229468893,-2.52784140635958,-7.42710418057828));
#62069=CARTESIAN_POINT('Ctrl Pts',(38.0011912566868,-2.52997090004405,-7.43959368388815));
#62070=CARTESIAN_POINT('Ctrl Pts',(37.98867986344,-2.53117935419479,-7.44683603498378));
#62071=CARTESIAN_POINT('Ctrl Pts',(37.9474673805177,-2.53515986955682,-7.47119097752929));
#62072=CARTESIAN_POINT('Ctrl Pts',(37.9190559102334,-2.53790379616859,-7.4887897857489));
#62073=CARTESIAN_POINT('Ctrl Pts',(37.8492145453966,-2.5446733380307,-7.53409206046493));
#62074=CARTESIAN_POINT('Ctrl Pts',(37.8082601834648,-2.54866509090709,-7.56250240611284));
#62075=CARTESIAN_POINT('Ctrl Pts',(37.6035272261156,-2.56890073061624,-7.71416243576407));
#62076=CARTESIAN_POINT('Ctrl Pts',(37.4551105380146,-2.58459463482503,-7.85670108677201));
#62077=CARTESIAN_POINT('Ctrl Pts',(37.2939689892477,-2.60525876972259,-8.0568042251627));
#62078=CARTESIAN_POINT('Ctrl Pts',(37.2627002843915,-2.60947809950996,-8.09831780018695));
#62079=CARTESIAN_POINT('Ctrl Pts',(37.2187585996923,-2.61575387748888,-8.16076723482489));
#62080=CARTESIAN_POINT('Ctrl Pts',(37.2050199784685,-2.61777034515942,-8.18093781830759));
#62081=CARTESIAN_POINT('Ctrl Pts',(37.1809979725102,-2.62139791857132,-8.21738602482849));
#62082=CARTESIAN_POINT('Ctrl Pts',(37.1705984735088,-2.62300456653339,-8.23358492580686));
#62083=CARTESIAN_POINT('Ctrl Pts',(37.1488032331037,-2.62645176634228,-8.26844800201589));
#62084=CARTESIAN_POINT('Ctrl Pts',(37.137465440381,-2.62829424585961,-8.28714612220379));
#62085=CARTESIAN_POINT('Ctrl Pts',(37.1068939142424,-2.63340311367296,-8.33915051827059));
#62086=CARTESIAN_POINT('Ctrl Pts',(37.0882025395988,-2.63668826477832,-8.37276599575652));
#62087=CARTESIAN_POINT('Ctrl Pts',(37.0630312599879,-2.64135273174106,-8.42070665348625));
#62088=CARTESIAN_POINT('Ctrl Pts',(37.0558727333429,-2.64270898144565,-8.43467095264946));
#62089=CARTESIAN_POINT('Ctrl Pts',(37.0290185542012,-2.64791282186277,-8.48834329229399));
#62090=CARTESIAN_POINT('Ctrl Pts',(37.0102863311945,-2.65178986437691,-8.5285206339614));
#62091=CARTESIAN_POINT('Ctrl Pts',(36.9805864919526,-2.6583773523619,-8.59710872023852));
#62092=CARTESIAN_POINT('Ctrl Pts',(36.9690327684355,-2.6610708467856,-8.62524320482257));
#62093=CARTESIAN_POINT('Ctrl Pts',(36.9580195936563,-2.66377399804174,-8.6535777131776));
#62094=CARTESIAN_POINT('Origin',(39.2,8.05522481984854,-9.525));
#62095=CARTESIAN_POINT('',(36.9580197210495,-4.20212274557561,-8.6535773854226));
#62096=CARTESIAN_POINT('',(36.958019684865,-3.93706097182542,-8.65357747851738));
#62097=CARTESIAN_POINT('',(36.958019684865,8.05522481984854,-8.65357747851728));
#62098=CARTESIAN_POINT('Ctrl Pts',(36.9580197210495,-4.20212274557561,-8.6535773854226));
#62099=CARTESIAN_POINT('Ctrl Pts',(36.9789532980316,-4.19708807503762,-8.5997198586879));
#62100=CARTESIAN_POINT('Ctrl Pts',(37.0018239103819,-4.19199730962815,-8.54662594563398));
#62101=CARTESIAN_POINT('Ctrl Pts',(37.0916764201578,-4.17337218780608,-8.35713803797883));
#62102=CARTESIAN_POINT('Ctrl Pts',(37.1696154487098,-4.15960777636597,-8.22636041517477));
#62103=CARTESIAN_POINT('Ctrl Pts',(37.2849661016787,-4.14223190600434,-8.06884894340515));
#62104=CARTESIAN_POINT('Ctrl Pts',(37.3115110053874,-4.13840032077303,-8.03458376386272));
#62105=CARTESIAN_POINT('Ctrl Pts',(37.3575349248862,-4.13204850734918,-7.97837977122856));
#62106=CARTESIAN_POINT('Ctrl Pts',(37.3765149164632,-4.12950594958048,-7.95604682548239));
#62107=CARTESIAN_POINT('Ctrl Pts',(37.3961206506064,-4.12696006776533,-7.93381416893564));
#62108=CARTESIAN_POINT('Ctrl Pts',(37.3963418037651,-4.12693136029805,-7.93356348938964));
#62109=CARTESIAN_POINT('Ctrl Pts',(37.396770574418,-4.12687572206829,-7.93307767730098));
#62110=CARTESIAN_POINT('Ctrl Pts',(37.3969781856565,-4.12684879090518,-7.93284253925882));
#62111=CARTESIAN_POINT('Ctrl Pts',(37.3973810455607,-4.12679654957534,-7.93238644472681));
#62112=CARTESIAN_POINT('Ctrl Pts',(37.3975762888425,-4.12677123906741,-7.93216548354789));
#62113=CARTESIAN_POINT('Ctrl Pts',(37.3979554642376,-4.12672209971508,-7.93173652127962));
#62114=CARTESIAN_POINT('Ctrl Pts',(37.3981393917136,-4.12669827057739,-7.93152851616316));
#62115=CARTESIAN_POINT('Ctrl Pts',(37.3984968794887,-4.12665196905311,-7.93112437129432));
#62116=CARTESIAN_POINT('Ctrl Pts',(37.3986704358203,-4.12662949640833,-7.93092822802543));
#62117=CARTESIAN_POINT('Ctrl Pts',(37.3990080304409,-4.12658579566507,-7.93054682376255));
#62118=CARTESIAN_POINT('Ctrl Pts',(37.3991720652657,-4.12656456734618,-7.93036155975378));
#62119=CARTESIAN_POINT('Ctrl Pts',(37.399491382033,-4.12652325427702,-7.93000102951215));
#62120=CARTESIAN_POINT('Ctrl Pts',(37.3996466609611,-4.12650316933541,-7.92982576066363));
#62121=CARTESIAN_POINT('Ctrl Pts',(37.3999491566322,-4.12646405198008,-7.92948442347234));
#62122=CARTESIAN_POINT('Ctrl Pts',(37.4000963707636,-4.12644501939719,-7.92931835283063));
#62123=CARTESIAN_POINT('Ctrl Pts',(37.4003833614409,-4.12640792452409,-7.92899469205353));
#62124=CARTESIAN_POINT('Ctrl Pts',(37.4005231357204,-4.12638986208348,-7.92883709988783));
#62125=CARTESIAN_POINT('Ctrl Pts',(37.400795812539,-4.12635463307465,-7.9285297446195));
#62126=CARTESIAN_POINT('Ctrl Pts',(37.4009287130801,-4.12633746637561,-7.92837997974711));
#62127=CARTESIAN_POINT('Ctrl Pts',(37.4011881559276,-4.12630396138085,-7.92808768858419));
#62128=CARTESIAN_POINT('Ctrl Pts',(37.4013146964558,-4.12628762297255,-7.92794516075973));
#62129=CARTESIAN_POINT('Ctrl Pts',(37.4015618860504,-4.12625571328808,-7.92766680755142));
#62130=CARTESIAN_POINT('Ctrl Pts',(37.4016825335585,-4.1262401419111,-7.92753098080234));
#62131=CARTESIAN_POINT('Ctrl Pts',(37.4019183621226,-4.12620971054969,-7.92726554208972));
#62132=CARTESIAN_POINT('Ctrl Pts',(37.402033541816,-4.12619485047391,-7.92713592890028));
#62133=CARTESIAN_POINT('Ctrl Pts',(37.4022588224155,-4.12616579091573,-7.92688247294624));
#62134=CARTESIAN_POINT('Ctrl Pts',(37.4023689220844,-4.12615159135594,-7.9267586291266));
#62135=CARTESIAN_POINT('Ctrl Pts',(37.4025843967646,-4.1261238064618,-7.92651630637436));
#62136=CARTESIAN_POINT('Ctrl Pts',(37.4026897707014,-4.12611022105525,-7.9263978264747));
#62137=CARTESIAN_POINT('Ctrl Pts',(37.4028961179395,-4.12608362207376,-7.92616586083553));
#62138=CARTESIAN_POINT('Ctrl Pts',(37.4029970902966,-4.12607060843263,-7.92605237421858));
#62139=CARTESIAN_POINT('Ctrl Pts',(37.4031949313833,-4.12604511415044,-7.92583005561599));
#62140=CARTESIAN_POINT('Ctrl Pts',(37.4032917991996,-4.12603263345914,-7.92572122292435));
#62141=CARTESIAN_POINT('Ctrl Pts',(37.4034817037152,-4.12600816947204,-7.92550790089866));
#62142=CARTESIAN_POINT('Ctrl Pts',(37.4035747397182,-4.12599618611548,-7.92540341079524));
#62143=CARTESIAN_POINT('Ctrl Pts',(37.4037572312183,-4.12597268407591,-7.92519848790906));
#62144=CARTESIAN_POINT('Ctrl Pts',(37.4038466859547,-4.12596116535579,-7.92509805458804));
#62145=CARTESIAN_POINT('Ctrl Pts',(37.4040222456106,-4.12593856248687,-7.92490098216027));
#62146=CARTESIAN_POINT('Ctrl Pts',(37.4041083498745,-4.12592747830098,-7.92480434253722));
#62147=CARTESIAN_POINT('Ctrl Pts',(37.4042774211697,-4.12590571677697,-7.92461461521679));
#62148=CARTESIAN_POINT('Ctrl Pts',(37.4043603877018,-4.12589503939356,-7.92452152695062));
#62149=CARTESIAN_POINT('Ctrl Pts',(37.404523379876,-4.12587406588367,-7.92433867871771));
#62150=CARTESIAN_POINT('Ctrl Pts',(37.4046034050206,-4.12586376972224,-7.92424891828947));
#62151=CARTESIAN_POINT('Ctrl Pts',(37.4047606960075,-4.1258435350015,-7.92407251904498));
#62152=CARTESIAN_POINT('Ctrl Pts',(37.4048379613342,-4.12583359641893,-7.9239858798844));
#62153=CARTESIAN_POINT('Ctrl Pts',(37.404989900738,-4.12581405497549,-7.92381553201053));
#62154=CARTESIAN_POINT('Ctrl Pts',(37.4050645743881,-4.12580445208829,-7.92373182293949));
#62155=CARTESIAN_POINT('Ctrl Pts',(37.4052114862019,-4.12578556176535,-7.92356715816415));
#62156=CARTESIAN_POINT('Ctrl Pts',(37.4052837240181,-4.12577627430047,-7.92348620208951));
#62157=CARTESIAN_POINT('Ctrl Pts',(37.4054259088033,-4.12575799600863,-7.92332687896706));
#62158=CARTESIAN_POINT('Ctrl Pts',(37.4054958554343,-4.12574900515794,-7.92324851160655));
#62159=CARTESIAN_POINT('Ctrl Pts',(37.4056335923282,-4.12573130261066,-7.92309421320107));
#62160=CARTESIAN_POINT('Ctrl Pts',(37.4057013822441,-4.1257225908974,-7.92301828191442));
#62161=CARTESIAN_POINT('Ctrl Pts',(37.405834930789,-4.12570543037012,-7.9228687136911));
#62162=CARTESIAN_POINT('Ctrl Pts',(37.4059006891946,-4.12569698152888,-7.92279507642928));
#62163=CARTESIAN_POINT('Ctrl Pts',(37.4060302913383,-4.12568033159704,-7.92264996396258));
#62164=CARTESIAN_POINT('Ctrl Pts',(37.4060941348202,-4.12567213048822,-7.92257848851863));
#62165=CARTESIAN_POINT('Ctrl Pts',(37.4063742785057,-4.1256361478853,-7.92226489368904));
#62166=CARTESIAN_POINT('Ctrl Pts',(37.4065906236066,-4.12560836938242,-7.92202281411367));
#62167=CARTESIAN_POINT('Ctrl Pts',(37.4070197056029,-4.12555329469829,-7.92154288796625));
#62168=CARTESIAN_POINT('Ctrl Pts',(37.4072324408335,-4.12552599840483,-7.92130503990681));
#62169=CARTESIAN_POINT('Ctrl Pts',(37.4076545540634,-4.12547185498491,-7.92083328628819));
#62170=CARTESIAN_POINT('Ctrl Pts',(37.4078639305308,-4.12544500775653,-7.92059937937601));
#62171=CARTESIAN_POINT('Ctrl Pts',(37.408279568603,-4.12539173051828,-7.92013522822932));
#62172=CARTESIAN_POINT('Ctrl Pts',(37.4084858288202,-4.12536530041351,-7.9199049827445));
#62173=CARTESIAN_POINT('Ctrl Pts',(37.4088954689702,-4.12531282656845,-7.91944788432453));
#62174=CARTESIAN_POINT('Ctrl Pts',(37.4090988476085,-4.12528678274524,-7.91922103028201));
#62175=CARTESIAN_POINT('Ctrl Pts',(37.4095029521103,-4.1252350516049,-7.91877045344044));
#62176=CARTESIAN_POINT('Ctrl Pts',(37.4097036768239,-4.12520936420876,-7.91854672960435));
#62177=CARTESIAN_POINT('Ctrl Pts',(37.4101026946897,-4.1251583169552,-7.91810215976993));
#62178=CARTESIAN_POINT('Ctrl Pts',(37.4103009867938,-4.12513295702687,-7.91788131283897));
#62179=CARTESIAN_POINT('Ctrl Pts',(37.4106953551029,-4.12508253653221,-7.91744225042664));
#62180=CARTESIAN_POINT('Ctrl Pts',(37.4108914303394,-4.12505747590474,-7.91722403412944));
#62181=CARTESIAN_POINT('Ctrl Pts',(37.411281575669,-4.12500762653886,-7.91678999284851));
#62182=CARTESIAN_POINT('Ctrl Pts',(37.4114756449382,-4.12498283773977,-7.91657416708302));
#62183=CARTESIAN_POINT('Ctrl Pts',(37.4118619849529,-4.12493350515906,-7.91614467208328));
#62184=CARTESIAN_POINT('Ctrl Pts',(37.4120542549334,-4.12490896132732,-7.91593100218758));
#62185=CARTESIAN_POINT('Ctrl Pts',(37.4124371995275,-4.12486009232179,-7.91550558871456));
#62186=CARTESIAN_POINT('Ctrl Pts',(37.4126278734531,-4.12483576710535,-7.91529384456808));
#62187=CARTESIAN_POINT('Ctrl Pts',(37.4130078262841,-4.12478730939674,-7.91487205619463));
#62188=CARTESIAN_POINT('Ctrl Pts',(37.413197104596,-4.1247631768665,-7.91466201146434));
#62189=CARTESIAN_POINT('Ctrl Pts',(37.4135744644207,-4.12471507893278,-7.91424339855288));
#62190=CARTESIAN_POINT('Ctrl Pts',(37.4137625454601,-4.12469111349204,-7.91403482990027));
#62191=CARTESIAN_POINT('Ctrl Pts',(37.4141377076009,-4.12464332437634,-7.9136189479316));
#62192=CARTESIAN_POINT('Ctrl Pts',(37.4143247882613,-4.12461950067569,-7.91341163426885));
#62193=CARTESIAN_POINT('Ctrl Pts',(37.4146981457748,-4.12457196983409,-7.91299804251065));
#62194=CARTESIAN_POINT('Ctrl Pts',(37.4148844223006,-4.12454826266832,-7.91279176409969));
#62195=CARTESIAN_POINT('Ctrl Pts',(37.4152563676823,-4.12450093975039,-7.9123800236916));
#62196=CARTESIAN_POINT('Ctrl Pts',(37.4154420362939,-4.12447732397798,-7.91217456144169));
#62197=CARTESIAN_POINT('Ctrl Pts',(37.4232564042349,-4.12348368463005,-7.90353012589604));
#62198=CARTESIAN_POINT('Ctrl Pts',(37.4309451422223,-4.12251783323578,-7.89514500987252));
#62199=CARTESIAN_POINT('Ctrl Pts',(37.4456939952901,-4.12068791537491,-7.87928767812337));
#62200=CARTESIAN_POINT('Ctrl Pts',(37.4527429698742,-4.11982301981645,-7.87180567157449));
#62201=CARTESIAN_POINT('Ctrl Pts',(37.4721094199341,-4.11747224703073,-7.85151174655619));
#62202=CARTESIAN_POINT('Ctrl Pts',(37.4845216177477,-4.11599329814897,-7.83879041372696));
#62203=CARTESIAN_POINT('Ctrl Pts',(37.5360401854048,-4.10996089118094,-7.78714650611917));
#62204=CARTESIAN_POINT('Ctrl Pts',(37.5763427167114,-4.10548819150956,-7.74943379609983));
#62205=CARTESIAN_POINT('Ctrl Pts',(37.7273906266859,-4.08942938825138,-7.61754123706096));
#62206=CARTESIAN_POINT('Ctrl Pts',(37.8453168031938,-4.0781803242236,-7.53205818744956));
#62207=CARTESIAN_POINT('Ctrl Pts',(38.0694773198436,-4.0576705845938,-7.39871157345516));
#62208=CARTESIAN_POINT('Ctrl Pts',(38.1728153415629,-4.04850673717436,-7.34691141991696));
#62209=CARTESIAN_POINT('Ctrl Pts',(38.3083603316237,-4.03653548916244,-7.29076410946533));
#62210=CARTESIAN_POINT('Ctrl Pts',(38.3374873760493,-4.03396641541602,-7.27935908827136));
#62211=CARTESIAN_POINT('Ctrl Pts',(38.3859662548256,-4.02969071972083,-7.2614589136261));
#62212=CARTESIAN_POINT('Ctrl Pts',(38.4051938102531,-4.02799498496983,-7.25463609629372));
#62213=CARTESIAN_POINT('Ctrl Pts',(38.4429969215956,-4.0246597396339,-7.24176087722895));
#62214=CARTESIAN_POINT('Ctrl Pts',(38.4615640599161,-4.02302102643937,-7.23568856055004));
#62215=CARTESIAN_POINT('Ctrl Pts',(38.5066943711579,-4.01903516255755,-7.22153498079274));
#62216=CARTESIAN_POINT('Ctrl Pts',(38.533326840471,-4.01668073174756,-7.21368640179291));
#62217=CARTESIAN_POINT('Ctrl Pts',(38.6269740611915,-4.00839000467793,-7.1878417468308));
#62218=CARTESIAN_POINT('Ctrl Pts',(38.6946198085465,-4.00237884242127,-7.17228746770328));
#62219=CARTESIAN_POINT('Ctrl Pts',(38.9370248085948,-3.98074145434473,-7.12748564819134));
#62220=CARTESIAN_POINT('Ctrl Pts',(39.1142241427494,-3.96469829245018,-7.11463501322177));
#62221=CARTESIAN_POINT('Ctrl Pts',(39.3419571608479,-3.94434636171703,-7.12327529256033));
#62222=CARTESIAN_POINT('Ctrl Pts',(39.3926488281336,-3.93983766250709,-7.12680889811879));
#62223=CARTESIAN_POINT('Ctrl Pts',(39.4768897713274,-3.93241398179583,-7.13536987425918));
#62224=CARTESIAN_POINT('Ctrl Pts',(39.5105121545372,-3.92946956844607,-7.13950578936547));
#62225=CARTESIAN_POINT('Ctrl Pts',(39.5584214068598,-3.92531009738881,-7.14642937226976));
#62226=CARTESIAN_POINT('Ctrl Pts',(39.572785858242,-3.9240676465764,-7.14863831186475));
#62227=CARTESIAN_POINT('Ctrl Pts',(39.5978661219795,-3.92190747460796,-7.15272813032605));
#62228=CARTESIAN_POINT('Ctrl Pts',(39.6085904291999,-3.92098677119622,-7.15455169739799));
#62229=CARTESIAN_POINT('Ctrl Pts',(39.6321604145059,-3.91896992730147,-7.15872427187156));
#62230=CARTESIAN_POINT('Ctrl Pts',(39.6449998090439,-3.91787554289805,-7.16110519697268));
#62231=CARTESIAN_POINT('Ctrl Pts',(39.6830238145486,-3.91464539556117,-7.16847712354815));
#62232=CARTESIAN_POINT('Ctrl Pts',(39.7081496906942,-3.91252515076306,-7.17376710518071));
#62233=CARTESIAN_POINT('Ctrl Pts',(39.8476157956945,-3.90081039849542,-7.20547048767433));
#62234=CARTESIAN_POINT('Ctrl Pts',(39.9600043482237,-3.89156929710719,-7.23982501214804));
#62235=CARTESIAN_POINT('Ctrl Pts',(40.1821008901161,-3.87288869501962,-7.32592555854827));
#62236=CARTESIAN_POINT('Ctrl Pts',(40.2912961120957,-3.86347518291296,-7.37802043881677));
#62237=CARTESIAN_POINT('Ctrl Pts',(40.4587820104216,-3.84809993948118,-7.4740152401336));
#62238=CARTESIAN_POINT('Ctrl Pts',(40.5197957522134,-3.84228277520531,-7.51273561472188));
#62239=CARTESIAN_POINT('Ctrl Pts',(40.601429497215,-3.83412274406667,-7.5698530321968));
#62240=CARTESIAN_POINT('Ctrl Pts',(40.623617538979,-3.83186446423351,-7.58594938708644));
#62241=CARTESIAN_POINT('Ctrl Pts',(40.6612462270892,-3.82796089790422,-7.61424117298881));
#62242=CARTESIAN_POINT('Ctrl Pts',(40.6768215897679,-3.82632273607092,-7.62625363069703));
#62243=CARTESIAN_POINT('Ctrl Pts',(40.7083639971057,-3.82295772860053,-7.65120351795884));
#62244=CARTESIAN_POINT('Ctrl Pts',(40.7243160120375,-3.82123033818843,-7.66415722232842));
#62245=CARTESIAN_POINT('Ctrl Pts',(40.7646849044199,-3.81679129434476,-7.69780584585513));
#62246=CARTESIAN_POINT('Ctrl Pts',(40.7888574283734,-3.81406835349167,-7.71878595194835));
#62247=CARTESIAN_POINT('Ctrl Pts',(40.902561207357,-3.80093673596931,-7.82152198169018));
#62248=CARTESIAN_POINT('Ctrl Pts',(40.9862292686534,-3.7902744661659,-7.90947304005815));
#62249=CARTESIAN_POINT('Ctrl Pts',(41.1360785131185,-3.76912174865601,-8.09292674472192));
#62250=CARTESIAN_POINT('Ctrl Pts',(41.2026961828504,-3.75867414896264,-8.18767392563903));
#62251=CARTESIAN_POINT('Ctrl Pts',(41.2884630035128,-3.74379354084922,-8.33052483261265));
#62252=CARTESIAN_POINT('Ctrl Pts',(41.3132956997025,-3.73927123387884,-8.37503014862045));
#62253=CARTESIAN_POINT('Ctrl Pts',(41.3522846385682,-3.73182795137076,-8.45044165359566));
#62254=CARTESIAN_POINT('Ctrl Pts',(41.3672330422283,-3.72887736385733,-8.48091854167637));
#62255=CARTESIAN_POINT('Ctrl Pts',(41.3876592106449,-3.72471084396812,-8.52489418294807));
#62256=CARTESIAN_POINT('Ctrl Pts',(41.3936664613343,-3.72346739723268,-8.53814035615214));
#62257=CARTESIAN_POINT('Ctrl Pts',(41.4039565948475,-3.72130614328152,-8.56138875891427));
#62258=CARTESIAN_POINT('Ctrl Pts',(41.4082922898067,-3.72038534344726,-8.57136669613979));
#62259=CARTESIAN_POINT('Ctrl Pts',(41.4176797458634,-3.71836906705837,-8.59337787694358));
#62260=CARTESIAN_POINT('Ctrl Pts',(41.4227014780813,-3.71727533869861,-8.6054232500178));
#62261=CARTESIAN_POINT('Ctrl Pts',(41.4372956597136,-3.71404921102,-8.64124771232734));
#62262=CARTESIAN_POINT('Ctrl Pts',(41.446586738446,-3.71193227226104,-8.66514061495986));
#62263=CARTESIAN_POINT('Ctrl Pts',(41.4970891370262,-3.70002740262558,-8.80142323874056));
#62264=CARTESIAN_POINT('Ctrl Pts',(41.5302531445201,-3.69060819809469,-8.91663295014179));
#62265=CARTESIAN_POINT('Ctrl Pts',(41.5795598851495,-3.6716749720438,-9.15302170123694));
#62266=CARTESIAN_POINT('Ctrl Pts',(41.5953331973741,-3.66218667001029,-9.27390318868021));
#62267=CARTESIAN_POINT('Ctrl Pts',(41.6056477328739,-3.64691727851862,-9.46514441927643));
#62268=CARTESIAN_POINT('Ctrl Pts',(41.6063713049834,-3.6412916789275,-9.5349577772375));
#62269=CARTESIAN_POINT('Ctrl Pts',(41.603161503988,-3.63335473955565,-9.63177995159698));
#62270=CARTESIAN_POINT('Ctrl Pts',(41.6018061915692,-3.63112173070182,-9.65884345281451));
#62271=CARTESIAN_POINT('Ctrl Pts',(41.5986820619398,-3.62724781452777,-9.70544976210793));
#62272=CARTESIAN_POINT('Ctrl Pts',(41.5971307299884,-3.62561374461683,-9.72500491589962));
#62273=CARTESIAN_POINT('Ctrl Pts',(41.5934560399586,-3.62224438149663,-9.7650987547253));
#62274=CARTESIAN_POINT('Ctrl Pts',(41.5913070512718,-3.62050842646071,-9.78563337631017));
#62275=CARTESIAN_POINT('Ctrl Pts',(41.5850971754671,-3.61601959108896,-9.83840028087918));
#62276=CARTESIAN_POINT('Ctrl Pts',(41.5806472896948,-3.61325491722198,-9.87058144189002));
#62277=CARTESIAN_POINT('Ctrl Pts',(41.5546636602376,-3.59906743619407,-10.0340225821006));
#62278=CARTESIAN_POINT('Ctrl Pts',(41.5229243160786,-3.58733485692584,-10.1634004617121));
#62279=CARTESIAN_POINT('Ctrl Pts',(41.4397342668789,-3.5639057257455,-10.4115834273111));
#62280=CARTESIAN_POINT('Ctrl Pts',(41.38906134793,-3.55225883200327,-10.530212122753));
#62281=CARTESIAN_POINT('Ctrl Pts',(41.3044020437448,-3.53613381855175,-10.6912633289709));
#62282=CARTESIAN_POINT('Ctrl Pts',(41.2781152029641,-3.5314689899327,-10.7374835902885));
#62283=CARTESIAN_POINT('Ctrl Pts',(41.241380125343,-3.52540818747297,-10.7973647791941));
#62284=CARTESIAN_POINT('Ctrl Pts',(41.232289214171,-3.52394220675367,-10.811835478693));
#62285=CARTESIAN_POINT('Ctrl Pts',(41.2169484883616,-3.52152518065634,-10.8356863570752));
#62286=CARTESIAN_POINT('Ctrl Pts',(41.2107857371713,-3.52056883923298,-10.8451214614957));
#62287=CARTESIAN_POINT('Ctrl Pts',(41.1979975565682,-3.51861459285457,-10.8644026759656));
#62288=CARTESIAN_POINT('Ctrl Pts',(41.1913651909022,-3.51761715534665,-10.874243662093));
#62289=CARTESIAN_POINT('Ctrl Pts',(41.1734040759166,-3.51495744543523,-10.9004730781691));
#62290=CARTESIAN_POINT('Ctrl Pts',(41.1619437664537,-3.51330351901142,-10.9167710200746));
#62291=CARTESIAN_POINT('Ctrl Pts',(41.0992797668646,-3.50447627766161,-11.003574229932));
#62292=CARTESIAN_POINT('Ctrl Pts',(41.0444692965066,-3.49751093621642,-11.0714095880769));
#62293=CARTESIAN_POINT('Ctrl Pts',(40.8846771709227,-3.47865809106085,-11.2485544594732));
#62294=CARTESIAN_POINT('Ctrl Pts',(40.7728772744397,-3.46695311311918,-11.3511530322382));
#62295=CARTESIAN_POINT('Ctrl Pts',(40.5886163438648,-3.44859799728784,-11.4906942505506));
#62296=CARTESIAN_POINT('Ctrl Pts',(40.5227118546039,-3.44219487720637,-11.5356317897003));
#62297=CARTESIAN_POINT('Ctrl Pts',(40.4305574262115,-3.43335649572197,-11.5919742074555));
#62298=CARTESIAN_POINT('Ctrl Pts',(40.4061531640495,-3.43102656147433,-11.6063092902611));
#62299=CARTESIAN_POINT('Ctrl Pts',(40.3642324192192,-3.42703826180018,-11.6299486750692));
#62300=CARTESIAN_POINT('Ctrl Pts',(40.3468429684908,-3.42538784940246,-11.6394732693829));
#62301=CARTESIAN_POINT('Ctrl Pts',(40.3135084569087,-3.42223043731733,-11.6571991702451));
#62302=CARTESIAN_POINT('Ctrl Pts',(40.2975854649628,-3.42072492796014,-11.6654393229157));
#62303=CARTESIAN_POINT('Ctrl Pts',(40.2599826738543,-3.41717497124717,-11.6843688683312));
#62304=CARTESIAN_POINT('Ctrl Pts',(40.2382313287017,-3.41512561719827,-11.6949107803947));
#62305=CARTESIAN_POINT('Ctrl Pts',(40.1586343863733,-3.40763832580429,-11.7320171384849));
#62306=CARTESIAN_POINT('Ctrl Pts',(40.0999044484281,-3.40213595380182,-11.7566081498705));
#62307=CARTESIAN_POINT('Ctrl Pts',(39.8395409974984,-3.37781560464478,-11.8536765858123));
#62308=CARTESIAN_POINT('Ctrl Pts',(39.6297153904147,-3.35828807712093,-11.9013562233397));
#62309=CARTESIAN_POINT('Ctrl Pts',(39.3662266600683,-3.33487102026445,-11.9251584059604));
#62310=CARTESIAN_POINT('Ctrl Pts',(39.315910056715,-3.33045426489502,-11.92811413104));
#62311=CARTESIAN_POINT('Ctrl Pts',(39.2487535190368,-3.32466078183622,-11.9299444488401));
#62312=CARTESIAN_POINT('Ctrl Pts',(39.2319688775182,-3.32322125668894,-11.9302261323537));
#62313=CARTESIAN_POINT('Ctrl Pts',(39.203971489103,-3.3208355938826,-11.9304028458654));
#62314=CARTESIAN_POINT('Ctrl Pts',(39.192760209582,-3.31988443656194,-11.9303952341023));
#62315=CARTESIAN_POINT('Ctrl Pts',(39.1695866833123,-3.31792748318182,-11.9302174695783));
#62316=CARTESIAN_POINT('Ctrl Pts',(39.1576249854969,-3.31692227211632,-11.9300364702339));
#62317=CARTESIAN_POINT('Ctrl Pts',(39.1253015719838,-3.31421802620232,-11.929306128465));
#62318=CARTESIAN_POINT('Ctrl Pts',(39.1049440355746,-3.31252782769893,-11.9285873736268));
#62319=CARTESIAN_POINT('Ctrl Pts',(38.9821664579536,-3.30239865618982,-11.9226900813933));
#62320=CARTESIAN_POINT('Ctrl Pts',(38.8801392831532,-3.29425047794686,-11.9112239274528));
#62321=CARTESIAN_POINT('Ctrl Pts',(38.642176440827,-3.27522646572246,-11.8689363942833));
#62322=CARTESIAN_POINT('Ctrl Pts',(38.5075848497028,-3.26443893238458,-11.832761937829));
#62323=CARTESIAN_POINT('Ctrl Pts',(38.3281371996946,-3.24925494190907,-11.7674091258753));
#62324=CARTESIAN_POINT('Ctrl Pts',(38.2799888757992,-3.24509938972881,-11.7480884658683));
#62325=CARTESIAN_POINT('Ctrl Pts',(38.195365669695,-3.23761217076366,-11.7109113409418));
#62326=CARTESIAN_POINT('Ctrl Pts',(38.1586469364684,-3.23429958007016,-11.6936590199096));
#62327=CARTESIAN_POINT('Ctrl Pts',(38.1024537088755,-3.22911822697883,-11.6655004186826));
#62328=CARTESIAN_POINT('Ctrl Pts',(38.0826639351457,-3.22727144536265,-11.655237064939));
#62329=CARTESIAN_POINT('Ctrl Pts',(38.0460929002093,-3.22381542298499,-11.6356208393992));
#62330=CARTESIAN_POINT('Ctrl Pts',(38.0292753689502,-3.22220877718984,-11.6263390291594));
#62331=CARTESIAN_POINT('Ctrl Pts',(37.9918657211441,-3.21859455072907,-11.6051036926888));
#62332=CARTESIAN_POINT('Ctrl Pts',(37.9713366046455,-3.21658332158825,-11.5930439989078));
#62333=CARTESIAN_POINT('Ctrl Pts',(37.9188063603266,-3.21136233349886,-11.5611272115355));
#62334=CARTESIAN_POINT('Ctrl Pts',(37.8870877743804,-3.20813676855155,-11.5408205056273));
#62335=CARTESIAN_POINT('Ctrl Pts',(37.7015898215468,-3.1888214035706,-11.4158266596755));
#62336=CARTESIAN_POINT('Ctrl Pts',(37.5599258705225,-3.17211393290507,-11.2943469481661));
#62337=CARTESIAN_POINT('Ctrl Pts',(37.3619322857455,-3.14592592451253,-11.0801647532617));
#62338=CARTESIAN_POINT('Ctrl Pts',(37.2953531773402,-3.1364814058271,-10.99787355272));
#62339=CARTESIAN_POINT('Ctrl Pts',(37.2226968545233,-3.12556214046695,-10.8948676548096));
#62340=CARTESIAN_POINT('Ctrl Pts',(37.2112046415306,-3.12381451709613,-10.8781290502756));
#62341=CARTESIAN_POINT('Ctrl Pts',(37.1932876076326,-3.12105905805202,-10.8513110799374));
#62342=CARTESIAN_POINT('Ctrl Pts',(37.1867239308571,-3.12004278821597,-10.8413264014068));
#62343=CARTESIAN_POINT('Ctrl Pts',(37.1742136133922,-3.11809304228882,-10.8219831859109));
#62344=CARTESIAN_POINT('Ctrl Pts',(37.1682568693557,-3.11715898007068,-10.8126318296403));
#62345=CARTESIAN_POINT('Ctrl Pts',(37.1534816677931,-3.11482682043273,-10.7890787537873));
#62346=CARTESIAN_POINT('Ctrl Pts',(37.1447459419464,-3.113433911843,-10.7748252619129));
#62347=CARTESIAN_POINT('Ctrl Pts',(37.1124406828129,-3.10822440847756,-10.7208601254948));
#62348=CARTESIAN_POINT('Ctrl Pts',(37.089865838044,-3.10446340398562,-10.6805604532745));
#62349=CARTESIAN_POINT('Ctrl Pts',(37.0047867861053,-3.08968072914683,-10.5178618188161));
#62350=CARTESIAN_POINT('Ctrl Pts',(36.9516559067394,-3.07900914396076,-10.3908474136524));
#62351=CARTESIAN_POINT('Ctrl Pts',(36.8825491351842,-3.06127033496665,-10.1754973039318));
#62352=CARTESIAN_POINT('Ctrl Pts',(36.8601353947718,-3.05428303189767,-10.089585621727));
#62353=CARTESIAN_POINT('Ctrl Pts',(36.8307823746546,-3.042438842247,-9.94470751144883));
#62354=CARTESIAN_POINT('Ctrl Pts',(36.8211857251668,-3.03765424644014,-9.88636977665981));
#62355=CARTESIAN_POINT('Ctrl Pts',(36.8105290415511,-3.03070536141989,-9.80237242937044));
#62356=CARTESIAN_POINT('Ctrl Pts',(36.8077153209344,-3.02859489614765,-9.77695403948363));
#62357=CARTESIAN_POINT('Ctrl Pts',(36.803482019121,-3.02486238548882,-9.73219638518592));
#62358=CARTESIAN_POINT('Ctrl Pts',(36.8018900041445,-3.02324581532336,-9.71287542717288));
#62359=CARTESIAN_POINT('Ctrl Pts',(36.7990436704656,-3.01984290016081,-9.67235227839468));
#62360=CARTESIAN_POINT('Ctrl Pts',(36.7978362967326,-3.01805524697543,-9.65114860662235));
#62361=CARTESIAN_POINT('Ctrl Pts',(36.7953671146356,-3.01326727402373,-9.59460110868981));
#62362=CARTESIAN_POINT('Ctrl Pts',(36.7946038128975,-3.01025195933057,-9.55924216341062));
#62363=CARTESIAN_POINT('Ctrl Pts',(36.7946876540845,-2.99476145035167,-9.37898726240768));
#62364=CARTESIAN_POINT('Ctrl Pts',(36.8078466843381,-2.9819201258553,-9.23442382642469));
#62365=CARTESIAN_POINT('Ctrl Pts',(36.8612781675293,-2.95529196437138,-8.94248823477183));
#62366=CARTESIAN_POINT('Ctrl Pts',(36.9027354158672,-2.94154878406301,-8.79594354544676));
#62367=CARTESIAN_POINT('Ctrl Pts',(36.9578377979202,-2.92831315340977,-8.65404554251884));
#62368=CARTESIAN_POINT('Ctrl Pts',(36.9579287230691,-2.92829132352758,-8.65381150340287));
#62369=CARTESIAN_POINT('Ctrl Pts',(36.9580196848651,-2.92826949524753,-8.65357747851701));
#62370=CARTESIAN_POINT('',(36.7946197192388,-2.74169975326257,-9.52385327436721));
#62371=CARTESIAN_POINT('Ctrl Pts',(36.9580195936563,-2.66377399804174,-8.6535777131776));
#62372=CARTESIAN_POINT('Ctrl Pts',(36.9106737021466,-2.67539490742279,-8.77538841585373));
#62373=CARTESIAN_POINT('Ctrl Pts',(36.8733187052698,-2.68721056326922,-8.90089459411834));
#62374=CARTESIAN_POINT('Ctrl Pts',(36.8303325329871,-2.70583740325456,-9.1048144841857));
#62375=CARTESIAN_POINT('Ctrl Pts',(36.8180044735395,-2.71271559683368,-9.18151787871706));
#62376=CARTESIAN_POINT('Ctrl Pts',(36.807248568324,-2.72112334906031,-9.27807134423992));
#62377=CARTESIAN_POINT('Ctrl Pts',(36.8053253359953,-2.7228005750893,-9.29747746650217));
#62378=CARTESIAN_POINT('Ctrl Pts',(36.8026196285361,-2.72547115943757,-9.32863572539961));
#62379=CARTESIAN_POINT('Ctrl Pts',(36.8016871328292,-2.72647212326772,-9.34037339463035));
#62380=CARTESIAN_POINT('Ctrl Pts',(36.8001093748583,-2.72832928820449,-9.36226861014263));
#62381=CARTESIAN_POINT('Ctrl Pts',(36.7994423303061,-2.72918664107325,-9.37242411577258));
#62382=CARTESIAN_POINT('Ctrl Pts',(36.7981671699529,-2.73099370122103,-9.39392352102553));
#62383=CARTESIAN_POINT('Ctrl Pts',(36.7975749109306,-2.73194255546792,-9.40526824213702));
#62384=CARTESIAN_POINT('Ctrl Pts',(36.7963438206684,-2.73421507975633,-9.43256250741328));
#62385=CARTESIAN_POINT('Ctrl Pts',(36.7957833186636,-2.73553484179597,-9.44851531670021));
#62386=CARTESIAN_POINT('Ctrl Pts',(36.7948835136303,-2.73847568131273,-9.48426287400214));
#62387=CARTESIAN_POINT('Ctrl Pts',(36.7946296861135,-2.74009288458285,-9.50405873585586));
#62388=CARTESIAN_POINT('Ctrl Pts',(36.7946202719557,-2.74170095028303,-9.52385618472513));
#62389=CARTESIAN_POINT('Ctrl Pts',(36.7946202733782,-2.74170070761246,-9.52385319712528));
#62390=CARTESIAN_POINT('Ctrl Pts',(36.7945125912583,-2.76004636507561,-9.74971275308896));
#62391=CARTESIAN_POINT('Ctrl Pts',(36.8262150259338,-2.77719279965518,-9.97450095176669));
#62392=CARTESIAN_POINT('Ctrl Pts',(36.9086202717484,-2.80088393047634,-10.2602076959855));
#62393=CARTESIAN_POINT('Ctrl Pts',(36.9314513592635,-2.80663604223582,-10.327892697815));
#62394=CARTESIAN_POINT('Ctrl Pts',(36.9671251313568,-2.81472008084598,-10.4199123671693));
#62395=CARTESIAN_POINT('Ctrl Pts',(36.9774259244323,-2.81696956957016,-10.4451970872159));
#62396=CARTESIAN_POINT('Ctrl Pts',(36.9958756686948,-2.82086250300826,-10.4883664363795));
#62397=CARTESIAN_POINT('Ctrl Pts',(37.0038177320463,-2.82249892060106,-10.5063370248979));
#62398=CARTESIAN_POINT('Ctrl Pts',(37.0205257432503,-2.82586444395748,-10.5429234929812));
#62399=CARTESIAN_POINT('Ctrl Pts',(37.0293121810437,-2.82759413184188,-10.5615281519121));
#62400=CARTESIAN_POINT('Ctrl Pts',(37.0524373007287,-2.8320478809966,-10.6089100720238));
#62401=CARTESIAN_POINT('Ctrl Pts',(37.067115781493,-2.83478338386549,-10.6375157469185));
#62402=CARTESIAN_POINT('Ctrl Pts',(37.1430241382827,-2.84850018615683,-10.7784203447903));
#62403=CARTESIAN_POINT('Ctrl Pts',(37.2125589543476,-2.85976644912611,-10.8859846288075));
#62404=CARTESIAN_POINT('Ctrl Pts',(37.3677845594014,-2.88259505763972,-11.08867539929));
#62405=CARTESIAN_POINT('Ctrl Pts',(37.4531878349822,-2.89411994025935,-11.1835360473055));
#62406=CARTESIAN_POINT('Ctrl Pts',(37.5748101924931,-2.90900413707591,-11.2987582923131));
#62407=CARTESIAN_POINT('Ctrl Pts',(37.6046024864356,-2.91254260614131,-11.3256020068992));
#62408=CARTESIAN_POINT('Ctrl Pts',(37.650423930098,-2.91781138372669,-11.3648577600313));
#62409=CARTESIAN_POINT('Ctrl Pts',(37.6659603131952,-2.91956907524939,-11.377831586249));
#62410=CARTESIAN_POINT('Ctrl Pts',(37.6938765430166,-2.92267420502874,-11.4005514397745));
#62411=CARTESIAN_POINT('Ctrl Pts',(37.7061916685781,-2.92402610656255,-11.4103747055352));
#62412=CARTESIAN_POINT('Ctrl Pts',(37.7187457928655,-2.92538555859961,-11.4201883682473));
#62413=CARTESIAN_POINT('Ctrl Pts',(37.7188886944257,-2.92540103059182,-11.4203000495419));
#62414=CARTESIAN_POINT('Ctrl Pts',(37.7191742267598,-2.92543194040184,-11.4205231484909));
#62415=CARTESIAN_POINT('Ctrl Pts',(37.7193168574513,-2.92544737822079,-11.4206345661887));
#62416=CARTESIAN_POINT('Ctrl Pts',(37.7196021645189,-2.92547825396057,-11.4208573854247));
#62417=CARTESIAN_POINT('Ctrl Pts',(37.7197448409393,-2.92549369188551,-11.4209687869902));
#62418=CARTESIAN_POINT('Ctrl Pts',(37.7200305625532,-2.92552460278646,-11.4211918261474));
#62419=CARTESIAN_POINT('Ctrl Pts',(37.7201736077866,-2.92554007575513,-11.4213034636454));
#62420=CARTESIAN_POINT('Ctrl Pts',(37.7204603997792,-2.92557109269399,-11.421527233924));
#62421=CARTESIAN_POINT('Ctrl Pts',(37.7206041466505,-2.92558663665323,-11.4216393665453));
#62422=CARTESIAN_POINT('Ctrl Pts',(37.7208926876854,-2.92561783288506,-11.4218643959884));
#62423=CARTESIAN_POINT('Ctrl Pts',(37.7210374820546,-2.92563348514481,-11.4219772925957));
#62424=CARTESIAN_POINT('Ctrl Pts',(37.7213284807267,-2.92566493706534,-11.4222041315706));
#62425=CARTESIAN_POINT('Ctrl Pts',(37.7214746852202,-2.92568073669882,-11.4223180735748));
#62426=CARTESIAN_POINT('Ctrl Pts',(37.7217688877519,-2.92571252466894,-11.4225473006952));
#62427=CARTESIAN_POINT('Ctrl Pts',(37.7219168861233,-2.92572851297974,-11.4226625854104));
#62428=CARTESIAN_POINT('Ctrl Pts',(37.7222150858603,-2.925760722342,-11.422894814835));
#62429=CARTESIAN_POINT('Ctrl Pts',(37.7223652876605,-2.92577694336323,-11.4230117590589));
#62430=CARTESIAN_POINT('Ctrl Pts',(37.7311257906304,-2.92672287608498,-11.429830847469));
#62431=CARTESIAN_POINT('Ctrl Pts',(37.7397819318189,-2.92764871883772,-11.4364746177967));
#62432=CARTESIAN_POINT('Ctrl Pts',(37.7567689312453,-2.92944804862587,-11.4493297514159));
#62433=CARTESIAN_POINT('Ctrl Pts',(37.7650952612827,-2.93032193515376,-11.4555463769337));
#62434=CARTESIAN_POINT('Ctrl Pts',(37.7882492186177,-2.93273065242486,-11.4726010829805));
#62435=CARTESIAN_POINT('Ctrl Pts',(37.8031615332257,-2.93425795194307,-11.4833239283069));
#62436=CARTESIAN_POINT('Ctrl Pts',(37.868586402283,-2.9408621797548,-11.5292406743148));
#62437=CARTESIAN_POINT('Ctrl Pts',(37.9203218509282,-2.94583762920622,-11.5626624850716));
#62438=CARTESIAN_POINT('Ctrl Pts',(38.1065169523827,-2.96311522128256,-11.6730541846325));
#62439=CARTESIAN_POINT('Ctrl Pts',(38.2470692183789,-2.97507219921551,-11.7389942489519));
#62440=CARTESIAN_POINT('Ctrl Pts',(38.4876521710619,-2.99522155030195,-11.8246761388048));
#62441=CARTESIAN_POINT('Ctrl Pts',(38.5843186943765,-3.00323510386928,-11.8524196137286));
#62442=CARTESIAN_POINT('Ctrl Pts',(38.7119768916635,-3.01391124669849,-11.880547061124));
#62443=CARTESIAN_POINT('Ctrl Pts',(38.7416452834822,-3.0163983692474,-11.8864993753687));
#62444=CARTESIAN_POINT('Ctrl Pts',(38.791289166463,-3.02057471908716,-11.8954886121179));
#62445=CARTESIAN_POINT('Ctrl Pts',(38.8112054589267,-3.02225409348217,-11.8988364641464));
#62446=CARTESIAN_POINT('Ctrl Pts',(38.850601760986,-3.02558510999255,-11.9049497603531));
#62447=CARTESIAN_POINT('Ctrl Pts',(38.8700782442013,-3.02723622045584,-11.9077277597645));
#62448=CARTESIAN_POINT('Ctrl Pts',(38.9179120423565,-3.03130325382365,-11.9139527583822));
#62449=CARTESIAN_POINT('Ctrl Pts',(38.9463001317429,-3.0337272063567,-11.9171340103329));
#62450=CARTESIAN_POINT('Ctrl Pts',(39.050078705026,-3.04263028380864,-11.9268957445653));
#62451=CARTESIAN_POINT('Ctrl Pts',(39.1257036524631,-3.04920019853352,-11.9304224195146));
#62452=CARTESIAN_POINT('Ctrl Pts',(39.3970729025622,-3.07308627547469,-11.9302688873136));
#62453=CARTESIAN_POINT('Ctrl Pts',(39.592011822878,-3.09089771757061,-11.9062746803096));
#62454=CARTESIAN_POINT('Ctrl Pts',(39.8325940921913,-3.11286321237424,-11.8462948462959));
#62455=CARTESIAN_POINT('Ctrl Pts',(39.8828908118675,-3.11744883283595,-11.8319994102766));
#62456=CARTESIAN_POINT('Ctrl Pts',(39.9488701921998,-3.12342428717553,-11.8108991843903));
#62457=CARTESIAN_POINT('Ctrl Pts',(39.9649994062981,-3.12488179196278,-11.8055520395921));
#62458=CARTESIAN_POINT('Ctrl Pts',(39.9917098663996,-3.12728859259921,-11.796381727355));
#62459=CARTESIAN_POINT('Ctrl Pts',(40.0023231263142,-3.12824309705897,-11.792654534464));
#62460=CARTESIAN_POINT('Ctrl Pts',(40.0241026973336,-3.13019758625375,-11.7848338676353));
#62461=CARTESIAN_POINT('Ctrl Pts',(40.0352654538315,-3.13119706866889,-11.7807318115428));
#62462=CARTESIAN_POINT('Ctrl Pts',(40.0651637042264,-3.13386920599787,-11.7694925123443));
#62463=CARTESIAN_POINT('Ctrl Pts',(40.0838417246682,-3.13553337626812,-11.7622033344472));
#62464=CARTESIAN_POINT('Ctrl Pts',(40.1860640249784,-3.14462451426257,-11.7208305122501));
#62465=CARTESIAN_POINT('Ctrl Pts',(40.2677420373222,-3.15182808097302,-11.682295863224));
#62466=CARTESIAN_POINT('Ctrl Pts',(40.4779120656208,-3.1707065911303,-11.5682699367938));
#62467=CARTESIAN_POINT('Ctrl Pts',(40.6018787005989,-3.18222158329457,-11.4852927418002));
#62468=CARTESIAN_POINT('Ctrl Pts',(40.7787623865758,-3.20032910513542,-11.3414857126284));
#62469=CARTESIAN_POINT('Ctrl Pts',(40.8376383747717,-3.20668397014376,-11.2885898687909));
#62470=CARTESIAN_POINT('Ctrl Pts',(40.9138401663082,-3.21546638591471,-11.2130170859233));
#62471=CARTESIAN_POINT('Ctrl Pts',(40.933530992621,-3.21779040565194,-11.1927889434943));
#62472=CARTESIAN_POINT('Ctrl Pts',(40.9664265139555,-3.22177138350558,-11.1577837434004));
#62473=CARTESIAN_POINT('Ctrl Pts',(40.9798132625443,-3.22342045517352,-11.143181103333));
#62474=CARTESIAN_POINT('Ctrl Pts',(41.0049737547915,-3.22657716867864,-11.1150454044706));
#62475=CARTESIAN_POINT('Ctrl Pts',(41.0167795265731,-3.22808333805738,-11.1015426598486));
#62476=CARTESIAN_POINT('Ctrl Pts',(41.0471846758565,-3.23202943847918,-11.0659719677585));
#62477=CARTESIAN_POINT('Ctrl Pts',(41.0655392514378,-3.23447899622937,-11.0436997654892));
#62478=CARTESIAN_POINT('Ctrl Pts',(41.1323949476538,-3.24366252086882,-10.959533215383));
#62479=CARTESIAN_POINT('Ctrl Pts',(41.1782473047807,-3.25049536623026,-10.8956095295234));
#62480=CARTESIAN_POINT('Ctrl Pts',(41.3247542283779,-3.27430112158797,-10.6686574124892));
#62481=CARTESIAN_POINT('Ctrl Pts',(41.409024172745,-3.2917250180917,-10.4959443470384));
#62482=CARTESIAN_POINT('Ctrl Pts',(41.4892366481062,-3.31336340570383,-10.2652888262993));
#62483=CARTESIAN_POINT('Ctrl Pts',(41.5049123780111,-3.31798912518039,-10.2149362451749));
#62484=CARTESIAN_POINT('Ctrl Pts',(41.5234491569062,-3.32400770370209,-10.1476775219903));
#62485=CARTESIAN_POINT('Ctrl Pts',(41.5278019821482,-3.32546941382646,-10.1312023295843));
#62486=CARTESIAN_POINT('Ctrl Pts',(41.5347393171738,-3.32788120684464,-10.1037676518486));
#62487=CARTESIAN_POINT('Ctrl Pts',(41.5374225516675,-3.32883654233937,-10.0928340528802));
#62488=CARTESIAN_POINT('Ctrl Pts',(41.5424358324578,-3.3306655171095,-10.0717681300744));
#62489=CARTESIAN_POINT('Ctrl Pts',(41.544777099896,-3.33153982056055,-10.0616389677891));
#62490=CARTESIAN_POINT('Ctrl Pts',(41.5510784718428,-3.33395115290408,-10.033548175126));
#62491=CARTESIAN_POINT('Ctrl Pts',(41.5548984717067,-3.33548062314349,-10.0155552758631));
#62492=CARTESIAN_POINT('Ctrl Pts',(41.5706655284014,-3.34211212739278,-9.93685631979261));
#62493=CARTESIAN_POINT('Ctrl Pts',(41.5804755878746,-3.34711163142915,-9.87573978007214));
#62494=CARTESIAN_POINT('Ctrl Pts',(41.606512469333,-3.36438811380741,-9.66083274944916));
#62495=CARTESIAN_POINT('Ctrl Pts',(41.6102684935216,-3.37632344124629,-9.50591696153514));
#62496=CARTESIAN_POINT('Ctrl Pts',(41.5918945590781,-3.39644548904117,-9.25154476645736));
#62497=CARTESIAN_POINT('Ctrl Pts',(41.5783956055124,-3.40445427168342,-9.15194845928137));
#62498=CARTESIAN_POINT('Ctrl Pts',(41.5527848385508,-3.41512501698208,-9.02382964780018));
#62499=CARTESIAN_POINT('Ctrl Pts',(41.5462956488388,-3.41761175062244,-8.99427899859305));
#62500=CARTESIAN_POINT('Ctrl Pts',(41.5345484472633,-3.42178763145481,-8.94522046040301));
#62501=CARTESIAN_POINT('Ctrl Pts',(41.529598745462,-3.42346693059095,-8.92564167616314));
#62502=CARTESIAN_POINT('Ctrl Pts',(41.5193413489712,-3.42679793810188,-8.88711621115025));
#62503=CARTESIAN_POINT('Ctrl Pts',(41.5140465259434,-3.42844911613836,-8.86816771717611));
#62504=CARTESIAN_POINT('Ctrl Pts',(41.5004944834659,-3.4325165758252,-8.82186824289984));
#62505=CARTESIAN_POINT('Ctrl Pts',(41.4919814756648,-3.43494089104611,-8.79459607041152));
#62506=CARTESIAN_POINT('Ctrl Pts',(41.4591412638438,-3.44384763244424,-8.69562306084226));
#62507=CARTESIAN_POINT('Ctrl Pts',(41.4319208252656,-3.45042095062522,-8.62493767753455));
#62508=CARTESIAN_POINT('Ctrl Pts',(41.3225690784297,-3.47430592029768,-8.3765945579448));
#62509=CARTESIAN_POINT('Ctrl Pts',(41.2221811910276,-3.49211226025945,-8.20784244334291));
#62510=CARTESIAN_POINT('Ctrl Pts',(41.0704901137421,-3.51407344239522,-8.01177417749548));
#62511=CARTESIAN_POINT('Ctrl Pts',(41.0371595847783,-3.51865958328926,-7.97147774174081));
#62512=CARTESIAN_POINT('Ctrl Pts',(40.991287933232,-3.52463559765534,-7.91956261177279));
#62513=CARTESIAN_POINT('Ctrl Pts',(40.9799018011249,-3.52609315729551,-7.90694830225337));
#62514=CARTESIAN_POINT('Ctrl Pts',(40.9607575803957,-3.52850002302619,-7.88618573055764));
#62515=CARTESIAN_POINT('Ctrl Pts',(40.9530744781089,-3.52945453830076,-7.87796953166388));
#62516=CARTESIAN_POINT('Ctrl Pts',(40.9371506181777,-3.5314090222328,-7.86117846804725));
#62517=CARTESIAN_POINT('Ctrl Pts',(40.9289034376554,-3.53240848881143,-7.85261030779499));
#62518=CARTESIAN_POINT('Ctrl Pts',(40.9065836142058,-3.53508053544583,-7.82976337805812));
#62519=CARTESIAN_POINT('Ctrl Pts',(40.8923950237439,-3.5367446318517,-7.81559834997993));
#62520=CARTESIAN_POINT('Ctrl Pts',(40.8134010540452,-3.54583385263985,-7.73868343140284));
#62521=CARTESIAN_POINT('Ctrl Pts',(40.7452736921767,-3.55303569001522,-7.67943134571003));
#62522=CARTESIAN_POINT('Ctrl Pts',(40.5563197333229,-3.57191400639663,-7.53291225900167));
#62523=CARTESIAN_POINT('Ctrl Pts',(40.430457359045,-3.58343037638657,-7.45280509602672));
#62524=CARTESIAN_POINT('Ctrl Pts',(40.2276077006718,-3.60153969653769,-7.34873389792574));
#62525=CARTESIAN_POINT('Ctrl Pts',(40.1554872207818,-3.60789491485214,-7.31611938790898));
#62526=CARTESIAN_POINT('Ctrl Pts',(40.0556341662975,-3.61667773817527,-7.27676958468121));
#62527=CARTESIAN_POINT('Ctrl Pts',(40.0291918070063,-3.61900179903486,-7.26688338687173));
#62528=CARTESIAN_POINT('Ctrl Pts',(39.9839078222573,-3.62298282572918,-7.25085534501553));
#62529=CARTESIAN_POINT('Ctrl Pts',(39.9651526129791,-3.62463190463479,-7.24447663567411));
#62530=CARTESIAN_POINT('Ctrl Pts',(39.9292706200044,-3.62778861751208,-7.23276549992536));
#62531=CARTESIAN_POINT('Ctrl Pts',(39.9121587003754,-3.62929477889295,-7.22739155016619));
#62532=CARTESIAN_POINT('Ctrl Pts',(39.8718071370074,-3.63284913272507,-7.21521333208578));
#62533=CARTESIAN_POINT('Ctrl Pts',(39.8485221213355,-3.63490226679751,-7.20856777637765));
#62534=CARTESIAN_POINT('Ctrl Pts',(39.7632576842616,-3.64243068491006,-7.18561957829622));
#62535=CARTESIAN_POINT('Ctrl Pts',(39.7007394313206,-3.64797138817349,-7.17144558562971));
#62536=CARTESIAN_POINT('Ctrl Pts',(39.42778098935,-3.67227257358065,-7.12092852591869));
#62537=CARTESIAN_POINT('Ctrl Pts',(39.2135934214388,-3.69173420860046,-7.11020470266322));
#62538=CARTESIAN_POINT('Ctrl Pts',(38.9505265241898,-3.71510047949061,-7.13205896541279));
#62539=CARTESIAN_POINT('Ctrl Pts',(38.9003329110166,-3.71952800606988,-7.13782500768089));
#62540=CARTESIAN_POINT('Ctrl Pts',(38.8337349334314,-3.7253329289799,-7.14760962759376));
#62541=CARTESIAN_POINT('Ctrl Pts',(38.8171416878524,-3.72677343218744,-7.15022534880261));
#62542=CARTESIAN_POINT('Ctrl Pts',(38.7895212741357,-3.7291600898002,-7.15487640756048));
#62543=CARTESIAN_POINT('Ctrl Pts',(38.7784787424096,-3.73011127537068,-7.15681536185065));
#62544=CARTESIAN_POINT('Ctrl Pts',(38.7556902579504,-3.73206757209957,-7.16098123923111));
#62545=CARTESIAN_POINT('Ctrl Pts',(38.7439466901258,-3.73307210490017,-7.16321862868808));
#62546=CARTESIAN_POINT('Ctrl Pts',(38.7122700655126,-3.73577318129861,-7.16949875931177));
#62547=CARTESIAN_POINT('Ctrl Pts',(38.6923701824208,-3.7374609208376,-7.17370702881564));
#62548=CARTESIAN_POINT('Ctrl Pts',(38.5748486350137,-3.74738727405593,-7.2001212139168));
#62549=CARTESIAN_POINT('Ctrl Pts',(38.4786229707858,-3.7553492313819,-7.22815504570517));
#62550=CARTESIAN_POINT('Ctrl Pts',(38.2517901766377,-3.77433805778187,-7.30990982442521));
#62551=CARTESIAN_POINT('Ctrl Pts',(38.1236307310857,-3.78526474956412,-7.36927397041474));
#62552=CARTESIAN_POINT('Ctrl Pts',(37.9345660810682,-3.80259913358369,-7.47793534515349));
#62553=CARTESIAN_POINT('Ctrl Pts',(37.8696160611345,-3.80879682619454,-7.5195391838841));
#62554=CARTESIAN_POINT('Ctrl Pts',(37.7839579303474,-3.81739773492141,-7.58040192927074));
#62555=CARTESIAN_POINT('Ctrl Pts',(37.7614209034836,-3.81970316909896,-7.5970148210287));
#62556=CARTESIAN_POINT('Ctrl Pts',(37.7234746200217,-3.8236621004384,-7.62602223874005));
#62557=CARTESIAN_POINT('Ctrl Pts',(37.7079184488684,-3.82530792758393,-7.63822064582628));
#62558=CARTESIAN_POINT('Ctrl Pts',(37.6785056797047,-3.82846504808786,-7.66187596252465));
#62559=CARTESIAN_POINT('Ctrl Pts',(37.6646236602856,-3.82997492937238,-7.67329926726274));
#62560=CARTESIAN_POINT('Ctrl Pts',(37.628605194894,-3.83394588123036,-7.70362182102778));
#62561=CARTESIAN_POINT('Ctrl Pts',(37.6066821654292,-3.83641681969319,-7.72276854355615));
#62562=CARTESIAN_POINT('Ctrl Pts',(37.5248935003285,-3.84584778474228,-7.79685841203626));
#62563=CARTESIAN_POINT('Ctrl Pts',(37.467484766387,-3.85291415342636,-7.85441838956483));
#62564=CARTESIAN_POINT('Ctrl Pts',(37.2984397129121,-3.87519073521511,-8.04200962359141));
#62565=CARTESIAN_POINT('Ctrl Pts',(37.1976999510234,-3.89072343726094,-8.18113360016381));
#62566=CARTESIAN_POINT('Ctrl Pts',(37.0793087148385,-3.91195051591422,-8.38789393332895));
#62567=CARTESIAN_POINT('Ctrl Pts',(37.0484565784658,-3.91786258999103,-8.44740792370253));
#62568=CARTESIAN_POINT('Ctrl Pts',(37.0123700360756,-3.92523959975757,-8.52476764381252));
#62569=CARTESIAN_POINT('Ctrl Pts',(37.0048033112149,-3.9268159811864,-8.54148528931296));
#62570=CARTESIAN_POINT('Ctrl Pts',(36.9927957553069,-3.9293650671299,-8.56884351078396));
#62571=CARTESIAN_POINT('Ctrl Pts',(36.9882389937428,-3.93034424281718,-8.5794318752999));
#62572=CARTESIAN_POINT('Ctrl Pts',(36.9798112609118,-3.93217730941835,-8.59940936172578));
#62573=CARTESIAN_POINT('Ctrl Pts',(36.9759233210151,-3.9330322179764,-8.60879096011471));
#62574=CARTESIAN_POINT('Ctrl Pts',(36.9673099539575,-3.9349479872454,-8.62995296428858));
#62575=CARTESIAN_POINT('Ctrl Pts',(36.9626180963518,-3.93600691130961,-8.64174676749004));
#62576=CARTESIAN_POINT('Ctrl Pts',(36.958019684865,-3.93706097182542,-8.65357747851738));
#62577=CARTESIAN_POINT('Origin',(39.2,8.05522481984854,-9.525));
#62578=CARTESIAN_POINT('',(36.9580198925264,-5.47085833376936,-8.6535769442499));
#62579=CARTESIAN_POINT('',(36.9580195978366,-5.20345233470371,-8.65357770242256));
#62580=CARTESIAN_POINT('',(36.958019684865,8.05522481984854,-8.65357747851728));
#62581=CARTESIAN_POINT('',(36.7946209885083,-4.27538907091946,-9.5271273713836));
#62582=CARTESIAN_POINT('Ctrl Pts',(36.9580198925264,-5.47085833376936,-8.65357694424991));
#62583=CARTESIAN_POINT('Ctrl Pts',(36.9952595237356,-5.46277457665365,-8.55776755312851));
#62584=CARTESIAN_POINT('Ctrl Pts',(37.0386247691785,-5.45461778154573,-8.46438559009306));
#62585=CARTESIAN_POINT('Ctrl Pts',(37.1056162592304,-5.44325209572759,-8.34145253667686));
#62586=CARTESIAN_POINT('Ctrl Pts',(37.124108616556,-5.44021917316755,-8.30930985803724));
#62587=CARTESIAN_POINT('Ctrl Pts',(37.1546361376661,-5.43536238716226,-8.25897690494473));
#62588=CARTESIAN_POINT('Ctrl Pts',(37.1661890441466,-5.43355579258796,-8.24049981009226));
#62589=CARTESIAN_POINT('Ctrl Pts',(37.1873822729682,-5.43029518366753,-8.20760732089903));
#62590=CARTESIAN_POINT('Ctrl Pts',(37.1969306018763,-5.42884462881036,-8.19313418882667));
#62591=CARTESIAN_POINT('Ctrl Pts',(37.2198200133046,-5.42540924812751,-8.15924188951536));
#62592=CARTESIAN_POINT('Ctrl Pts',(37.2332913346773,-5.42341966520666,-8.13991338286865));
#62593=CARTESIAN_POINT('Ctrl Pts',(37.2745907558289,-5.41741263346382,-8.08247485069053));
#62594=CARTESIAN_POINT('Ctrl Pts',(37.3032568255642,-5.41336393379002,-8.04498505828743));
#62595=CARTESIAN_POINT('Ctrl Pts',(37.37324146227,-5.40374446103385,-7.95883314863532));
#62596=CARTESIAN_POINT('Ctrl Pts',(37.4154297141937,-5.39814367745725,-7.91092662909951));
#62597=CARTESIAN_POINT('Ctrl Pts',(37.5275699675128,-5.38374392300581,-7.7933632983783));
#62598=CARTESIAN_POINT('Ctrl Pts',(37.5999952297682,-5.37487933463865,-7.7262309232486));
#62599=CARTESIAN_POINT('Ctrl Pts',(37.7689183410649,-5.35526201927055,-7.58794683865562));
#62600=CARTESIAN_POINT('Ctrl Pts',(37.8670423877495,-5.3445326041192,-7.5191583393165));
#62601=CARTESIAN_POINT('Ctrl Pts',(37.987653042601,-5.33236951226657,-7.44738236265103));
#62602=CARTESIAN_POINT('Ctrl Pts',(38.0055520857263,-5.33058960973234,-7.43704059898525));
#62603=CARTESIAN_POINT('Ctrl Pts',(38.0340735883837,-5.32779534910148,-7.42104819530141));
#62604=CARTESIAN_POINT('Ctrl Pts',(38.0446083734972,-5.3267721658066,-7.4152446106881));
#62605=CARTESIAN_POINT('Ctrl Pts',(38.0650152825358,-5.32480789650844,-7.40420120493602));
#62606=CARTESIAN_POINT('Ctrl Pts',(38.0748810290998,-5.32386623922299,-7.39895081242697));
#62607=CARTESIAN_POINT('Ctrl Pts',(38.0994878188598,-5.32153648255053,-7.38607472921195));
#62608=CARTESIAN_POINT('Ctrl Pts',(38.1142722791227,-5.32015337640034,-7.37853226471361));
#62609=CARTESIAN_POINT('Ctrl Pts',(38.1727709749811,-5.3147412159474,-7.34944757971296));
#62610=CARTESIAN_POINT('Ctrl Pts',(38.2170612757656,-5.31077528231635,-7.32908101242674));
#62611=CARTESIAN_POINT('Ctrl Pts',(38.4767628571486,-5.28809341421452,-7.21909339367113));
#62612=CARTESIAN_POINT('Ctrl Pts',(38.7036803471764,-5.27039467113278,-7.1598443529106));
#62613=CARTESIAN_POINT('Ctrl Pts',(38.9880514015228,-5.24739370287977,-7.12839485222316));
#62614=CARTESIAN_POINT('Ctrl Pts',(39.0406820737562,-5.24310974667196,-7.12432187748376));
#62615=CARTESIAN_POINT('Ctrl Pts',(39.1179236018891,-5.23675638333033,-7.12089539046101));
#62616=CARTESIAN_POINT('Ctrl Pts',(39.1424609282994,-5.23472843251291,-7.12018302710016));
#62617=CARTESIAN_POINT('Ctrl Pts',(39.1862693323847,-5.23108797961879,-7.1195820243055));
#62618=CARTESIAN_POINT('Ctrl Pts',(39.205536581584,-5.22948005637867,-7.11954921694751));
#62619=CARTESIAN_POINT('Ctrl Pts',(39.2465870623378,-5.22603848844538,-7.11997250568584));
#62620=CARTESIAN_POINT('Ctrl Pts',(39.2683677092172,-5.22420299588322,-7.12049310832679));
#62621=CARTESIAN_POINT('Ctrl Pts',(39.3281588657947,-5.21913649896992,-7.12273525508449));
#62622=CARTESIAN_POINT('Ctrl Pts',(39.3661385737245,-5.21588725495576,-7.12506287165176));
#62623=CARTESIAN_POINT('Ctrl Pts',(39.5288318176334,-5.2018258112237,-7.13891382610556));
#62624=CARTESIAN_POINT('Ctrl Pts',(39.6525768907362,-5.19075529625799,-7.15926507153355));
#62625=CARTESIAN_POINT('Ctrl Pts',(39.9134242802172,-5.16670180232868,-7.22338184221743));
#62626=CARTESIAN_POINT('Ctrl Pts',(40.0493555975232,-5.15371784252894,-7.27000139908325));
#62627=CARTESIAN_POINT('Ctrl Pts',(40.2158631063779,-5.13767180753853,-7.34431447983958));
#62628=CARTESIAN_POINT('Ctrl Pts',(40.251010849335,-5.13427769872927,-7.36103514827078));
#62629=CARTESIAN_POINT('Ctrl Pts',(40.2997452158124,-5.12957566174219,-7.38568708782715));
#62630=CARTESIAN_POINT('Ctrl Pts',(40.3136812338339,-5.12823156394618,-7.39290867312603));
#62631=CARTESIAN_POINT('Ctrl Pts',(40.3372818086305,-5.12595736250596,-7.40543294322179));
#62632=CARTESIAN_POINT('Ctrl Pts',(40.3469821986928,-5.12502322657124,-7.41066646918281));
#62633=CARTESIAN_POINT('Ctrl Pts',(40.3675108099487,-5.12304799989191,-7.42192487603242));
#62634=CARTESIAN_POINT('Ctrl Pts',(40.3783289376723,-5.12200798176452,-7.4279669997374));
#62635=CARTESIAN_POINT('Ctrl Pts',(40.4085615156707,-5.11910257882854,-7.44516028503417));
#62636=CARTESIAN_POINT('Ctrl Pts',(40.4278683714197,-5.11724838786384,-7.45649968585288));
#62637=CARTESIAN_POINT('Ctrl Pts',(40.5679614385546,-5.1037811565107,-7.5414327513729));
#62638=CARTESIAN_POINT('Ctrl Pts',(40.6822254997664,-5.09271595196789,-7.6252952056509));
#62639=CARTESIAN_POINT('Ctrl Pts',(40.9029700060062,-5.06968870244783,-7.8194222510935));
#62640=CARTESIAN_POINT('Ctrl Pts',(41.0076219690653,-5.05776539702349,-7.93076135256273));
#62641=CARTESIAN_POINT('Ctrl Pts',(41.1242252562459,-5.04232431529775,-8.08117046470317));
#62642=CARTESIAN_POINT('Ctrl Pts',(41.1467125382999,-5.03922875957192,-8.11163644286042));
#62643=CARTESIAN_POINT('Ctrl Pts',(41.1810900905479,-5.03429495010918,-8.16058906959175));
#62644=CARTESIAN_POINT('Ctrl Pts',(41.1934627916882,-5.03247493448336,-8.17873064876448));
#62645=CARTESIAN_POINT('Ctrl Pts',(41.2151457588537,-5.02920285032391,-8.21147785722361));
#62646=CARTESIAN_POINT('Ctrl Pts',(41.224550052118,-5.02775439584812,-8.22601966829421));
#62647=CARTESIAN_POINT('Ctrl Pts',(41.2462528638732,-5.02434090257683,-8.26038684822782));
#62648=CARTESIAN_POINT('Ctrl Pts',(41.2584213571337,-5.02237129796934,-8.28029174476192));
#62649=CARTESIAN_POINT('Ctrl Pts',(41.2936888652565,-5.01649130197676,-8.33991320992022));
#62650=CARTESIAN_POINT('Ctrl Pts',(41.3159402087058,-5.01255161034865,-8.3801156471563));
#62651=CARTESIAN_POINT('Ctrl Pts',(41.4023414680293,-4.99625099492513,-8.54735258917987));
#62652=CARTESIAN_POINT('Ctrl Pts',(41.4562992913907,-4.98356939668883,-8.67930324580215));
#62653=CARTESIAN_POINT('Ctrl Pts',(41.5379166258791,-4.95872118621878,-8.94358269746234));
#62654=CARTESIAN_POINT('Ctrl Pts',(41.5667385457816,-4.94661212878722,-9.0750488606894));
#62655=CARTESIAN_POINT('Ctrl Pts',(41.5876930035189,-4.9327602439805,-9.232787721622));
#62656=CARTESIAN_POINT('Ctrl Pts',(41.5905743522289,-4.93062030754814,-9.25738029599692));
#62657=CARTESIAN_POINT('Ctrl Pts',(41.5943917267559,-4.92738289666199,-9.29497620979715));
#62658=CARTESIAN_POINT('Ctrl Pts',(41.5956025465786,-4.92627196598824,-9.30794897289716));
#62659=CARTESIAN_POINT('Ctrl Pts',(41.5976311401401,-4.92424373154533,-9.33177403046012));
#62660=CARTESIAN_POINT('Ctrl Pts',(41.5984807336038,-4.92332485333288,-9.34262253342965));
#62661=CARTESIAN_POINT('Ctrl Pts',(41.6002959705358,-4.92118467918,-9.36801401929874));
#62662=CARTESIAN_POINT('Ctrl Pts',(41.60120311266,-4.91996655436588,-9.38256057705231));
#62663=CARTESIAN_POINT('Ctrl Pts',(41.603792244002,-4.91591810771237,-9.43119050885038));
#62664=CARTESIAN_POINT('Ctrl Pts',(41.6048812931098,-4.91311724508659,-9.46530332553512));
#62665=CARTESIAN_POINT('Ctrl Pts',(41.6057899080726,-4.90617069602086,-9.55077329097243));
#62666=CARTESIAN_POINT('Ctrl Pts',(41.6046916533188,-4.90206119574809,-9.60212462268245));
#62667=CARTESIAN_POINT('Ctrl Pts',(41.5921734991456,-4.88345330538711,-9.83628950761009));
#62668=CARTESIAN_POINT('Ctrl Pts',(41.561542776729,-4.86937780776652,-10.0174565033301));
#62669=CARTESIAN_POINT('Ctrl Pts',(41.4927417446297,-4.84960001703423,-10.2553022208268));
#62670=CARTESIAN_POINT('Ctrl Pts',(41.4723552008387,-4.84439769625684,-10.3164584799679));
#62671=CARTESIAN_POINT('Ctrl Pts',(41.4409484308044,-4.83712957474374,-10.3994093952956));
#62672=CARTESIAN_POINT('Ctrl Pts',(41.4320144919434,-4.83513091732007,-10.4219687182125));
#62673=CARTESIAN_POINT('Ctrl Pts',(41.4158801731828,-4.83163405031406,-10.4609755415955));
#62674=CARTESIAN_POINT('Ctrl Pts',(41.4088339336347,-4.83014102781194,-10.4774850515771));
#62675=CARTESIAN_POINT('Ctrl Pts',(41.3936262066864,-4.82698755311929,-10.5120406464656));
#62676=CARTESIAN_POINT('Ctrl Pts',(41.3854253287289,-4.82532587034114,-10.5300677862163));
#62677=CARTESIAN_POINT('Ctrl Pts',(41.3650183403392,-4.82128117877937,-10.5734954156536));
#62678=CARTESIAN_POINT('Ctrl Pts',(41.3525869398724,-4.81889065602758,-10.5987859990957));
#62679=CARTESIAN_POINT('Ctrl Pts',(41.3037872305908,-4.80977035477408,-10.6938101943024));
#62680=CARTESIAN_POINT('Ctrl Pts',(41.2644550852237,-4.80294069384992,-10.7619560504568));
#62681=CARTESIAN_POINT('Ctrl Pts',(41.1422397220461,-4.78306905905059,-10.9515905637411));
#62682=CARTESIAN_POINT('Ctrl Pts',(41.0514678854628,-4.76980822234398,-11.0675674287773));
#62683=CARTESIAN_POINT('Ctrl Pts',(40.8872396364637,-4.74834047988365,-11.2418684736214));
#62684=CARTESIAN_POINT('Ctrl Pts',(40.8199436590886,-4.74010445566711,-11.3055060466609));
#62685=CARTESIAN_POINT('Ctrl Pts',(40.7337333010786,-4.73034423420925,-11.3780841019535));
#62686=CARTESIAN_POINT('Ctrl Pts',(40.7181638346249,-4.72861091387313,-11.3908609757667));
#62687=CARTESIAN_POINT('Ctrl Pts',(40.6931314230891,-4.72587265826061,-11.4108826648556));
#62688=CARTESIAN_POINT('Ctrl Pts',(40.6837724260908,-4.72485945997,-11.4182549429006));
#62689=CARTESIAN_POINT('Ctrl Pts',(40.6654777278209,-4.72289990739667,-11.432447066174));
#62690=CARTESIAN_POINT('Ctrl Pts',(40.6565484084893,-4.72195311119634,-11.4392742813818));
#62691=CARTESIAN_POINT('Ctrl Pts',(40.6340441756963,-4.719590040886,-11.4562320246187));
#62692=CARTESIAN_POINT('Ctrl Pts',(40.6204091094291,-4.71817908314182,-11.4662825253065));
#62693=CARTESIAN_POINT('Ctrl Pts',(40.5646861562773,-4.71249127626714,-11.5064548175052));
#62694=CARTESIAN_POINT('Ctrl Pts',(40.5217336504703,-4.70828601789915,-11.5353613484773));
#62695=CARTESIAN_POINT('Ctrl Pts',(40.3083314051909,-4.68806546734245,-11.6691790076998));
#62696=CARTESIAN_POINT('Ctrl Pts',(40.1261723761242,-4.67276760209691,-11.7539277827152));
#62697=CARTESIAN_POINT('Ctrl Pts',(39.8663984223725,-4.65105265712098,-11.8373689801358));
#62698=CARTESIAN_POINT('Ctrl Pts',(39.796223232101,-4.64520364297387,-11.8564487235966));
#62699=CARTESIAN_POINT('Ctrl Pts',(39.6977666161631,-4.63694724543407,-11.8784819443695));
#62700=CARTESIAN_POINT('Ctrl Pts',(39.6701304420351,-4.63462454706768,-11.8841579215339));
#62701=CARTESIAN_POINT('Ctrl Pts',(39.6231230971082,-4.63066117815669,-11.892953647643));
#62702=CARTESIAN_POINT('Ctrl Pts',(39.6038014291256,-4.62902852061959,-11.8963249441562));
#62703=CARTESIAN_POINT('Ctrl Pts',(39.5644161244845,-4.62569197211084,-11.9027016952473));
#62704=CARTESIAN_POINT('Ctrl Pts',(39.5443514265039,-4.62398769773444,-11.9056903419996));
#62705=CARTESIAN_POINT('Ctrl Pts',(39.4938340991769,-4.61968412972374,-11.9125629495981));
#62706=CARTESIAN_POINT('Ctrl Pts',(39.4633413708639,-4.61707488978525,-11.916118242847));
#62707=CARTESIAN_POINT('Ctrl Pts',(39.326923574192,-4.60534388986004,-11.9293828957315));
#62708=CARTESIAN_POINT('Ctrl Pts',(39.220508077027,-4.59603007609643,-11.9326418632413));
#62709=CARTESIAN_POINT('Ctrl Pts',(39.0231904332455,-4.57846898434809,-11.9256024560702));
#62710=CARTESIAN_POINT('Ctrl Pts',(38.932401549067,-4.57027540034288,-11.9171837952093));
#62711=CARTESIAN_POINT('Ctrl Pts',(38.7380049948022,-4.55261422397464,-11.8879515325751));
#62712=CARTESIAN_POINT('Ctrl Pts',(38.6348290555813,-4.54316669485518,-11.8654200449498));
#62713=CARTESIAN_POINT('Ctrl Pts',(38.5087643842345,-4.53173863575749,-11.8290630747263));
#62714=CARTESIAN_POINT('Ctrl Pts',(38.4841869540101,-4.52951655122016,-11.8215463577246));
#62715=CARTESIAN_POINT('Ctrl Pts',(38.4473048195213,-4.5261954216782,-11.8096167153856));
#62716=CARTESIAN_POINT('Ctrl Pts',(38.4349088871332,-4.52508152047773,-11.8054953813695));
#62717=CARTESIAN_POINT('Ctrl Pts',(38.4122528865247,-4.52305064552759,-11.797757301889));
#62718=CARTESIAN_POINT('Ctrl Pts',(38.4019832868098,-4.52213206422272,-11.7941717881331));
#62719=CARTESIAN_POINT('Ctrl Pts',(38.3780566166997,-4.51999617280301,-11.7856355331143));
#62720=CARTESIAN_POINT('Ctrl Pts',(38.3644195373108,-4.51878198989379,-11.780630568632));
#62721=CARTESIAN_POINT('Ctrl Pts',(38.3191782179908,-4.51476177276066,-11.7635598645217));
#62722=CARTESIAN_POINT('Ctrl Pts',(38.2877813708595,-4.51198464128137,-11.7509503132214));
#62723=CARTESIAN_POINT('Ctrl Pts',(38.2100120615735,-4.50511219978048,-11.7177946156581));
#62724=CARTESIAN_POINT('Ctrl Pts',(38.1640023430201,-4.50105209090411,-11.696435927314));
#62725=CARTESIAN_POINT('Ctrl Pts',(37.9546189820863,-4.48244504208671,-11.5910638029214));
#62726=CARTESIAN_POINT('Ctrl Pts',(37.8005388598102,-4.46833085895413,-11.4899694158746));
#62727=CARTESIAN_POINT('Ctrl Pts',(37.6096948390994,-4.44848469402268,-11.3308188746062));
#62728=CARTESIAN_POINT('Ctrl Pts',(37.5616287664727,-4.44325427505207,-11.2873253492816));
#62729=CARTESIAN_POINT('Ctrl Pts',(37.4980196805413,-4.43595253749243,-11.2249139679507));
#62730=CARTESIAN_POINT('Ctrl Pts',(37.480918748672,-4.43394917370213,-11.207618218903));
#62731=CARTESIAN_POINT('Ctrl Pts',(37.4516485250698,-4.4304464830367,-11.1771025294082));
#62732=CARTESIAN_POINT('Ctrl Pts',(37.4393593986464,-4.42895238789145,-11.163999781525));
#62733=CARTESIAN_POINT('Ctrl Pts',(37.4138420416727,-4.42579904189795,-11.1361748440464));
#62734=CARTESIAN_POINT('Ctrl Pts',(37.4006465266495,-4.42413858034533,-11.1214246484365));
#62735=CARTESIAN_POINT('Ctrl Pts',(37.3871262788759,-4.42240529599392,-11.1059308695077));
#62736=CARTESIAN_POINT('Ctrl Pts',(37.3866179060256,-4.42234007536982,-11.1053477225455));
#62737=CARTESIAN_POINT('Ctrl Pts',(37.3857177958894,-4.42222451311658,-11.1043142133637));
#62738=CARTESIAN_POINT('Ctrl Pts',(37.3853259444945,-4.42217417615615,-11.1038639501106));
#62739=CARTESIAN_POINT('Ctrl Pts',(37.3846231171822,-4.42208384040779,-11.1030557476077));
#62740=CARTESIAN_POINT('Ctrl Pts',(37.3843120793003,-4.4220438441541,-11.1026978620292));
#62741=CARTESIAN_POINT('Ctrl Pts',(37.3837486536747,-4.42197136088832,-11.1020491874478));
#62742=CARTESIAN_POINT('Ctrl Pts',(37.383496229809,-4.42193887535067,-11.1017584296713));
#62743=CARTESIAN_POINT('Ctrl Pts',(37.3820164477946,-4.42174836615,-11.1000530961666));
#62744=CARTESIAN_POINT('Ctrl Pts',(37.3807906758085,-4.42159027790435,-11.0986371521305));
#62745=CARTESIAN_POINT('Ctrl Pts',(37.3783399345589,-4.42127364151454,-11.0957995009524));
#62746=CARTESIAN_POINT('Ctrl Pts',(37.377114972979,-4.42111509320416,-11.0943777889452));
#62747=CARTESIAN_POINT('Ctrl Pts',(37.3746449761036,-4.42079482551441,-11.0915042735329));
#62748=CARTESIAN_POINT('Ctrl Pts',(37.3734000061919,-4.42063310363375,-11.0900524160025));
#62749=CARTESIAN_POINT('Ctrl Pts',(37.3708695737756,-4.42030379758371,-11.0870943471385));
#62750=CARTESIAN_POINT('Ctrl Pts',(37.3695842372668,-4.42013620848173,-11.0855880305159));
#62751=CARTESIAN_POINT('Ctrl Pts',(37.3669519858763,-4.41979234805102,-11.082495506436));
#62752=CARTESIAN_POINT('Ctrl Pts',(37.3656052668289,-4.41961606901278,-11.0809091353632));
#62753=CARTESIAN_POINT('Ctrl Pts',(37.3390630774199,-4.4161348498314,-11.0495613366961));
#62754=CARTESIAN_POINT('Ctrl Pts',(37.314594590791,-4.41280120192612,-11.0191952891368));
#62755=CARTESIAN_POINT('Ctrl Pts',(37.2602283217251,-4.40509534935517,-10.9482628167489));
#62756=CARTESIAN_POINT('Ctrl Pts',(37.2308465062441,-4.40070602922078,-10.9073259314246));
#62757=CARTESIAN_POINT('Ctrl Pts',(37.1298366205566,-4.38477112304315,-10.7568301094805));
#62758=CARTESIAN_POINT('Ctrl Pts',(37.0658975076619,-4.37300947777917,-10.6423993981754));
#62759=CARTESIAN_POINT('Ctrl Pts',(36.968135221261,-4.35184891748952,-10.4281019737769));
#62760=CARTESIAN_POINT('Ctrl Pts',(36.9309424719433,-4.34247395595559,-10.3301063844806));
#62761=CARTESIAN_POINT('Ctrl Pts',(36.8927321453947,-4.33111874617036,-10.2054602809163));
#62762=CARTESIAN_POINT('Ctrl Pts',(36.8856052751858,-4.32890040588748,-10.1808112266383));
#62763=CARTESIAN_POINT('Ctrl Pts',(36.8754490160686,-4.32558369539335,-10.1434545867036));
#62764=CARTESIAN_POINT('Ctrl Pts',(36.8721267631786,-4.3244705253407,-10.1308296546545));
#62765=CARTESIAN_POINT('Ctrl Pts',(36.8662246097815,-4.32244030236372,-10.1076351500212));
#62766=CARTESIAN_POINT('Ctrl Pts',(36.863613491522,-4.32152165002608,-10.0970746310514));
#62767=CARTESIAN_POINT('Ctrl Pts',(36.8585622955632,-4.31970234639919,-10.0760337452753));
#62768=CARTESIAN_POINT('Ctrl Pts',(36.8561208120645,-4.31880161382848,-10.0655544173153));
#62769=CARTESIAN_POINT('Ctrl Pts',(36.8505669167431,-4.31670032244282,-10.0409706731652));
#62770=CARTESIAN_POINT('Ctrl Pts',(36.847511012862,-4.31550271040201,-10.0268537072932));
#62771=CARTESIAN_POINT('Ctrl Pts',(36.8376137773697,-4.31147540321102,-9.97905451557714));
#62772=CARTESIAN_POINT('Ctrl Pts',(36.8313668298997,-4.30867371131835,-9.94525159629413));
#62773=CARTESIAN_POINT('Ctrl Pts',(36.805178275617,-4.29550206162921,-9.78430988895812));
#62774=CARTESIAN_POINT('Ctrl Pts',(36.79473479356,-4.28547290397762,-9.65583208521157));
#62775=CARTESIAN_POINT('Ctrl Pts',(36.7946209411353,-4.27538918813332,-9.52712780995419));
#62776=CARTESIAN_POINT('Ctrl Pts',(36.7946209407417,-4.27538915327001,-9.52712736497368));
#62777=CARTESIAN_POINT('Ctrl Pts',(36.7944991403118,-4.2645992395797,-9.38940948057675));
#62778=CARTESIAN_POINT('Ctrl Pts',(36.8062043998384,-4.25377919108456,-9.25194856682721));
#62779=CARTESIAN_POINT('Ctrl Pts',(36.8342255556644,-4.24039179038781,-9.08944994601524));
#62780=CARTESIAN_POINT('Ctrl Pts',(36.8393010269769,-4.23817159305936,-9.06273079798787));
#62781=CARTESIAN_POINT('Ctrl Pts',(36.8488385541642,-4.23431700667048,-9.01678537028102));
#62782=CARTESIAN_POINT('Ctrl Pts',(36.8530863144503,-4.23268922636811,-8.99751695765488));
#62783=CARTESIAN_POINT('Ctrl Pts',(36.8620704505594,-4.22941312977994,-8.9590226425274));
#62784=CARTESIAN_POINT('Ctrl Pts',(36.8668081349445,-4.22776489093062,-8.93979865086665));
#62785=CARTESIAN_POINT('Ctrl Pts',(36.8768942240024,-4.22440746598798,-8.90094357887893));
#62786=CARTESIAN_POINT('Ctrl Pts',(36.882255469653,-4.22269799330744,-8.88131754658095));
#62787=CARTESIAN_POINT('Ctrl Pts',(36.8964109360524,-4.21836377810118,-8.83196968524037));
#62788=CARTESIAN_POINT('Ctrl Pts',(36.9055316201117,-4.21572879034417,-8.80234638053156));
#62789=CARTESIAN_POINT('Ctrl Pts',(36.928440781962,-4.20945597332542,-8.73275060355609));
#62790=CARTESIAN_POINT('Ctrl Pts',(36.9427123752434,-4.20580426847111,-8.69295984675209));
#62791=CARTESIAN_POINT('Ctrl Pts',(36.9580197210495,-4.20212274557561,-8.6535773854226));
#62792=CARTESIAN_POINT('Ctrl Pts',(36.958019684865,-3.93706097182542,-8.65357747851738));
#62793=CARTESIAN_POINT('Ctrl Pts',(36.9564218065497,-3.93742724188324,-8.65768847133716));
#62794=CARTESIAN_POINT('Ctrl Pts',(36.9548352114531,-3.93779292469071,-8.66180392061865));
#62795=CARTESIAN_POINT('Ctrl Pts',(36.9356569182194,-3.94223798500041,-8.71196086723292));
#62796=CARTESIAN_POINT('Ctrl Pts',(36.9194713198563,-3.94624560074252,-8.75853270417446));
#62797=CARTESIAN_POINT('Ctrl Pts',(36.864362832756,-3.96105178130554,-8.93435194880606));
#62798=CARTESIAN_POINT('Ctrl Pts',(36.8349046012429,-3.97153258611843,-9.06631020610886));
#62799=CARTESIAN_POINT('Ctrl Pts',(36.8020319549446,-3.99062091621821,-9.30741523895724));
#62800=CARTESIAN_POINT('Ctrl Pts',(36.7946666042369,-3.99916619663588,-9.41563278385659));
#62801=CARTESIAN_POINT('Ctrl Pts',(36.7946011773878,-4.01150833552565,-9.56844855980404));
#62802=CARTESIAN_POINT('Ctrl Pts',(36.79581582193,-4.01513154800105,-9.61291598123295));
#62803=CARTESIAN_POINT('Ctrl Pts',(36.7995453838213,-4.02071170174965,-9.68061040585967));
#62804=CARTESIAN_POINT('Ctrl Pts',(36.8011670843105,-4.02264131717661,-9.70387852562828));
#62805=CARTESIAN_POINT('Ctrl Pts',(36.8047387400157,-4.02617713335041,-9.7462338917954));
#62806=CARTESIAN_POINT('Ctrl Pts',(36.8065792194015,-4.02777981633833,-9.76532865064845));
#62807=CARTESIAN_POINT('Ctrl Pts',(36.8110939448816,-4.03129326098282,-9.80694911871452));
#62808=CARTESIAN_POINT('Ctrl Pts',(36.813858820439,-4.03320669280442,-9.82946287332989));
#62809=CARTESIAN_POINT('Ctrl Pts',(36.8227271522041,-4.03873986384661,-9.89410526243208));
#62810=CARTESIAN_POINT('Ctrl Pts',(36.829630747841,-4.04238389676091,-9.93611312735005));
#62811=CARTESIAN_POINT('Ctrl Pts',(36.8614024510447,-4.05696273351156,-10.1018316111671));
#62812=CARTESIAN_POINT('Ctrl Pts',(36.8948696593243,-4.06814853415373,-10.2236684158856));
#62813=CARTESIAN_POINT('Ctrl Pts',(36.9918764428223,-4.09374584844926,-10.492181194954));
#62814=CARTESIAN_POINT('Ctrl Pts',(37.0607889311303,-4.10817963761743,-10.6363206319144));
#62815=CARTESIAN_POINT('Ctrl Pts',(37.1552599489578,-4.12400390981974,-10.7920472700935));
#62816=CARTESIAN_POINT('Ctrl Pts',(37.1673374996701,-4.1259674127758,-10.8113335241509));
#62817=CARTESIAN_POINT('Ctrl Pts',(37.186524970979,-4.12899317869822,-10.841028104447));
#62818=CARTESIAN_POINT('Ctrl Pts',(37.193445637932,-4.13006646650255,-10.8515561723586));
#62819=CARTESIAN_POINT('Ctrl Pts',(37.2065400300636,-4.13206314469821,-10.8711390617977));
#62820=CARTESIAN_POINT('Ctrl Pts',(37.2126931040418,-4.13298768399567,-10.8802063809301));
#62821=CARTESIAN_POINT('Ctrl Pts',(37.2275675907473,-4.1351907750014,-10.9018066099371));
#62822=CARTESIAN_POINT('Ctrl Pts',(37.2363467351261,-4.13646552409189,-10.9142990834695));
#62823=CARTESIAN_POINT('Ctrl Pts',(37.2677527313933,-4.14094014904069,-10.9580964062999));
#62824=CARTESIAN_POINT('Ctrl Pts',(37.291015541257,-4.14410148039958,-10.9889411361014));
#62825=CARTESIAN_POINT('Ctrl Pts',(37.3532668438202,-4.15221677799298,-11.0674726166837));
#62826=CARTESIAN_POINT('Ctrl Pts',(37.3933628543573,-4.15711703858195,-11.1142478033346));
#62827=CARTESIAN_POINT('Ctrl Pts',(37.5749194330834,-4.17821304081308,-11.3102840389316));
#62828=CARTESIAN_POINT('Ctrl Pts',(37.7333766102004,-4.19401602400693,-11.4425862530464));
#62829=CARTESIAN_POINT('Ctrl Pts',(37.9397928596778,-4.21385915489795,-11.5742118208705));
#62830=CARTESIAN_POINT('Ctrl Pts',(37.9733701704987,-4.21706308320526,-11.5944854528791));
#62831=CARTESIAN_POINT('Ctrl Pts',(38.0267432277663,-4.22212980257689,-11.6249562509932));
#62832=CARTESIAN_POINT('Ctrl Pts',(38.0462115668302,-4.22397262192054,-11.6357154930785));
#62833=CARTESIAN_POINT('Ctrl Pts',(38.0827640763653,-4.22742462980712,-11.6552595545121));
#62834=CARTESIAN_POINT('Ctrl Pts',(38.0998098367328,-4.22903126480804,-11.6641127688518));
#62835=CARTESIAN_POINT('Ctrl Pts',(38.1382644873064,-4.2326499394892,-11.6835041069582));
#62836=CARTESIAN_POINT('Ctrl Pts',(38.1597275238272,-4.23466567556183,-11.6939295437685));
#62837=CARTESIAN_POINT('Ctrl Pts',(38.2256085560158,-4.2408433961207,-11.7247277326397));
#62838=CARTESIAN_POINT('Ctrl Pts',(38.2704924972094,-4.245039358591,-11.7440664361145));
#62839=CARTESIAN_POINT('Ctrl Pts',(38.3498379074304,-4.25244119461422,-11.7754236517792));
#62840=CARTESIAN_POINT('Ctrl Pts',(38.3840434342024,-4.25562704870653,-11.7880503317101));
#62841=CARTESIAN_POINT('Ctrl Pts',(38.5448530055747,-4.27058084470239,-11.8432921579502));
#62842=CARTESIAN_POINT('Ctrl Pts',(38.6745687372117,-4.28259348784099,-11.8760871752182));
#62843=CARTESIAN_POINT('Ctrl Pts',(38.9061979690985,-4.30368191199174,-11.9145153563092));
#62844=CARTESIAN_POINT('Ctrl Pts',(39.0070345721715,-4.31273991162085,-11.924765014113));
#62845=CARTESIAN_POINT('Ctrl Pts',(39.1334064398001,-4.32375321629474,-11.9295900213183));
#62846=CARTESIAN_POINT('Ctrl Pts',(39.1586009642749,-4.3259319174706,-11.9301557423096));
#62847=CARTESIAN_POINT('Ctrl Pts',(39.1969194403864,-4.32921541775753,-11.9304138002995));
#62848=CARTESIAN_POINT('Ctrl Pts',(39.2100386630119,-4.33033423550841,-11.9303948304914));
#62849=CARTESIAN_POINT('Ctrl Pts',(39.2340252845103,-4.33236927472427,-11.9301638911338));
#62850=CARTESIAN_POINT('Ctrl Pts',(39.2448919407255,-4.33328716068351,-11.9299856107112));
#62851=CARTESIAN_POINT('Ctrl Pts',(39.2701931227031,-4.33541522225661,-11.9293989605366));
#62852=CARTESIAN_POINT('Ctrl Pts',(39.2846257302597,-4.33662234756427,-11.9289342657371));
#62853=CARTESIAN_POINT('Ctrl Pts',(39.3323416217746,-4.34059345891391,-11.9269676514473));
#62854=CARTESIAN_POINT('Ctrl Pts',(39.3655998126963,-4.34332949194643,-11.9249041516008));
#62855=CARTESIAN_POINT('Ctrl Pts',(39.4482560315581,-4.35007460462585,-11.9180490863296));
#62856=CARTESIAN_POINT('Ctrl Pts',(39.4975703308239,-4.35405013662522,-11.9124186127147));
#62857=CARTESIAN_POINT('Ctrl Pts',(39.7739691187715,-4.37623661433595,-11.8721619495239));
#62858=CARTESIAN_POINT('Ctrl Pts',(39.9953332907939,-4.39376263930941,-11.8066782966727));
#62859=CARTESIAN_POINT('Ctrl Pts',(40.2377413160252,-4.41542617959691,-11.6953271627589));
#62860=CARTESIAN_POINT('Ctrl Pts',(40.2710620332021,-4.4184592724644,-11.679078192295));
#62861=CARTESIAN_POINT('Ctrl Pts',(40.3231685859487,-4.42329978124538,-11.6521603460662));
#62862=CARTESIAN_POINT('Ctrl Pts',(40.34221001533,-4.42508975479324,-11.6419967001463));
#62863=CARTESIAN_POINT('Ctrl Pts',(40.3780117755566,-4.42849720944141,-11.6222633582596));
#62864=CARTESIAN_POINT('Ctrl Pts',(40.3947988349424,-4.43011275915449,-11.6127454430817));
#62865=CARTESIAN_POINT('Ctrl Pts',(40.4329614073952,-4.43382775217469,-11.5904970419608));
#62866=CARTESIAN_POINT('Ctrl Pts',(40.4542571842657,-4.43593176825608,-11.5776350572525));
#62867=CARTESIAN_POINT('Ctrl Pts',(40.5217924048129,-4.44270704139511,-11.535402519815));
#62868=CARTESIAN_POINT('Ctrl Pts',(40.5672260931139,-4.44742270445586,-11.5047841381315));
#62869=CARTESIAN_POINT('Ctrl Pts',(40.6756056243339,-4.45907604189103,-11.4262351695994));
#62870=CARTESIAN_POINT('Ctrl Pts',(40.7373053370498,-4.46606497161795,-11.3767011093379));
#62871=CARTESIAN_POINT('Ctrl Pts',(40.9135520980542,-4.4870885101725,-11.2203176539786));
#62872=CARTESIAN_POINT('Ctrl Pts',(41.0202307834518,-4.50129192912323,-11.1052288843261));
#62873=CARTESIAN_POINT('Ctrl Pts',(41.1413958517441,-4.51896084423093,-10.9458244190945));
#62874=CARTESIAN_POINT('Ctrl Pts',(41.1668721583249,-4.52277885190597,-10.9103427267695));
#62875=CARTESIAN_POINT('Ctrl Pts',(41.2005591177537,-4.52795503193203,-10.8606214054747));
#62876=CARTESIAN_POINT('Ctrl Pts',(41.2096095654249,-4.52935925031895,-10.8469647359009));
#62877=CARTESIAN_POINT('Ctrl Pts',(41.224516117627,-4.53169380532353,-10.8239645783502));
#62878=CARTESIAN_POINT('Ctrl Pts',(41.2304486495963,-4.53262887763718,-10.8146715823945));
#62879=CARTESIAN_POINT('Ctrl Pts',(41.2427370307949,-4.53457793323102,-10.7951274843059));
#62880=CARTESIAN_POINT('Ctrl Pts',(41.2490800114608,-4.53559111150193,-10.7848688541453));
#62881=CARTESIAN_POINT('Ctrl Pts',(41.2661696795052,-4.53834182694285,-10.7567588763515));
#62882=CARTESIAN_POINT('Ctrl Pts',(41.2767623626784,-4.54007000108603,-10.7388143404077));
#62883=CARTESIAN_POINT('Ctrl Pts',(41.3523452624266,-4.55259195563401,-10.6068863960687));
#62884=CARTESIAN_POINT('Ctrl Pts',(41.4081562780743,-4.56290474507926,-10.4878736187829));
#62885=CARTESIAN_POINT('Ctrl Pts',(41.5121044935809,-4.58623992287144,-10.2089091159635));
#62886=CARTESIAN_POINT('Ctrl Pts',(41.5538707783974,-4.59920569414261,-10.0473430206926));
#62887=CARTESIAN_POINT('Ctrl Pts',(41.5841763996209,-4.61574373888441,-9.84585705659293));
#62888=CARTESIAN_POINT('Ctrl Pts',(41.5888682028853,-4.61879654446586,-9.80882171248753));
#62889=CARTESIAN_POINT('Ctrl Pts',(41.5949362017491,-4.62367751744164,-9.74996794998442));
#62890=CARTESIAN_POINT('Ctrl Pts',(41.5968801361547,-4.62548810816445,-9.72821303334206));
#62891=CARTESIAN_POINT('Ctrl Pts',(41.5998344743201,-4.62875167249049,-9.68915746990398));
#62892=CARTESIAN_POINT('Ctrl Pts',(41.6009546848394,-4.63020113705926,-9.67186642585032));
#62893=CARTESIAN_POINT('Ctrl Pts',(41.6031524725772,-4.6336282191167,-9.63112371557899));
#62894=CARTESIAN_POINT('Ctrl Pts',(41.6040736937177,-4.63561052642731,-9.60766583750798));
#62895=CARTESIAN_POINT('Ctrl Pts',(41.6058019721924,-4.64157261216605,-9.53746364425242));
#62896=CARTESIAN_POINT('Ctrl Pts',(41.6055897198507,-4.64558295179576,-9.49070826565345));
#62897=CARTESIAN_POINT('Ctrl Pts',(41.6018940251512,-4.65509067382821,-9.38103369510855));
#62898=CARTESIAN_POINT('Ctrl Pts',(41.5973003456823,-4.66061709172731,-9.31818874583957));
#62899=CARTESIAN_POINT('Ctrl Pts',(41.5790538141281,-4.67505029371285,-9.15629572517049));
#62900=CARTESIAN_POINT('Ctrl Pts',(41.5616841746118,-4.68402822547005,-9.05778999729089));
#62901=CARTESIAN_POINT('Ctrl Pts',(41.5101155328111,-4.70377987384432,-8.84412573069977));
#62902=CARTESIAN_POINT('Ctrl Pts',(41.4733146077423,-4.71453011837482,-8.72984507182877));
#62903=CARTESIAN_POINT('Ctrl Pts',(41.4203489949477,-4.72671357120512,-8.59961851977961));
#62904=CARTESIAN_POINT('Ctrl Pts',(41.4123112988146,-4.72849422096922,-8.58056400502867));
#62905=CARTESIAN_POINT('Ctrl Pts',(41.3992114667894,-4.73128922753371,-8.5505942740487));
#62906=CARTESIAN_POINT('Ctrl Pts',(41.3943117289174,-4.73231241989635,-8.53960989943921));
#62907=CARTESIAN_POINT('Ctrl Pts',(41.3847024096533,-4.73427633109521,-8.51849459985349));
#62908=CARTESIAN_POINT('Ctrl Pts',(41.3800043490762,-4.7352176243638,-8.50835906737563));
#62909=CARTESIAN_POINT('Ctrl Pts',(41.3681573826961,-4.73754590696035,-8.48326035263044));
#62910=CARTESIAN_POINT('Ctrl Pts',(41.3609238339825,-4.73892791427912,-8.46833725327713));
#62911=CARTESIAN_POINT('Ctrl Pts',(41.331869824326,-4.74433121611485,-8.40994411295681));
#62912=CARTESIAN_POINT('Ctrl Pts',(41.3088855035372,-4.74828964392965,-8.36706155623103));
#62913=CARTESIAN_POINT('Ctrl Pts',(41.1672900725772,-4.77111524213714,-8.12110519626352));
#62914=CARTESIAN_POINT('Ctrl Pts',(41.0207138722834,-4.78894811431386,-7.93560725214195));
#62915=CARTESIAN_POINT('Ctrl Pts',(40.811969595921,-4.81202067723423,-7.7389229671705));
#62916=CARTESIAN_POINT('Ctrl Pts',(40.7732758317323,-4.81621252134748,-7.70474739205083));
#62917=CARTESIAN_POINT('Ctrl Pts',(40.7147596743687,-4.82245539356396,-7.65632433428605));
#62918=CARTESIAN_POINT('Ctrl Pts',(40.6957700971007,-4.82446706209007,-7.64108987935604));
#62919=CARTESIAN_POINT('Ctrl Pts',(40.6613613997418,-4.82808942084773,-7.61433358509546));
#62920=CARTESIAN_POINT('Ctrl Pts',(40.6460287923643,-4.82969570512639,-7.60270346307054));
#62921=CARTESIAN_POINT('Ctrl Pts',(40.612948656071,-4.83314584986249,-7.57823117003711));
#62922=CARTESIAN_POINT('Ctrl Pts',(40.5951620646422,-4.83499167404586,-7.56544506908707));
#62923=CARTESIAN_POINT('Ctrl Pts',(40.5455164226411,-4.84012022623625,-7.53077526693075));
#62924=CARTESIAN_POINT('Ctrl Pts',(40.5133022234595,-4.84342195938408,-7.50941481727415));
#62925=CARTESIAN_POINT('Ctrl Pts',(40.3704926554486,-4.85795708181521,-7.41959844697226));
#62926=CARTESIAN_POINT('Ctrl Pts',(40.2549807598847,-4.86947029226611,-7.35941154830786));
#62927=CARTESIAN_POINT('Ctrl Pts',(39.9934437539558,-4.89491209466127,-7.24904518125998));
#62928=CARTESIAN_POINT('Ctrl Pts',(39.846276212584,-4.90884573141768,-7.202962795462));
#62929=CARTESIAN_POINT('Ctrl Pts',(39.6681453080884,-4.92473587916687,-7.16544787544363));
#62930=CARTESIAN_POINT('Ctrl Pts',(39.6404824135889,-4.92717564696432,-7.16012754913506));
#62931=CARTESIAN_POINT('Ctrl Pts',(39.5993983104324,-4.93075220465543,-7.152971948227));
#62932=CARTESIAN_POINT('Ctrl Pts',(39.586046079463,-4.93190728298411,-7.15076232438096));
#62933=CARTESIAN_POINT('Ctrl Pts',(39.5619653031494,-4.93397654154886,-7.14698578818419));
#62934=CARTESIAN_POINT('Ctrl Pts',(39.5512440914666,-4.93489278253082,-7.14537858598069));
#62935=CARTESIAN_POINT('Ctrl Pts',(39.5267198560311,-4.93697733938558,-7.1418715555689));
#62936=CARTESIAN_POINT('Ctrl Pts',(39.5129106971364,-4.93814306941781,-7.14001908354762));
#62937=CARTESIAN_POINT('Ctrl Pts',(39.4689617319374,-4.941829873964,-7.13451171623176));
#62938=CARTESIAN_POINT('Ctrl Pts',(39.4387668859735,-4.94432819959118,-7.13130718789372));
#62939=CARTESIAN_POINT('Ctrl Pts',(39.365146423466,-4.95035361701698,-7.12490106727131));
#62940=CARTESIAN_POINT('Ctrl Pts',(39.3216778229234,-4.95385571865512,-7.1223049965251));
#62941=CARTESIAN_POINT('Ctrl Pts',(39.1245985597038,-4.96958066501487,-7.11589777760175));
#62942=CARTESIAN_POINT('Ctrl Pts',(38.970905686005,-4.98144414186177,-7.12562927223598));
#62943=CARTESIAN_POINT('Ctrl Pts',(38.7217970732718,-5.00135344755902,-7.16557146069848));
#62944=CARTESIAN_POINT('Ctrl Pts',(38.6254742698223,-5.00922042062027,-7.18715970774608));
#62945=CARTESIAN_POINT('Ctrl Pts',(38.501276458948,-5.01977662080017,-7.22313545468633));
#62946=CARTESIAN_POINT('Ctrl Pts',(38.4719634357677,-5.02229860799912,-7.23223800610766));
#62947=CARTESIAN_POINT('Ctrl Pts',(38.4235834731627,-5.02651704906705,-7.24828270131149));
#62948=CARTESIAN_POINT('Ctrl Pts',(38.4044151946945,-5.02820321309416,-7.25490990348813));
#62949=CARTESIAN_POINT('Ctrl Pts',(38.3666689297738,-5.03155443799323,-7.26849700187981));
#62950=CARTESIAN_POINT('Ctrl Pts',(38.348088689092,-5.03321902216912,-7.27544592838382));
#62951=CARTESIAN_POINT('Ctrl Pts',(38.3031430452642,-5.03728355112441,-7.29289207140762));
#62952=CARTESIAN_POINT('Ctrl Pts',(38.2768740375155,-5.0396911963857,-7.30362733621964));
#62953=CARTESIAN_POINT('Ctrl Pts',(38.1768930945831,-5.04898322311293,-7.34656586147726));
#62954=CARTESIAN_POINT('Ctrl Pts',(38.1046323412267,-5.05597253412571,-7.38199052181724));
#62955=CARTESIAN_POINT('Ctrl Pts',(37.8991843539477,-5.0766757088816,-7.49581594495521));
#62956=CARTESIAN_POINT('Ctrl Pts',(37.7716121605515,-5.09063484665905,-7.58350344839258));
#62957=CARTESIAN_POINT('Ctrl Pts',(37.5893836504235,-5.11192937486515,-7.73649729246795));
#62958=CARTESIAN_POINT('Ctrl Pts',(37.5282573426784,-5.1193421076161,-7.7934957793787));
#62959=CARTESIAN_POINT('Ctrl Pts',(37.456478262848,-5.12828472555001,-7.86778075301754));
#62960=CARTESIAN_POINT('Ctrl Pts',(37.4429177273388,-5.12998541335302,-7.88216536275201));
#62961=CARTESIAN_POINT('Ctrl Pts',(37.4215261642184,-5.13268424704774,-7.9054248249398));
#62962=CARTESIAN_POINT('Ctrl Pts',(37.4135810143153,-5.13369027154547,-7.9141926997654));
#62963=CARTESIAN_POINT('Ctrl Pts',(37.3981832076199,-5.13564653529233,-7.9314390199572));
#62964=CARTESIAN_POINT('Ctrl Pts',(37.3907250121288,-5.13659712412946,-7.9399118701817));
#62965=CARTESIAN_POINT('Ctrl Pts',(37.3831467253694,-5.13756653716907,-7.94864433006089));
#62966=CARTESIAN_POINT('Ctrl Pts',(37.3829669224932,-5.13758953956821,-7.94885158854521));
#62967=CARTESIAN_POINT('Ctrl Pts',(37.382607045393,-5.13763558319315,-7.94926656171896));
#62968=CARTESIAN_POINT('Ctrl Pts',(37.3824269712959,-5.13765862441054,-7.94947427653505));
#62969=CARTESIAN_POINT('Ctrl Pts',(37.3820663591634,-5.13770477035167,-7.94989038542191));
#62970=CARTESIAN_POINT('Ctrl Pts',(37.3818858213655,-5.1377278750573,-7.9500987796467));
#62971=CARTESIAN_POINT('Ctrl Pts',(37.381524090612,-5.13777417249707,-7.95051646943799));
#62972=CARTESIAN_POINT('Ctrl Pts',(37.3813428979343,-5.1377973652125,-7.95072576526779));
#62973=CARTESIAN_POINT('Ctrl Pts',(37.3809796666208,-5.13784386315861,-7.95114548049473));
#62974=CARTESIAN_POINT('Ctrl Pts',(37.38079762837,-5.13786716836146,-7.95135590018896));
#62975=CARTESIAN_POINT('Ctrl Pts',(37.3804325149379,-5.13791391580972,-7.95177808619828));
#62976=CARTESIAN_POINT('Ctrl Pts',(37.3802494402194,-5.13793735802204,-7.95198985288091));
#62977=CARTESIAN_POINT('Ctrl Pts',(37.3798820620862,-5.13798440413703,-7.95241495747763));
#62978=CARTESIAN_POINT('Ctrl Pts',(37.3796977591661,-5.13800800800739,-7.95262829588671));
#62979=CARTESIAN_POINT('Ctrl Pts',(37.3793277311396,-5.13805540232662,-7.95305677119684));
#62980=CARTESIAN_POINT('Ctrl Pts',(37.3791420066629,-5.13807919273088,-7.95327190860566));
#62981=CARTESIAN_POINT('Ctrl Pts',(37.37876893984,-5.1381269853071,-7.9537042123882));
#62982=CARTESIAN_POINT('Ctrl Pts',(37.378581598213,-5.13815098742822,-7.95392137934151));
#62983=CARTESIAN_POINT('Ctrl Pts',(37.378205098543,-5.13819922901521,-7.95435797670007));
#62984=CARTESIAN_POINT('Ctrl Pts',(37.3780159412777,-5.13822346842822,-7.95457740779998));
#62985=CARTESIAN_POINT('Ctrl Pts',(37.3776356081895,-5.13827221065856,-7.95501877283076));
#62986=CARTESIAN_POINT('Ctrl Pts',(37.3774444332266,-5.13829671341825,-7.95524070755223));
#62987=CARTESIAN_POINT('Ctrl Pts',(37.3770598582648,-5.13834600898041,-7.95568732499344));
#62988=CARTESIAN_POINT('Ctrl Pts',(37.376866459262,-5.13837080171387,-7.95591200854696));
#62989=CARTESIAN_POINT('Ctrl Pts',(37.3764772248428,-5.13842070451432,-7.95636437530127));
#62990=CARTESIAN_POINT('Ctrl Pts',(37.3762813905294,-5.13844581450502,-7.95659205942394));
#62991=CARTESIAN_POINT('Ctrl Pts',(37.3758870684821,-5.13849637985814,-7.95705068634192));
#62992=CARTESIAN_POINT('Ctrl Pts',(37.3756885819548,-5.13852183513785,-7.95728163016382));
#62993=CARTESIAN_POINT('Ctrl Pts',(37.375288732162,-5.1385731199437,-7.95774704372643));
#62994=CARTESIAN_POINT('Ctrl Pts',(37.3750873701966,-5.1385989493825,-7.9579815146248));
#62995=CARTESIAN_POINT('Ctrl Pts',(37.374681539083,-5.13865101232452,-7.95845425881746));
#62996=CARTESIAN_POINT('Ctrl Pts',(37.374477071377,-5.13867724573001,-7.95869253335952));
#62997=CARTESIAN_POINT('Ctrl Pts',(37.3740647904667,-5.13873014746429,-7.95917317148005));
#62998=CARTESIAN_POINT('Ctrl Pts',(37.3738569788701,-5.13875681568255,-7.95941553638736));
#62999=CARTESIAN_POINT('Ctrl Pts',(37.3734377633411,-5.13881061902815,-7.95990465287597));
#63000=CARTESIAN_POINT('Ctrl Pts',(37.3732263611292,-5.13883775403959,-7.96015140594851));
#63001=CARTESIAN_POINT('Ctrl Pts',(37.3727997081077,-5.1388925242028,-7.96064960853773));
#63002=CARTESIAN_POINT('Ctrl Pts',(37.3725844591586,-5.13892015923054,-7.96090105969881));
#63003=CARTESIAN_POINT('Ctrl Pts',(37.3723012094811,-5.13895652879637,-7.96123208675578));
#63004=CARTESIAN_POINT('Ctrl Pts',(37.3722331622188,-5.13896526645575,-7.96131162245678));
#63005=CARTESIAN_POINT('Ctrl Pts',(37.3720947385011,-5.13898304150204,-7.96147343767126));
#63006=CARTESIAN_POINT('Ctrl Pts',(37.3720243623906,-5.13899207886688,-7.96155571751681));
#63007=CARTESIAN_POINT('Ctrl Pts',(37.371881134098,-5.13901047225392,-7.96172319498457));
#63008=CARTESIAN_POINT('Ctrl Pts',(37.3718082822899,-5.13901982825256,-7.96180839297852));
#63009=CARTESIAN_POINT('Ctrl Pts',(37.3716599441049,-5.13903887933764,-7.96198189456902));
#63010=CARTESIAN_POINT('Ctrl Pts',(37.3715844581852,-5.13904857439234,-7.96207019852269));
#63011=CARTESIAN_POINT('Ctrl Pts',(37.3714306807572,-5.13906832563774,-7.96225011481478));
#63012=CARTESIAN_POINT('Ctrl Pts',(37.3713523897163,-5.13907838179826,-7.9623417275917));
#63013=CARTESIAN_POINT('Ctrl Pts',(37.3711928169677,-5.13909887911991,-7.96252848110824));
#63014=CARTESIAN_POINT('Ctrl Pts',(37.3711115358281,-5.13910932024114,-7.96262362227367));
#63015=CARTESIAN_POINT('Ctrl Pts',(37.3709457826479,-5.13913061330774,-7.96281767027519));
#63016=CARTESIAN_POINT('Ctrl Pts',(37.3708613111888,-5.13914146521513,-7.96291657763994));
#63017=CARTESIAN_POINT('Ctrl Pts',(37.3706889600457,-5.13916360788668,-7.96311841619834));
#63018=CARTESIAN_POINT('Ctrl Pts',(37.370601081077,-5.13917489859979,-7.96322134789813));
#63019=CARTESIAN_POINT('Ctrl Pts',(37.3704216791747,-5.13919794929695,-7.96343151535327));
#63020=CARTESIAN_POINT('Ctrl Pts',(37.3703301569516,-5.13920970923524,-7.96353875177282));
#63021=CARTESIAN_POINT('Ctrl Pts',(37.3701432120181,-5.13923373148482,-7.96375783380939));
#63022=CARTESIAN_POINT('Ctrl Pts',(37.3700477901319,-5.13924599374111,-7.96386968013115));
#63023=CARTESIAN_POINT('Ctrl Pts',(37.3698527665755,-5.13927105667535,-7.96409831445133));
#63024=CARTESIAN_POINT('Ctrl Pts',(37.3697531658085,-5.13928385729427,-7.96421510325992));
#63025=CARTESIAN_POINT('Ctrl Pts',(37.3695494798791,-5.1393100362787,-7.96445398544944));
#63026=CARTESIAN_POINT('Ctrl Pts',(37.3694453957187,-5.13932341457948,-7.96457607975107));
#63027=CARTESIAN_POINT('Ctrl Pts',(37.3692324101243,-5.13935079191195,-7.96482596981878));
#63028=CARTESIAN_POINT('Ctrl Pts',(37.3691235098844,-5.13936479086227,-7.96495376653987));
#63029=CARTESIAN_POINT('Ctrl Pts',(37.3689005280116,-5.13939345652417,-7.9652154959622));
#63030=CARTESIAN_POINT('Ctrl Pts',(37.3687864477202,-5.13940812314472,-7.9653494297442));
#63031=CARTESIAN_POINT('Ctrl Pts',(37.3685527067653,-5.13943817569377,-7.96562390983597));
#63032=CARTESIAN_POINT('Ctrl Pts',(37.3684330475777,-5.13945356152467,-7.96576445741302));
#63033=CARTESIAN_POINT('Ctrl Pts',(37.3681877109628,-5.13948510908146,-7.96605268859481));
#63034=CARTESIAN_POINT('Ctrl Pts',(37.3680620351538,-5.1395012707038,-7.96620037369759));
#63035=CARTESIAN_POINT('Ctrl Pts',(37.3678041836314,-5.13953443210911,-7.96650345637212));
#63036=CARTESIAN_POINT('Ctrl Pts',(37.3676720098507,-5.13955143176251,-7.96665885553446));
#63037=CARTESIAN_POINT('Ctrl Pts',(37.3674006321143,-5.13958633780094,-7.96697800162658));
#63038=CARTESIAN_POINT('Ctrl Pts',(37.3672614303116,-5.13960424404488,-7.96714175042555));
#63039=CARTESIAN_POINT('Ctrl Pts',(37.3669754114797,-5.13964103894506,-7.96747829752053));
#63040=CARTESIAN_POINT('Ctrl Pts',(37.3668285969074,-5.1396599274408,-7.96765109795586));
#63041=CARTESIAN_POINT('Ctrl Pts',(37.366526705891,-5.13969877052325,-7.96800652487232));
#63042=CARTESIAN_POINT('Ctrl Pts',(37.3663716323022,-5.13971872492129,-7.9681891537585));
#63043=CARTESIAN_POINT('Ctrl Pts',(37.3660525074491,-5.13975979247258,-7.96856509829356));
#63044=CARTESIAN_POINT('Ctrl Pts',(37.3658884594421,-5.13978090541262,-7.96875841673723));
#63045=CARTESIAN_POINT('Ctrl Pts',(37.3655505918557,-5.13982439286459,-7.96915669632795));
#63046=CARTESIAN_POINT('Ctrl Pts',(37.3653767760338,-5.13984676713109,-7.96936166069798));
#63047=CARTESIAN_POINT('Ctrl Pts',(37.3650184907207,-5.13989289152661,-7.96978429585711));
#63048=CARTESIAN_POINT('Ctrl Pts',(37.3648340256011,-5.13991664136932,-7.97000197034912));
#63049=CARTESIAN_POINT('Ctrl Pts',(37.3644534599163,-5.13996564418464,-7.97045121155202));
#63050=CARTESIAN_POINT('Ctrl Pts',(37.3642573644202,-5.13999089682653,-7.97068278257198));
#63051=CARTESIAN_POINT('Ctrl Pts',(37.3638524433131,-5.14004304721613,-7.97116114124246));
#63052=CARTESIAN_POINT('Ctrl Pts',(37.3636436235842,-5.14006994458271,-7.97140793394487));
#63053=CARTESIAN_POINT('Ctrl Pts',(37.3632120311691,-5.14012554311096,-7.97191821818251));
#63054=CARTESIAN_POINT('Ctrl Pts',(37.3629892653949,-5.14015424382399,-7.97218171558891));
#63055=CARTESIAN_POINT('Ctrl Pts',(37.3625284125873,-5.14021362672004,-7.97272707104065));
#63056=CARTESIAN_POINT('Ctrl Pts',(37.3622903336792,-5.14024430837654,-7.97300893596624));
#63057=CARTESIAN_POINT('Ctrl Pts',(37.3617973209124,-5.14030785244359,-7.97359289313026));
#63058=CARTESIAN_POINT('Ctrl Pts',(37.3615423966214,-5.14034071423669,-7.97389499348669));
#63059=CARTESIAN_POINT('Ctrl Pts',(37.3610139712229,-5.14040884247556,-7.97452152210394));
#63060=CARTESIAN_POINT('Ctrl Pts',(37.360740481402,-5.14044410819761,-7.97484596000798));
#63061=CARTESIAN_POINT('Ctrl Pts',(37.3601729885504,-5.14051729629013,-7.97551953201326));
#63062=CARTESIAN_POINT('Ctrl Pts',(37.3598789989865,-5.14055521779636,-7.97586867749637));
#63063=CARTESIAN_POINT('Ctrl Pts',(37.3363556790367,-5.14358999101517,-8.003821395009));
#63064=CARTESIAN_POINT('Ctrl Pts',(37.3137483572184,-5.14654695197108,-8.03194619825229));
#63065=CARTESIAN_POINT('Ctrl Pts',(37.2782077345349,-5.15128300733771,-8.07825729478609));
#63066=CARTESIAN_POINT('Ctrl Pts',(37.2648808648161,-5.15308014992894,-8.0961319256744));
#63067=CARTESIAN_POINT('Ctrl Pts',(37.1901355122883,-5.16329997089006,-8.19934822840204));
#63068=CARTESIAN_POINT('Ctrl Pts',(37.1341120226287,-5.17152014443217,-8.28846522314088));
#63069=CARTESIAN_POINT('Ctrl Pts',(37.0364096980596,-5.18761099129585,-8.46916717581044));
#63070=CARTESIAN_POINT('Ctrl Pts',(36.9943077805397,-5.19546105951395,-8.56021608581399));
#63071=CARTESIAN_POINT('Ctrl Pts',(36.9580195978366,-5.20345233470371,-8.65357770242256));
#63072=CARTESIAN_POINT('Origin',(39.2,8.05522481984854,-9.525));
#63073=CARTESIAN_POINT('',(36.9580196851476,-6.73822005631196,-8.65357747779021));
#63074=CARTESIAN_POINT('',(36.9596139210734,-6.47468182945015,-8.65421859155223));
#63075=CARTESIAN_POINT('',(36.958019684865,8.05522481984854,-8.65357747851728));
#63076=CARTESIAN_POINT('Ctrl Pts',(36.9580196851476,-6.73822005631196,-8.65357747779021));
#63077=CARTESIAN_POINT('Ctrl Pts',(36.9617632876953,-6.73732493420928,-8.64394600395906));
#63078=CARTESIAN_POINT('Ctrl Pts',(36.9655691048304,-6.7364326449218,-8.63433826822591));
#63079=CARTESIAN_POINT('Ctrl Pts',(36.9751700656461,-6.73422539355429,-8.61054969304967));
#63080=CARTESIAN_POINT('Ctrl Pts',(36.9810390153733,-6.73291421589457,-8.59639901597012));
#63081=CARTESIAN_POINT('Ctrl Pts',(36.9913409806347,-6.73067762730601,-8.57221537059667));
#63082=CARTESIAN_POINT('Ctrl Pts',(36.995708044588,-6.72974852321965,-8.56215514665832));
#63083=CARTESIAN_POINT('Ctrl Pts',(37.0052308720689,-6.72776294903167,-8.5406222281924));
#63084=CARTESIAN_POINT('Ctrl Pts',(37.0104080080805,-6.72670774970838,-8.52915962448612));
#63085=CARTESIAN_POINT('Ctrl Pts',(37.02515821817,-6.72376667044422,-8.49717266876666));
#63086=CARTESIAN_POINT('Ctrl Pts',(37.0349319176222,-6.72189216412974,-8.47674139129352));
#63087=CARTESIAN_POINT('Ctrl Pts',(37.1161897070929,-6.70686484166701,-8.31286408263086));
#63088=CARTESIAN_POINT('Ctrl Pts',(37.2015708021965,-6.69441356220162,-8.1767281771791));
#63089=CARTESIAN_POINT('Ctrl Pts',(37.3755072074582,-6.67218516050087,-7.95264745657533));
#63090=CARTESIAN_POINT('Ctrl Pts',(37.458511783565,-6.66248933493119,-7.86118509309098));
#63091=CARTESIAN_POINT('Ctrl Pts',(37.5708004800093,-6.65000379136199,-7.75510388194618));
#63092=CARTESIAN_POINT('Ctrl Pts',(37.5938571623798,-6.64747059549469,-7.73415428826679));
#63093=CARTESIAN_POINT('Ctrl Pts',(37.6333013925827,-6.64318109659655,-7.69968928695764));
#63094=CARTESIAN_POINT('Ctrl Pts',(37.6494733214651,-6.6414344333673,-7.68593211455313));
#63095=CARTESIAN_POINT('Ctrl Pts',(37.6671808776097,-6.63953370052731,-7.67126820095321));
#63096=CARTESIAN_POINT('Ctrl Pts',(37.6685382520381,-6.63938807380186,-7.67014664750604));
#63097=CARTESIAN_POINT('Ctrl Pts',(37.6712600756542,-6.63909620868146,-7.66790271941159));
#63098=CARTESIAN_POINT('Ctrl Pts',(37.6726245323447,-6.63894996998278,-7.66678035565537));
#63099=CARTESIAN_POINT('Ctrl Pts',(37.6754466796612,-6.63864765171348,-7.66446414493327));
#63100=CARTESIAN_POINT('Ctrl Pts',(37.6769045384281,-6.63849156420354,-7.66327050583539));
#63101=CARTESIAN_POINT('Ctrl Pts',(37.6800493630152,-6.63815503779881,-7.66070180974682));
#63102=CARTESIAN_POINT('Ctrl Pts',(37.6817367941519,-6.63797457672905,-7.65932732807841));
#63103=CARTESIAN_POINT('Ctrl Pts',(37.6976120293693,-6.63627783768494,-7.64643210085669));
#63104=CARTESIAN_POINT('Ctrl Pts',(37.7119284223306,-6.63475539226718,-7.63507145452685));
#63105=CARTESIAN_POINT('Ctrl Pts',(37.7425622002386,-6.63151278937312,-7.61132615255223));
#63106=CARTESIAN_POINT('Ctrl Pts',(37.7589110164648,-6.62979110882047,-7.59898467800878));
#63107=CARTESIAN_POINT('Ctrl Pts',(37.8009451972879,-6.62538535777805,-7.56808852067323));
#63108=CARTESIAN_POINT('Ctrl Pts',(37.8268423927752,-6.62269033423657,-7.54983042274668));
#63109=CARTESIAN_POINT('Ctrl Pts',(37.9458759828876,-6.61038255860204,-7.46938154361071));
#63110=CARTESIAN_POINT('Ctrl Pts',(38.0429106479893,-6.60055645517692,-7.41323989339178));
#63111=CARTESIAN_POINT('Ctrl Pts',(38.2701190271191,-6.57802028181283,-7.30215426009766));
#63112=CARTESIAN_POINT('Ctrl Pts',(38.4019433277125,-6.56525751550808,-7.25149479849223));
#63113=CARTESIAN_POINT('Ctrl Pts',(38.5969246568206,-6.54721870987632,-7.19562633303788));
#63114=CARTESIAN_POINT('Ctrl Pts',(38.6570490389488,-6.54176914670581,-7.18088236616085));
#63115=CARTESIAN_POINT('Ctrl Pts',(38.7352459054524,-6.53487509170483,-7.16487754279157));
#63116=CARTESIAN_POINT('Ctrl Pts',(38.7528509064137,-6.53333551884981,-7.16147887068167));
#63117=CARTESIAN_POINT('Ctrl Pts',(38.7817487065672,-6.53083055211108,-7.15623457009995));
#63118=CARTESIAN_POINT('Ctrl Pts',(38.7930192020985,-6.52985908382715,-7.15427216741645));
#63119=CARTESIAN_POINT('Ctrl Pts',(38.8157844488211,-6.52790844759465,-7.15047545210971));
#63120=CARTESIAN_POINT('Ctrl Pts',(38.8272793278231,-6.52692945011543,-7.14864402147418));
#63121=CARTESIAN_POINT('Ctrl Pts',(38.8574383659131,-6.52437529971452,-7.14406313519393));
#63122=CARTESIAN_POINT('Ctrl Pts',(38.8761228817015,-6.52280737414565,-7.14144960032692));
#63123=CARTESIAN_POINT('Ctrl Pts',(38.9611921081414,-6.51572612648478,-7.13056922250495));
#63124=CARTESIAN_POINT('Ctrl Pts',(39.0278803730816,-6.51033316904641,-7.12485314492138));
#63125=CARTESIAN_POINT('Ctrl Pts',(39.2443969461397,-6.49307836567454,-7.11536813755116));
#63126=CARTESIAN_POINT('Ctrl Pts',(39.3943568228586,-6.48150273421907,-7.12280796894516));
#63127=CARTESIAN_POINT('Ctrl Pts',(39.6410462369733,-6.46183336385126,-7.1583119504988));
#63128=CARTESIAN_POINT('Ctrl Pts',(39.7384518990124,-6.45390307346302,-7.17855598356188));
#63129=CARTESIAN_POINT('Ctrl Pts',(39.8634263135476,-6.44332082728093,-7.21272208856444));
#63130=CARTESIAN_POINT('Ctrl Pts',(39.8923816996738,-6.44084021023864,-7.22122678394347));
#63131=CARTESIAN_POINT('Ctrl Pts',(39.940422740592,-6.43667142025576,-7.23632473577453));
#63132=CARTESIAN_POINT('Ctrl Pts',(39.9595997632192,-6.43499301680374,-7.24261781295982));
#63133=CARTESIAN_POINT('Ctrl Pts',(39.9973266423046,-6.43166134067247,-7.2555262814895));
#63134=CARTESIAN_POINT('Ctrl Pts',(40.0158789603609,-6.43000857575912,-7.26212965322686));
#63135=CARTESIAN_POINT('Ctrl Pts',(40.0569160058768,-6.42631939660508,-7.27730631477722));
#63136=CARTESIAN_POINT('Ctrl Pts',(40.0793570539079,-6.42427947064588,-7.28599061523573));
#63137=CARTESIAN_POINT('Ctrl Pts',(40.1594038099944,-6.41691922974186,-7.31835632365124));
#63138=CARTESIAN_POINT('Ctrl Pts',(40.21620989349,-6.41153757785529,-7.34393421720117));
#63139=CARTESIAN_POINT('Ctrl Pts',(40.4384415418904,-6.38982333259559,-7.45456465709944));
#63140=CARTESIAN_POINT('Ctrl Pts',(40.5947397533889,-6.37298054649957,-7.55646688203441));
#63141=CARTESIAN_POINT('Ctrl Pts',(40.7771573655121,-6.35179173635574,-7.70811837674365));
#63142=CARTESIAN_POINT('Ctrl Pts',(40.815546189843,-6.34723783469156,-7.74216645793597));
#63143=CARTESIAN_POINT('Ctrl Pts',(40.8775942195695,-6.33974907837542,-7.80084994513031));
#63144=CARTESIAN_POINT('Ctrl Pts',(40.9018699802078,-6.33678419194224,-7.82480745270185));
#63145=CARTESIAN_POINT('Ctrl Pts',(40.9357801864565,-6.33260135466889,-7.85972753655362));
#63146=CARTESIAN_POINT('Ctrl Pts',(40.9458357920986,-6.33135560774718,-7.87027263471603));
#63147=CARTESIAN_POINT('Ctrl Pts',(40.9632327349762,-6.32919185155013,-7.88885157513314));
#63148=CARTESIAN_POINT('Ctrl Pts',(40.9706162556708,-6.32827082573229,-7.89684477377029));
#63149=CARTESIAN_POINT('Ctrl Pts',(40.9867227172739,-6.32625584533185,-7.9145203552941));
#63150=CARTESIAN_POINT('Ctrl Pts',(40.9954215500755,-6.32516362084392,-7.92422386441594));
#63151=CARTESIAN_POINT('Ctrl Pts',(41.0209337916485,-6.32194669716284,-7.95315226187664));
#63152=CARTESIAN_POINT('Ctrl Pts',(41.0375210865199,-6.31983732708361,-7.97257557323292));
#63153=CARTESIAN_POINT('Ctrl Pts',(41.1329344721321,-6.30757115000303,-8.08797485831539));
#63154=CARTESIAN_POINT('Ctrl Pts',(41.2045525960589,-6.29781322727732,-8.1896891916301));
#63155=CARTESIAN_POINT('Ctrl Pts',(41.3311472018903,-6.27838567107459,-8.40279187484914));
#63156=CARTESIAN_POINT('Ctrl Pts',(41.3859998902747,-6.26874217145774,-8.51379226876584));
#63157=CARTESIAN_POINT('Ctrl Pts',(41.4486825380718,-6.2553053979647,-8.66985955813001));
#63158=CARTESIAN_POINT('Ctrl Pts',(41.4641361821291,-6.25171931273061,-8.71165797551311));
#63159=CARTESIAN_POINT('Ctrl Pts',(41.4900234305108,-6.2451573368809,-8.78814466990518));
#63160=CARTESIAN_POINT('Ctrl Pts',(41.5008514781816,-6.24219408799807,-8.82268576157862));
#63161=CARTESIAN_POINT('Ctrl Pts',(41.516836877065,-6.2374385119812,-8.87802383753787));
#63162=CARTESIAN_POINT('Ctrl Pts',(41.5225031421398,-6.23566256111774,-8.89866912647387));
#63163=CARTESIAN_POINT('Ctrl Pts',(41.5327626263355,-6.23226518490991,-8.93810514483334));
#63164=CARTESIAN_POINT('Ctrl Pts',(41.5374062426974,-6.23064551324529,-8.95688112868409));
#63165=CARTESIAN_POINT('Ctrl Pts',(41.5474859403931,-6.22693241201079,-8.99985458000316));
#63166=CARTESIAN_POINT('Ctrl Pts',(41.5527751291091,-6.22483451716637,-9.02408379408837));
#63167=CARTESIAN_POINT('Ctrl Pts',(41.5687678124529,-6.21796751208791,-9.10319612269222));
#63168=CARTESIAN_POINT('Ctrl Pts',(41.5779316196392,-6.21315158159198,-9.15836724187236));
#63169=CARTESIAN_POINT('Ctrl Pts',(41.6109195015664,-6.19093840323978,-9.41120223122716));
#63170=CARTESIAN_POINT('Ctrl Pts',(41.6120653831861,-6.17289934019233,-9.61101541992265));
#63171=CARTESIAN_POINT('Ctrl Pts',(41.5827176011395,-6.15068148692619,-9.85816223897083));
#63172=CARTESIAN_POINT('Ctrl Pts',(41.575297428387,-6.14625685843701,-9.90749584153287));
#63173=CARTESIAN_POINT('Ctrl Pts',(41.560349006788,-6.13895450013743,-9.98946046965122));
#63174=CARTESIAN_POINT('Ctrl Pts',(41.5536641906323,-6.13604844213904,-10.0222284901388));
#63175=CARTESIAN_POINT('Ctrl Pts',(41.5431122892356,-6.13193280231949,-10.0689548436887));
#63176=CARTESIAN_POINT('Ctrl Pts',(41.5397995474366,-6.13069657537435,-10.0830324204316));
#63177=CARTESIAN_POINT('Ctrl Pts',(41.5337741617397,-6.12854314511448,-10.1076399481452));
#63178=CARTESIAN_POINT('Ctrl Pts',(41.5311168162326,-6.12762302436337,-10.1181825649661));
#63179=CARTESIAN_POINT('Ctrl Pts',(41.5250978360649,-6.12560254477502,-10.1413966543453));
#63180=CARTESIAN_POINT('Ctrl Pts',(41.5217039906145,-6.1245039919606,-10.1540591287194));
#63181=CARTESIAN_POINT('Ctrl Pts',(41.5114994861476,-6.1213143061097,-10.1909243046892));
#63182=CARTESIAN_POINT('Ctrl Pts',(41.5044124112449,-6.11923777688948,-10.2150497405517));
#63183=CARTESIAN_POINT('Ctrl Pts',(41.4609714704746,-6.1072489642283,-10.3547879043515));
#63184=CARTESIAN_POINT('Ctrl Pts',(41.4162949157245,-6.09771662276638,-10.4676480982827));
#63185=CARTESIAN_POINT('Ctrl Pts',(41.3098505940253,-6.07862994592636,-10.6866042205433));
#63186=CARTESIAN_POINT('Ctrl Pts',(41.2481098308799,-6.06910124965959,-10.792295354218));
#63187=CARTESIAN_POINT('Ctrl Pts',(41.1396377229013,-6.05388472510908,-10.9492031649496));
#63188=CARTESIAN_POINT('Ctrl Pts',(41.0982809803045,-6.04835819458522,-11.003876891567));
#63189=CARTESIAN_POINT('Ctrl Pts',(41.0375021287759,-6.04053690080271,-11.0774703120498));
#63190=CARTESIAN_POINT('Ctrl Pts',(41.0200071030013,-6.0383173326261,-11.0979437909876));
#63191=CARTESIAN_POINT('Ctrl Pts',(40.9891986898125,-6.03445912854515,-11.1327949870413));
#63192=CARTESIAN_POINT('Ctrl Pts',(40.9760462450375,-6.03282717824222,-11.1473120414329));
#63193=CARTESIAN_POINT('Ctrl Pts',(40.9486326795084,-6.02945519070382,-11.1768369314884));
#63194=CARTESIAN_POINT('Ctrl Pts',(40.9343522206689,-6.02771442745515,-11.1918244698666));
#63195=CARTESIAN_POINT('Ctrl Pts',(40.8969815866578,-6.02319769938935,-11.2300452471005));
#63196=CARTESIAN_POINT('Ctrl Pts',(40.8736078931447,-6.02040965430334,-11.252993690112));
#63197=CARTESIAN_POINT('Ctrl Pts',(40.7504643489673,-6.00589956425235,-11.3690542873462));
#63198=CARTESIAN_POINT('Ctrl Pts',(40.6433889578231,-5.99385045387143,-11.4540129472089));
#63199=CARTESIAN_POINT('Ctrl Pts',(40.4271535582749,-5.9706093319988,-11.5974608473102));
#63200=CARTESIAN_POINT('Ctrl Pts',(40.3195244837418,-5.95948640846034,-11.6575257418319));
#63201=CARTESIAN_POINT('Ctrl Pts',(40.158227233283,-5.94373343670977,-11.7319504980944));
#63202=CARTESIAN_POINT('Ctrl Pts',(40.1079163080143,-5.93894207212785,-11.7531200883342));
#63203=CARTESIAN_POINT('Ctrl Pts',(40.0408195983243,-5.93274567540705,-11.7787019317493));
#63204=CARTESIAN_POINT('Ctrl Pts',(40.0246490200211,-5.93126682506256,-11.7846690113618));
#63205=CARTESIAN_POINT('Ctrl Pts',(39.9977743403617,-5.92883448782804,-11.794259061274));
#63206=CARTESIAN_POINT('Ctrl Pts',(39.987106631958,-5.92787556985234,-11.7979812488116));
#63207=CARTESIAN_POINT('Ctrl Pts',(39.9652223638526,-5.92592234557862,-11.8054445759096));
#63208=CARTESIAN_POINT('Ctrl Pts',(39.9540037628862,-5.92492845178307,-11.8091784243139));
#63209=CARTESIAN_POINT('Ctrl Pts',(39.9240024159592,-5.92228902496824,-11.8189185433317));
#63210=CARTESIAN_POINT('Ctrl Pts',(39.9051720203854,-5.92065161827214,-11.8247770067141));
#63211=CARTESIAN_POINT('Ctrl Pts',(39.807573326011,-5.9122531806656,-11.8538301123938));
#63212=CARTESIAN_POINT('Ctrl Pts',(39.7277170384287,-5.90567613948618,-11.8732149368493));
#63213=CARTESIAN_POINT('Ctrl Pts',(39.4941296177812,-5.88685949958672,-11.9173943922438));
#63214=CARTESIAN_POINT('Ctrl Pts',(39.3387995799375,-5.87484286204838,-11.9314079673804));
#63215=CARTESIAN_POINT('Ctrl Pts',(39.1025025399608,-5.85608414372925,-11.9297577765034));
#63216=CARTESIAN_POINT('Ctrl Pts',(39.0218909637995,-5.84960492601225,-11.9251334172715));
#63217=CARTESIAN_POINT('Ctrl Pts',(38.9134250808235,-5.84067886678781,-11.9134168210842));
#63218=CARTESIAN_POINT('Ctrl Pts',(38.8852365266294,-5.83834022655684,-11.9098655964751));
#63219=CARTESIAN_POINT('Ctrl Pts',(38.8374746602102,-5.83434157424136,-11.9029870085379));
#63220=CARTESIAN_POINT('Ctrl Pts',(38.8178670655835,-5.83268961730645,-11.8999149891599));
#63221=CARTESIAN_POINT('Ctrl Pts',(38.7806416173982,-5.82953228057051,-11.8936097753284));
#63222=CARTESIAN_POINT('Ctrl Pts',(38.7630173824434,-5.82802841888467,-11.8904217120192));
#63223=CARTESIAN_POINT('Ctrl Pts',(38.7217743692136,-5.82448702663994,-11.8824845806877));
#63224=CARTESIAN_POINT('Ctrl Pts',(38.6981885315037,-5.82244465002882,-11.8775769831172));
#63225=CARTESIAN_POINT('Ctrl Pts',(38.6135077247214,-5.81504723860042,-11.8586258023767));
#63226=CARTESIAN_POINT('Ctrl Pts',(38.5528991174626,-5.80962995434926,-11.8425507557642));
#63227=CARTESIAN_POINT('Ctrl Pts',(38.2869390602945,-5.78528680433578,-11.7607651565887));
#63228=CARTESIAN_POINT('Ctrl Pts',(38.0903467014128,-5.7656346295313,-11.6699875869335));
#63229=CARTESIAN_POINT('Ctrl Pts',(37.8661221209814,-5.74211087553907,-11.5272859424611));
#63230=CARTESIAN_POINT('Ctrl Pts',(37.8245713105267,-5.73770523398101,-11.49897469517));
#63231=CARTESIAN_POINT('Ctrl Pts',(37.7703770435447,-5.7319237744806,-11.4595057354295));
#63232=CARTESIAN_POINT('Ctrl Pts',(37.7569226576988,-5.73048547387496,-11.4494900808571));
#63233=CARTESIAN_POINT('Ctrl Pts',(37.7346535900901,-5.72810125882929,-11.4325477617431));
#63234=CARTESIAN_POINT('Ctrl Pts',(37.7257807868404,-5.72715033748417,-11.4256988975437));
#63235=CARTESIAN_POINT('Ctrl Pts',(37.7075338508162,-5.72519323776088,-11.4114095393946));
#63236=CARTESIAN_POINT('Ctrl Pts',(37.6981668410966,-5.72418764997645,-11.4039607071011));
#63237=CARTESIAN_POINT('Ctrl Pts',(37.6729915944048,-5.7214812436611,-11.3836322999105));
#63238=CARTESIAN_POINT('Ctrl Pts',(37.6572903968992,-5.71978928554687,-11.3706207254715));
#63239=CARTESIAN_POINT('Ctrl Pts',(37.5601887042316,-5.70928587629362,-11.2880474370306));
#63240=CARTESIAN_POINT('Ctrl Pts',(37.4833310081189,-5.70079253976512,-11.2133044670983));
#63241=CARTESIAN_POINT('Ctrl Pts',(37.3209233792285,-5.68169521221423,-11.0327626464593));
#63242=CARTESIAN_POINT('Ctrl Pts',(37.238853538038,-5.67116022287281,-10.9243499671334));
#63243=CARTESIAN_POINT('Ctrl Pts',(37.1389832251379,-5.65628667485469,-10.7662460920522));
#63244=CARTESIAN_POINT('Ctrl Pts',(37.1129949173773,-5.65217738587393,-10.7220343251728));
#63245=CARTESIAN_POINT('Ctrl Pts',(37.0691780535898,-5.64476468373186,-10.6417221478682));
#63246=CARTESIAN_POINT('Ctrl Pts',(37.0508052825954,-5.64147977256848,-10.6059404322621));
#63247=CARTESIAN_POINT('Ctrl Pts',(37.0236868419793,-5.63633210306697,-10.5496989172435));
#63248=CARTESIAN_POINT('Ctrl Pts',(37.0143128058653,-5.63449085519254,-10.5295487812455));
#63249=CARTESIAN_POINT('Ctrl Pts',(36.9973571311387,-5.63103982064296,-10.4917401578452));
#63250=CARTESIAN_POINT('Ctrl Pts',(36.9897052451479,-5.62943256572078,-10.4741149517957));
#63251=CARTESIAN_POINT('Ctrl Pts',(36.9730109495247,-5.62580986630952,-10.4343645820266));
#63252=CARTESIAN_POINT('Ctrl Pts',(36.9640856554668,-5.62379069445494,-10.4121928365886));
#63253=CARTESIAN_POINT('Ctrl Pts',(36.9418351655035,-5.61853378096758,-10.3544499571195));
#63254=CARTESIAN_POINT('Ctrl Pts',(36.9290200698861,-5.61527986165507,-10.3186910347625));
#63255=CARTESIAN_POINT('Ctrl Pts',(36.8586020307597,-5.59596973608905,-10.1065070297757));
#63256=CARTESIAN_POINT('Ctrl Pts',(36.8207380237783,-5.57930051890073,-9.92422533382003));
#63257=CARTESIAN_POINT('Ctrl Pts',(36.7977867859462,-5.55618743923678,-9.66781775090883));
#63258=CARTESIAN_POINT('Ctrl Pts',(36.7945903213438,-5.54975260958905,-9.59592895843203));
#63259=CARTESIAN_POINT('Ctrl Pts',(36.7946376502955,-5.53970999683671,-9.48202068814434));
#63260=CARTESIAN_POINT('Ctrl Pts',(36.7957540752139,-5.53604252743491,-9.44004474681283));
#63261=CARTESIAN_POINT('Ctrl Pts',(36.7988223204285,-5.53103101498072,-9.3819599937646));
#63262=CARTESIAN_POINT('Ctrl Pts',(36.799838757767,-5.52964461290738,-9.3658122241438));
#63263=CARTESIAN_POINT('Ctrl Pts',(36.8018192412762,-5.52733069010559,-9.33871311521891));
#63264=CARTESIAN_POINT('Ctrl Pts',(36.8026955466722,-5.52639861951119,-9.32775615125956));
#63265=CARTESIAN_POINT('Ctrl Pts',(36.8046979925372,-5.52444578697903,-9.30470772694864));
#63266=CARTESIAN_POINT('Ctrl Pts',(36.8058406255734,-5.5234259203755,-9.29261819697242));
#63267=CARTESIAN_POINT('Ctrl Pts',(36.8092307565423,-5.52063741178237,-9.25943385384409));
#63268=CARTESIAN_POINT('Ctrl Pts',(36.8116659024057,-5.51887856483244,-9.23835861012314));
#63269=CARTESIAN_POINT('Ctrl Pts',(36.8307047768568,-5.50662621036752,-9.09074056940703));
#63270=CARTESIAN_POINT('Ctrl Pts',(36.8570807199413,-5.49658439037482,-8.96564233949315));
#63271=CARTESIAN_POINT('Ctrl Pts',(36.9122212614242,-5.48133196633905,-8.77908232341413));
#63272=CARTESIAN_POINT('Ctrl Pts',(36.9338279612903,-5.4761097739669,-8.71581746937143));
#63273=CARTESIAN_POINT('Ctrl Pts',(36.9580198925264,-5.47085833376936,-8.65357694424991));
#63274=CARTESIAN_POINT('',(36.7953937665934,-5.27977575808644,-9.52712105355602));
#63275=CARTESIAN_POINT('Ctrl Pts',(36.9580195978366,-5.20345233470371,-8.65357770242256));
#63276=CARTESIAN_POINT('Ctrl Pts',(36.9423609402093,-5.20690063750865,-8.69386402929538));
#63277=CARTESIAN_POINT('Ctrl Pts',(36.9277847806697,-5.21037444878413,-8.73458104174594));
#63278=CARTESIAN_POINT('Ctrl Pts',(36.9022171597942,-5.21702892112913,-8.81257191891362));
#63279=CARTESIAN_POINT('Ctrl Pts',(36.8910202278685,-5.22020074035216,-8.84974313907366));
#63280=CARTESIAN_POINT('Ctrl Pts',(36.8748524133117,-5.22522801618809,-8.90853212764523));
#63281=CARTESIAN_POINT('Ctrl Pts',(36.8692724073146,-5.2270640211245,-8.9299766739618));
#63282=CARTESIAN_POINT('Ctrl Pts',(36.8594082182302,-5.23050993985417,-8.97015562393998));
#63283=CARTESIAN_POINT('Ctrl Pts',(36.8550507176876,-5.23211737822682,-8.98887036230359));
#63284=CARTESIAN_POINT('Ctrl Pts',(36.8469379765276,-5.23528696707361,-9.02570602778406));
#63285=CARTESIAN_POINT('Ctrl Pts',(36.8431667138616,-5.23684848821396,-9.04382209399185));
#63286=CARTESIAN_POINT('Ctrl Pts',(36.8350760192108,-5.2404105884101,-9.08506698208142));
#63287=CARTESIAN_POINT('Ctrl Pts',(36.830886252031,-5.24241506382615,-9.10821893009701));
#63288=CARTESIAN_POINT('Ctrl Pts',(36.8195276657382,-5.24836071037824,-9.17670319407919));
#63289=CARTESIAN_POINT('Ctrl Pts',(36.8133162770967,-5.2523302120571,-9.22218089056959));
#63290=CARTESIAN_POINT('Ctrl Pts',(36.7991452241016,-5.26389805224255,-9.35395403251787));
#63291=CARTESIAN_POINT('Ctrl Pts',(36.7945433759335,-5.27158206251985,-9.44052960809255));
#63292=CARTESIAN_POINT('Ctrl Pts',(36.794620964868,-5.27933234931437,-9.52715447146443));
#63293=CARTESIAN_POINT('Ctrl Pts',(36.7953937665934,-5.27977575808644,-9.52712105355602));
#63294=CARTESIAN_POINT('Ctrl Pts',(36.7935531956842,-5.2976235321573,-9.73963463083655));
#63295=CARTESIAN_POINT('Ctrl Pts',(36.9163459897307,-5.3823399067148,-10.7462609175526));
#63296=CARTESIAN_POINT('Ctrl Pts',(38.3249527608304,-5.53392488175899,-12.2249208567151));
#63297=CARTESIAN_POINT('Ctrl Pts',(40.9825464123629,-5.73453068321897,-11.733576145637));
#63298=CARTESIAN_POINT('Ctrl Pts',(42.0237943679678,-5.93513648467895,-9.23957808294332));
#63299=CARTESIAN_POINT('Ctrl Pts',(40.504532346838,-6.13574228613894,-7.00438982399976));
#63300=CARTESIAN_POINT('Ctrl Pts',(38.0819715177778,-6.31559073439599,-7.04957992665282));
#63301=CARTESIAN_POINT('Ctrl Pts',(37.1630963681982,-6.42857058216639,-8.14366218756688));
#63302=CARTESIAN_POINT('Ctrl Pts',(36.9596139210735,-6.47468182945012,-8.65421859155197));
#63303=CARTESIAN_POINT('Origin',(39.2,8.05522481984854,-9.525));
#63304=CARTESIAN_POINT('',(36.960685369651,-8.0104155729454,-8.65458630036363));
#63305=CARTESIAN_POINT('',(36.9580196848652,-7.74707540691375,-8.65357747851679));
#63306=CARTESIAN_POINT('',(36.958019684865,8.05522481984854,-8.65357747851728));
#63307=CARTESIAN_POINT('',(36.7979795612525,-6.81524146755324,-9.52396154577679));
#63308=CARTESIAN_POINT('Ctrl Pts',(36.7980085683911,-6.81522481984856,-9.52396299273671));
#63309=CARTESIAN_POINT('Ctrl Pts',(36.7998408421343,-6.85429379911921,-9.99043766253926));
#63310=CARTESIAN_POINT('Ctrl Pts',(37.155387877586,-6.96023137887653,-11.2578897609434));
#63311=CARTESIAN_POINT('Ctrl Pts',(39.2043913575984,-7.13303755912051,-12.363179688143));
#63312=CARTESIAN_POINT('Ctrl Pts',(41.5790395607839,-7.33364336058048,-11.0727254258319));
#63313=CARTESIAN_POINT('Ctrl Pts',(41.7964646321477,-7.53424916204047,-8.3788522608558));
#63314=CARTESIAN_POINT('Ctrl Pts',(39.6595137365683,-7.73485496350045,-6.72426253398319));
#63315=CARTESIAN_POINT('Ctrl Pts',(37.6390531498371,-7.89357710046876,-7.42449738893203));
#63316=CARTESIAN_POINT('Ctrl Pts',(37.0669560907077,-7.98543063695042,-8.37601688395995));
#63317=CARTESIAN_POINT('Ctrl Pts',(36.960685369651,-8.0104155729454,-8.65458630036363));
#63318=CARTESIAN_POINT('Ctrl Pts',(36.7946203023417,-6.81716940505584,-9.52379397623225));
#63319=CARTESIAN_POINT('Ctrl Pts',(36.7947236645737,-6.7994075675383,-9.31764097916309));
#63320=CARTESIAN_POINT('Ctrl Pts',(36.8213300094935,-6.78083055974931,-9.11238328777849));
#63321=CARTESIAN_POINT('Ctrl Pts',(36.8896249052172,-6.75676977471914,-8.85275714142221));
#63322=CARTESIAN_POINT('Ctrl Pts',(36.9078343242278,-6.75120685609406,-8.79307025277999));
#63323=CARTESIAN_POINT('Ctrl Pts',(36.9377559246244,-6.74320114444374,-8.70712224457528));
#63324=CARTESIAN_POINT('Ctrl Pts',(36.9476490838554,-6.7406997411387,-8.68025877573441));
#63325=CARTESIAN_POINT('Ctrl Pts',(36.9580196851476,-6.73822005631196,-8.65357747779021));
#63326=CARTESIAN_POINT('',(36.7912413910993,-6.54982113404641,-9.52410385179467));
#63327=CARTESIAN_POINT('Ctrl Pts',(36.9596139210735,-6.47468182945012,-8.65421859155197));
#63328=CARTESIAN_POINT('Ctrl Pts',(36.8680146416272,-6.49543918265305,-8.88404971154581));
#63329=CARTESIAN_POINT('Ctrl Pts',(36.7994752463598,-6.5204702995535,-9.17684559940756));
#63330=CARTESIAN_POINT('Ctrl Pts',(36.7909182968623,-6.54550141645394,-9.47345140065415));
#63331=CARTESIAN_POINT('Ctrl Pts',(36.7911611527837,-6.54977518015146,-9.52410755556446));
#63332=CARTESIAN_POINT('Ctrl Pts',(36.7946202300976,-6.55175625458268,-9.52394788588594));
#63333=CARTESIAN_POINT('Ctrl Pts',(36.7945192429906,-6.57057638584763,-9.7548281115921));
#63334=CARTESIAN_POINT('Ctrl Pts',(36.8276582622447,-6.58807846590248,-9.98456139645675));
#63335=CARTESIAN_POINT('Ctrl Pts',(36.913485047566,-6.61222119073305,-10.2752709658564));
#63336=CARTESIAN_POINT('Ctrl Pts',(36.9370116534691,-6.6180310435769,-10.3434980442765));
#63337=CARTESIAN_POINT('Ctrl Pts',(36.9736516944288,-6.62618226114725,-10.4360305520619));
#63338=CARTESIAN_POINT('Ctrl Pts',(36.9841714418198,-6.62843927809972,-10.4613263965217));
#63339=CARTESIAN_POINT('Ctrl Pts',(37.0029798955398,-6.63234105742448,-10.5044601804163));
#63340=CARTESIAN_POINT('Ctrl Pts',(37.0110597725077,-6.63397870689111,-10.5223866936633));
#63341=CARTESIAN_POINT('Ctrl Pts',(37.0280301087171,-6.63734300289247,-10.5588384282946));
#63342=CARTESIAN_POINT('Ctrl Pts',(37.0369399624873,-6.63907019712561,-10.5773527557263));
#63343=CARTESIAN_POINT('Ctrl Pts',(37.0603350133932,-6.64350943445977,-10.6244140992691));
#63344=CARTESIAN_POINT('Ctrl Pts',(37.0751544165008,-6.64623277238769,-10.6527892758816));
#63345=CARTESIAN_POINT('Ctrl Pts',(37.1489780264201,-6.65939761601173,-10.7875188140521));
#63346=CARTESIAN_POINT('Ctrl Pts',(37.2154157112662,-6.67009447107294,-10.8895733192653));
#63347=CARTESIAN_POINT('Ctrl Pts',(37.3698533729294,-6.69279948136676,-11.0915292819344));
#63348=CARTESIAN_POINT('Ctrl Pts',(37.4590132488357,-6.70480223993357,-11.1900572313959));
#63349=CARTESIAN_POINT('Ctrl Pts',(37.5856563622757,-6.72022330687607,-11.3086524542241));
#63350=CARTESIAN_POINT('Ctrl Pts',(37.6161800852135,-6.72382997238577,-11.3358109725625));
#63351=CARTESIAN_POINT('Ctrl Pts',(37.6630318637157,-6.7291881757941,-11.3754058195997));
#63352=CARTESIAN_POINT('Ctrl Pts',(37.6788501177488,-6.73096807486855,-11.3884312065346));
#63353=CARTESIAN_POINT('Ctrl Pts',(37.7072945431781,-6.73411471909965,-11.4112498687287));
#63354=CARTESIAN_POINT('Ctrl Pts',(37.7198552916762,-6.73548599752059,-11.4211223147714));
#63355=CARTESIAN_POINT('Ctrl Pts',(37.7326816424699,-6.73686719019395,-11.4309983805954));
#63356=CARTESIAN_POINT('Ctrl Pts',(37.7328493229138,-6.73688524341524,-11.4311274563635));
#63357=CARTESIAN_POINT('Ctrl Pts',(37.7331836619575,-6.7369212333024,-11.4313847510581));
#63358=CARTESIAN_POINT('Ctrl Pts',(37.7333503203456,-6.73693916998665,-11.431512970264));
#63359=CARTESIAN_POINT('Ctrl Pts',(37.7336830354551,-6.73697497213335,-11.4317688763368));
#63360=CARTESIAN_POINT('Ctrl Pts',(37.7338490920594,-6.73699283760785,-11.4318965633782));
#63361=CARTESIAN_POINT('Ctrl Pts',(37.7341810275632,-6.73702854301002,-11.4321517318273));
#63362=CARTESIAN_POINT('Ctrl Pts',(37.7343469064506,-6.73704638294455,-11.4322792133131));
#63363=CARTESIAN_POINT('Ctrl Pts',(37.7346789187009,-6.73708208375974,-11.432534302964));
#63364=CARTESIAN_POINT('Ctrl Pts',(37.7348450520678,-6.73709994463227,-11.4326619110403));
#63365=CARTESIAN_POINT('Ctrl Pts',(37.7351780183152,-6.73713573513146,-11.4329175953405));
#63366=CARTESIAN_POINT('Ctrl Pts',(37.7353448513137,-6.73715366474497,-11.4330456713778));
#63367=CARTESIAN_POINT('Ctrl Pts',(37.7356796799401,-6.73718964240742,-11.4333026462008));
#63368=CARTESIAN_POINT('Ctrl Pts',(37.7358476757828,-6.73720769043537,-11.4334315446793));
#63369=CARTESIAN_POINT('Ctrl Pts',(37.7361853171221,-6.73724395710308,-11.4336905365446));
#63370=CARTESIAN_POINT('Ctrl Pts',(37.7363549629734,-6.73726217571738,-11.4338206295227));
#63371=CARTESIAN_POINT('Ctrl Pts',(37.7366964219543,-6.73729883894172,-11.4340824051724));
#63372=CARTESIAN_POINT('Ctrl Pts',(37.736868235519,-6.73731728351362,-11.4342140872691));
#63373=CARTESIAN_POINT('Ctrl Pts',(37.7372145857926,-6.7373544580567,-11.4344794643356));
#63374=CARTESIAN_POINT('Ctrl Pts',(37.7373891230734,-6.73737318798078,-11.4346131585831));
#63375=CARTESIAN_POINT('Ctrl Pts',(37.7377415239058,-6.7374109976085,-11.43488301832));
#63376=CARTESIAN_POINT('Ctrl Pts',(37.7379193881638,-6.73743007725286,-11.4350191829061));
#63377=CARTESIAN_POINT('Ctrl Pts',(37.7382791040823,-6.73746865681699,-11.4352944849595));
#63378=CARTESIAN_POINT('Ctrl Pts',(37.7384609565821,-6.73748815666127,-11.4354336213003));
#63379=CARTESIAN_POINT('Ctrl Pts',(37.7388293809965,-6.73752765459989,-11.4357154214385));
#63380=CARTESIAN_POINT('Ctrl Pts',(37.7390159539487,-6.73754765260462,-11.4358580838842));
#63381=CARTESIAN_POINT('Ctrl Pts',(37.739394637933,-6.73758823398598,-11.4361475555698));
#63382=CARTESIAN_POINT('Ctrl Pts',(37.7395867502073,-6.73760881725327,-11.4362943631711));
#63383=CARTESIAN_POINT('Ctrl Pts',(37.7399774375662,-6.7376506674804,-11.4365928238029));
#63384=CARTESIAN_POINT('Ctrl Pts',(37.7401760141838,-6.73767193431238,-11.4367444748885));
#63385=CARTESIAN_POINT('Ctrl Pts',(37.7405806853476,-6.7377152637571,-11.4370534186145));
#63386=CARTESIAN_POINT('Ctrl Pts',(37.7407867817177,-6.73773732621305,-11.4372107088933));
#63387=CARTESIAN_POINT('Ctrl Pts',(37.7412077086163,-6.73778237600391,-11.4375318475774));
#63388=CARTESIAN_POINT('Ctrl Pts',(37.7414225413037,-6.73780536314421,-11.4376956930943));
#63389=CARTESIAN_POINT('Ctrl Pts',(37.7418623574362,-6.73785241255197,-11.438031008572));
#63390=CARTESIAN_POINT('Ctrl Pts',(37.7420873435587,-6.73787647458877,-11.4382024750684));
#63391=CARTESIAN_POINT('Ctrl Pts',(37.7425491346872,-6.73792585057906,-11.4385542867136));
#63392=CARTESIAN_POINT('Ctrl Pts',(37.7427859429672,-6.73795116425038,-11.4387346276292));
#63393=CARTESIAN_POINT('Ctrl Pts',(37.7432733654522,-6.73800325393794,-11.4391056804099));
#63394=CARTESIAN_POINT('Ctrl Pts',(37.7435239836945,-6.73803002960599,-11.4392963870586));
#63395=CARTESIAN_POINT('Ctrl Pts',(37.7524331798043,-6.73898161442979,-11.4460730311482));
#63396=CARTESIAN_POINT('Ctrl Pts',(37.761136422089,-6.73990242395748,-11.4526002992707));
#63397=CARTESIAN_POINT('Ctrl Pts',(37.7803585487991,-6.74191682629841,-11.4668137890099));
#63398=CARTESIAN_POINT('Ctrl Pts',(37.7908959667028,-6.74300869093637,-11.4744739005115));
#63399=CARTESIAN_POINT('Ctrl Pts',(37.8222640585244,-6.74622421569818,-11.4968895038783));
#63400=CARTESIAN_POINT('Ctrl Pts',(37.8432688417769,-6.74833256294983,-11.5114000762294));
#63401=CARTESIAN_POINT('Ctrl Pts',(37.9641873841679,-6.76024257099755,-11.592120135349));
#63402=CARTESIAN_POINT('Ctrl Pts',(38.0687224461405,-6.76967388898407,-11.6511321611206));
#63403=CARTESIAN_POINT('Ctrl Pts',(38.2873834282866,-6.7886158749594,-11.7538548467886));
#63404=CARTESIAN_POINT('Ctrl Pts',(38.401292479853,-6.79810090833219,-11.7971634779365));
#63405=CARTESIAN_POINT('Ctrl Pts',(38.5849579538793,-6.81337050174021,-11.8514680719438));
#63406=CARTESIAN_POINT('Ctrl Pts',(38.6527548206729,-6.81899987655743,-11.8683419358709));
#63407=CARTESIAN_POINT('Ctrl Pts',(38.7477409148245,-6.82694091070454,-11.8876360336061));
#63408=CARTESIAN_POINT('Ctrl Pts',(38.7743858473484,-6.82917411420624,-11.8925809975287));
#63409=CARTESIAN_POINT('Ctrl Pts',(38.8204492586569,-6.83304795322695,-11.9003271057356));
#63410=CARTESIAN_POINT('Ctrl Pts',(38.8398293911233,-6.83468174645656,-11.9033428493689));
#63411=CARTESIAN_POINT('Ctrl Pts',(38.8796740548795,-6.83805014577164,-11.9090449205769));
#63412=CARTESIAN_POINT('Ctrl Pts',(38.9001405480022,-6.83978540982395,-11.9117055006084));
#63413=CARTESIAN_POINT('Ctrl Pts',(38.9528809944916,-6.84427156090478,-11.9178725336195));
#63414=CARTESIAN_POINT('Ctrl Pts',(38.9851951655634,-6.84703421948019,-11.9209894463542));
#63415=CARTESIAN_POINT('Ctrl Pts',(39.154662731107,-6.8616040651487,-11.9338800625799));
#63416=CARTESIAN_POINT('Ctrl Pts',(39.2923794695661,-6.87374447884458,-11.9325321528038));
#63417=CARTESIAN_POINT('Ctrl Pts',(39.5509855063054,-6.89701388041658,-11.9077776026887));
#63418=CARTESIAN_POINT('Ctrl Pts',(39.6717031521427,-6.90806971246242,-11.8868461744628));
#63419=CARTESIAN_POINT('Ctrl Pts',(39.8434288012692,-6.92378020262187,-11.8433733816551));
#63420=CARTESIAN_POINT('Ctrl Pts',(39.8960815563142,-6.9285927737816,-11.8281125587806));
#63421=CARTESIAN_POINT('Ctrl Pts',(39.9645728675133,-6.93481162982387,-11.8056970587235));
#63422=CARTESIAN_POINT('Ctrl Pts',(39.9809162230095,-6.93629238467935,-11.8001528848118));
#63423=CARTESIAN_POINT('Ctrl Pts',(40.0078608141697,-6.93872683237865,-11.7906878746723));
#63424=CARTESIAN_POINT('Ctrl Pts',(40.0184963349342,-6.93968597757649,-11.7868674612639));
#63425=CARTESIAN_POINT('Ctrl Pts',(40.0401935171523,-6.94163854392647,-11.7789004704902));
#63426=CARTESIAN_POINT('Ctrl Pts',(40.0512522462144,-6.94263156257877,-11.7747471211273));
#63427=CARTESIAN_POINT('Ctrl Pts',(40.0806500064579,-6.94526669973878,-11.7634583345894));
#63428=CARTESIAN_POINT('Ctrl Pts',(40.0989333776727,-6.9469007351729,-11.7561788383743));
#63429=CARTESIAN_POINT('Ctrl Pts',(40.1919966226582,-6.95520366280167,-11.7177961031288));
#63430=CARTESIAN_POINT('Ctrl Pts',(40.2652699604614,-6.96169375148389,-11.6831509350186));
#63431=CARTESIAN_POINT('Ctrl Pts',(40.4746208673889,-6.98050300226922,-11.5708979512558));
#63432=CARTESIAN_POINT('Ctrl Pts',(40.6050269756479,-6.9925895708988,-11.4836366796581));
#63433=CARTESIAN_POINT('Ctrl Pts',(40.7885758196115,-7.01143830824701,-11.3329896599929));
#63434=CARTESIAN_POINT('Ctrl Pts',(40.8484831470591,-7.01793395749599,-11.2785394417222));
#63435=CARTESIAN_POINT('Ctrl Pts',(40.9255759232657,-7.02687861515469,-11.2010217535354));
#63436=CARTESIAN_POINT('Ctrl Pts',(40.9452635025684,-7.02921879139036,-11.1805109040702));
#63437=CARTESIAN_POINT('Ctrl Pts',(40.9780695963466,-7.03321897771903,-11.1450973258889));
#63438=CARTESIAN_POINT('Ctrl Pts',(40.9913759229167,-7.03487091201093,-11.1303719469763));
#63439=CARTESIAN_POINT('Ctrl Pts',(41.016334868724,-7.03802746795102,-11.1020545487435));
#63440=CARTESIAN_POINT('Ctrl Pts',(41.0280209943483,-7.03953056551109,-11.0884937199208));
#63441=CARTESIAN_POINT('Ctrl Pts',(41.0550597121541,-7.04306900646214,-11.0563998633379));
#63442=CARTESIAN_POINT('Ctrl Pts',(41.0702873893966,-7.04510917880011,-11.0377647099678));
#63443=CARTESIAN_POINT('Ctrl Pts',(41.1239757211677,-7.0524782179523,-10.9700127558453));
#63444=CARTESIAN_POINT('Ctrl Pts',(41.1607984526013,-7.05786865066967,-10.9196370040375));
#63445=CARTESIAN_POINT('Ctrl Pts',(41.3161643070524,-7.08221193381776,-10.6887539425036));
#63446=CARTESIAN_POINT('Ctrl Pts',(41.4120335234907,-7.1018957366992,-10.4942048998635));
#63447=CARTESIAN_POINT('Ctrl Pts',(41.4966273510425,-7.12545217856426,-10.2418572465852));
#63448=CARTESIAN_POINT('Ctrl Pts',(41.5111126641656,-7.12985987359822,-10.1936858318763));
#63449=CARTESIAN_POINT('Ctrl Pts',(41.528401992268,-7.13564334628572,-10.1288860881664));
#63450=CARTESIAN_POINT('Ctrl Pts',(41.5325562912574,-7.13708166834152,-10.1126354672255));
#63451=CARTESIAN_POINT('Ctrl Pts',(41.5392022018627,-7.13946574671488,-10.0854565825735));
#63452=CARTESIAN_POINT('Ctrl Pts',(41.5417879716383,-7.1404165114773,-10.0745522188296));
#63453=CARTESIAN_POINT('Ctrl Pts',(41.5469762837167,-7.14237306633793,-10.051970937339));
#63454=CARTESIAN_POINT('Ctrl Pts',(41.5495680853971,-7.14337826812535,-10.0402920302354));
#63455=CARTESIAN_POINT('Ctrl Pts',(41.5563388034762,-7.14608318061396,-10.0086688871477));
#63456=CARTESIAN_POINT('Ctrl Pts',(41.5603517338086,-7.14777404456037,-9.98868947203034));
#63457=CARTESIAN_POINT('Ctrl Pts',(41.5834156080898,-7.15807825410333,-9.86579020240314));
#63458=CARTESIAN_POINT('Ctrl Pts',(41.5959888290629,-7.16638815582971,-9.76175328351839));
#63459=CARTESIAN_POINT('Ctrl Pts',(41.609303289201,-7.1854464791118,-9.51988788413041));
#63460=CARTESIAN_POINT('Ctrl Pts',(41.6050711605563,-7.19611602353937,-9.38217148976502));
#63461=CARTESIAN_POINT('Ctrl Pts',(41.5802468024443,-7.21310905505812,-9.16992358403679));
#63462=CARTESIAN_POINT('Ctrl Pts',(41.5678117207838,-7.21923401000237,-9.09474469183967));
#63463=CARTESIAN_POINT('Ctrl Pts',(41.5459815571247,-7.2277507799812,-8.99302141375947));
#63464=CARTESIAN_POINT('Ctrl Pts',(41.5396564342281,-7.23004741377237,-8.96585930089216));
#63465=CARTESIAN_POINT('Ctrl Pts',(41.5280479998318,-7.23399592570049,-8.91966085858103));
#63466=CARTESIAN_POINT('Ctrl Pts',(41.5229996769323,-7.23564023579455,-8.90056792375326));
#63467=CARTESIAN_POINT('Ctrl Pts',(41.5122581110401,-7.23899905865904,-8.86187724229014));
#63468=CARTESIAN_POINT('Ctrl Pts',(41.5065494230994,-7.24071394413184,-8.84228551521467));
#63469=CARTESIAN_POINT('Ctrl Pts',(41.491449594579,-7.24508129875793,-8.79281664961974));
#63470=CARTESIAN_POINT('Ctrl Pts',(41.4817232373491,-7.24774434467291,-8.76304686987602));
#63471=CARTESIAN_POINT('Ctrl Pts',(41.4368783200271,-7.2594152058107,-8.63435625015533));
#63472=CARTESIAN_POINT('Ctrl Pts',(41.3958923154472,-7.26860837135119,-8.53761894578032));
#63473=CARTESIAN_POINT('Ctrl Pts',(41.2825107275651,-7.29104467985914,-8.31227283041029));
#63474=CARTESIAN_POINT('Ctrl Pts',(41.2043462575023,-7.30439011615891,-8.18703455269513));
#63475=CARTESIAN_POINT('Ctrl Pts',(41.0770538417761,-7.32311044022609,-8.01950967201676));
#63476=CARTESIAN_POINT('Ctrl Pts',(41.036923703605,-7.32866877645552,-7.9707975292015));
#63477=CARTESIAN_POINT('Ctrl Pts',(40.9829175125755,-7.33567673440827,-7.91026064983037));
#63478=CARTESIAN_POINT('Ctrl Pts',(40.9707633029699,-7.3372251856827,-7.89694121401002));
#63479=CARTESIAN_POINT('Ctrl Pts',(40.9506412288704,-7.33974066313203,-7.87538200183495));
#63480=CARTESIAN_POINT('Ctrl Pts',(40.9427624964945,-7.34071385987671,-7.86706057043653));
#63481=CARTESIAN_POINT('Ctrl Pts',(40.9277557464838,-7.34254499472489,-7.85143579324031));
#63482=CARTESIAN_POINT('Ctrl Pts',(40.9206402192662,-7.34340387044973,-7.84412096759225));
#63483=CARTESIAN_POINT('Ctrl Pts',(40.901282556124,-7.34571604528823,-7.82447285515044));
#63484=CARTESIAN_POINT('Ctrl Pts',(40.8889526347475,-7.34716280630934,-7.81222623854819));
#63485=CARTESIAN_POINT('Ctrl Pts',(40.839475904814,-7.35287180796252,-7.76413769347751));
#63486=CARTESIAN_POINT('Ctrl Pts',(40.8013090479579,-7.35706377639324,-7.72935868942916));
#63487=CARTESIAN_POINT('Ctrl Pts',(40.6607940735945,-7.37189143919899,-7.60936359430232));
#63488=CARTESIAN_POINT('Ctrl Pts',(40.5525263257329,-7.38223228760084,-7.53144522605973));
#63489=CARTESIAN_POINT('Ctrl Pts',(40.3636713449649,-7.39951503978045,-7.41803260097788));
#63490=CARTESIAN_POINT('Ctrl Pts',(40.2866090963879,-7.40637994508828,-7.37727530010874));
#63491=CARTESIAN_POINT('Ctrl Pts',(40.1544738549429,-7.41804344883372,-7.31632528217816));
#63492=CARTESIAN_POINT('Ctrl Pts',(40.1005680473364,-7.42277280644113,-7.29380290118905));
#63493=CARTESIAN_POINT('Ctrl Pts',(40.0220655853351,-7.42965597334912,-7.26431219118926));
#63494=CARTESIAN_POINT('Ctrl Pts',(39.9980914436809,-7.43175739982458,-7.25573775377028));
#63495=CARTESIAN_POINT('Ctrl Pts',(39.9556489513511,-7.43547934972116,-7.24131378795487));
#63496=CARTESIAN_POINT('Ctrl Pts',(39.9372372553629,-7.43709449387007,-7.23530368043308));
#63497=CARTESIAN_POINT('Ctrl Pts',(39.8984453192548,-7.44049985045436,-7.22315725364914));
#63498=CARTESIAN_POINT('Ctrl Pts',(39.8780523027481,-7.44229142140527,-7.21706782915396));
#63499=CARTESIAN_POINT('Ctrl Pts',(39.8233393019105,-7.44710339623546,-7.20151806061534));
#63500=CARTESIAN_POINT('Ctrl Pts',(39.788886984732,-7.45013907017388,-7.19254806340412));
#63501=CARTESIAN_POINT('Ctrl Pts',(39.5724500673931,-7.46925690701238,-7.14129733218012));
#63502=CARTESIAN_POINT('Ctrl Pts',(39.386289774908,-7.48598117123899,-7.11958440573875));
#63503=CARTESIAN_POINT('Ctrl Pts',(39.084101005368,-7.5131316433615,-7.1196420736939));
#63504=CARTESIAN_POINT('Ctrl Pts',(38.9687974283207,-7.52347149521631,-7.12797446899214));
#63505=CARTESIAN_POINT('Ctrl Pts',(38.8342146259304,-7.53525485945145,-7.14750652346068));
#63506=CARTESIAN_POINT('Ctrl Pts',(38.8139411176832,-7.53702193602859,-7.15071425548855));
#63507=CARTESIAN_POINT('Ctrl Pts',(38.7818884797256,-7.53980063131737,-7.15620715199266));
#63508=CARTESIAN_POINT('Ctrl Pts',(38.7700817420961,-7.54082092028483,-7.15832150238878));
#63509=CARTESIAN_POINT('Ctrl Pts',(38.7474207796818,-7.54277231434138,-7.16255480967862));
#63510=CARTESIAN_POINT('Ctrl Pts',(38.7365646370478,-7.54370405939397,-7.16466042679972));
#63511=CARTESIAN_POINT('Ctrl Pts',(38.7121176425693,-7.54579599692027,-7.16957724655369));
#63512=CARTESIAN_POINT('Ctrl Pts',(38.6985355659258,-7.54695385491767,-7.17243140553701));
#63513=CARTESIAN_POINT('Ctrl Pts',(38.6495097132471,-7.55112004207163,-7.18317766153988));
#63514=CARTESIAN_POINT('Ctrl Pts',(38.6142187403869,-7.55409399807666,-7.19175501664385));
#63515=CARTESIAN_POINT('Ctrl Pts',(38.3306292569215,-7.57789191888648,-7.26752144154939));
#63516=CARTESIAN_POINT('Ctrl Pts',(38.0943662873774,-7.59726436997668,-7.37334475882706));
#63517=CARTESIAN_POINT('Ctrl Pts',(37.8399552926992,-7.62181673862617,-7.54047206003717));
#63518=CARTESIAN_POINT('Ctrl Pts',(37.8013484148333,-7.62565114144592,-7.56748986856382));
#63519=CARTESIAN_POINT('Ctrl Pts',(37.7446781114511,-7.63146445660931,-7.60968138054314));
#63520=CARTESIAN_POINT('Ctrl Pts',(37.7260022544897,-7.63341165048591,-7.6240166284239));
#63521=CARTESIAN_POINT('Ctrl Pts',(37.693946787916,-7.6368110863648,-7.64937820288367));
#63522=CARTESIAN_POINT('Ctrl Pts',(37.6804701345545,-7.6382583443645,-7.66027954958062));
#63523=CARTESIAN_POINT('Ctrl Pts',(37.650317950409,-7.64153847116682,-7.68521374962079));
#63524=CARTESIAN_POINT('Ctrl Pts',(37.6337131969188,-7.64337457300378,-7.69932930534523));
#63525=CARTESIAN_POINT('Ctrl Pts',(37.5893616877527,-7.64836189819676,-7.73808255289733));
#63526=CARTESIAN_POINT('Ctrl Pts',(37.5619906890326,-7.65153001601184,-7.76313879533985));
#63527=CARTESIAN_POINT('Ctrl Pts',(37.4128868552171,-7.66931288530945,-7.90611119976877));
#63528=CARTESIAN_POINT('Ctrl Pts',(37.3033244738866,-7.684438800844,-8.03598223007141));
#63529=CARTESIAN_POINT('Ctrl Pts',(37.1360743121515,-7.71124531933222,-8.28295695108838));
#63530=CARTESIAN_POINT('Ctrl Pts',(37.072497836211,-7.72282786446461,-8.39530858016603));
#63531=CARTESIAN_POINT('Ctrl Pts',(37.0095099486189,-7.7357927206205,-8.53100064399404));
#63532=CARTESIAN_POINT('Ctrl Pts',(37.0010370610652,-7.73757515561057,-8.54988797231634));
#63533=CARTESIAN_POINT('Ctrl Pts',(36.9880262531494,-7.74037230706476,-8.57992336701947));
#63534=CARTESIAN_POINT('Ctrl Pts',(36.9833266177378,-7.7413958809209,-8.59099955306472));
#63535=CARTESIAN_POINT('Ctrl Pts',(36.9744746554689,-7.74334900692064,-8.61230522698373));
#63536=CARTESIAN_POINT('Ctrl Pts',(36.9703093571092,-7.74427924014572,-8.62252869679819));
#63537=CARTESIAN_POINT('Ctrl Pts',(36.9634507368028,-7.74583057432999,-8.63970013303504));
#63538=CARTESIAN_POINT('Ctrl Pts',(36.9607191031609,-7.74645386404971,-8.64663246328934));
#63539=CARTESIAN_POINT('Ctrl Pts',(36.9580196848653,-7.74707540691374,-8.65357747851663));
#63540=CARTESIAN_POINT('Origin',(39.2,8.05522481984854,-9.525));
#63541=CARTESIAN_POINT('',(36.958019684865,-9.28019056162069,-8.65357747851727));
#63542=CARTESIAN_POINT('',(36.9580196445751,-9.01353011641035,-8.65357758217454));
#63543=CARTESIAN_POINT('',(36.958019684865,8.05522481984854,-8.65357747851728));
#63544=CARTESIAN_POINT('',(36.7946209480143,-8.08522481984856,-9.52713557209757));
#63545=CARTESIAN_POINT('Ctrl Pts',(36.7946209480143,-8.08522481984856,-9.52713557209757));
#63546=CARTESIAN_POINT('Ctrl Pts',(36.7947125349209,-8.09388971051084,-9.63029351600966));
#63547=CARTESIAN_POINT('Ctrl Pts',(36.8014440163763,-8.10255460117313,-9.73316083263825));
#63548=CARTESIAN_POINT('Ctrl Pts',(36.8146812005732,-8.11121949183542,-9.83501156349611));
#63549=CARTESIAN_POINT('Ctrl Pts',(36.8273339973927,-8.11950185003041,-9.93236584853728));
#63550=CARTESIAN_POINT('Ctrl Pts',(36.8459303117105,-8.12778420822541,-10.0287917844142));
#63551=CARTESIAN_POINT('Ctrl Pts',(36.8703130343641,-8.1360665664204,-10.1236748587891));
#63552=CARTESIAN_POINT('Ctrl Pts',(36.890192917571,-8.14281939365521,-10.2010355565127));
#63553=CARTESIAN_POINT('Ctrl Pts',(36.9139671233725,-8.14957222089002,-10.2775483060069));
#63554=CARTESIAN_POINT('Ctrl Pts',(36.9415464626432,-8.15632504812483,-10.3527925851326));
#63555=CARTESIAN_POINT('Ctrl Pts',(36.969086513572,-8.16306825557206,-10.4279296744907));
#63556=CARTESIAN_POINT('Ctrl Pts',(37.0004207730383,-8.16981146301929,-10.5018014480561));
#63557=CARTESIAN_POINT('Ctrl Pts',(37.0354096749355,-8.17655467046653,-10.5740003188927));
#63558=CARTESIAN_POINT('Ctrl Pts',(37.0703585153005,-8.1832901570878,-10.6461165235915));
#63559=CARTESIAN_POINT('Ctrl Pts',(37.1089534794919,-8.19002564370908,-10.7165632147592));
#63560=CARTESIAN_POINT('Ctrl Pts',(37.1510066430008,-8.19676113033035,-10.7849520496325));
#63561=CARTESIAN_POINT('Ctrl Pts',(37.1930334705739,-8.20349239883036,-10.8532980557668));
#63562=CARTESIAN_POINT('Ctrl Pts',(37.2385139547638,-8.21022366733036,-10.9195883676319));
#63563=CARTESIAN_POINT('Ctrl Pts',(37.2872144678815,-8.21695493583037,-10.983459616348));
#63564=CARTESIAN_POINT('Ctrl Pts',(37.3358994818713,-8.22368406207796,-11.0473105377906));
#63565=CARTESIAN_POINT('Ctrl Pts',(37.3878022070609,-8.23041318832557,-11.1087435544642));
#63566=CARTESIAN_POINT('Ctrl Pts',(37.44264680587,-8.23714231457317,-11.1674258569205));
#63567=CARTESIAN_POINT('Ctrl Pts',(37.4974908418339,-8.2438713717628,-11.2261075571471));
#63568=CARTESIAN_POINT('Ctrl Pts',(37.555276371965,-8.25060042895244,-11.2820382595347));
#63569=CARTESIAN_POINT('Ctrl Pts',(37.6156895375635,-8.25732948614207,-11.3349208002048));
#63570=CARTESIAN_POINT('Ctrl Pts',(37.676162183044,-8.26406516843609,-11.3878554064679));
#63571=CARTESIAN_POINT('Ctrl Pts',(37.7392672801181,-8.27080085073012,-11.4377355482707));
#63572=CARTESIAN_POINT('Ctrl Pts',(37.8046570358675,-8.27753653302414,-11.484303691837));
#63573=CARTESIAN_POINT('Ctrl Pts',(37.8700780195631,-8.28427543205327,-11.530894074781));
#63574=CARTESIAN_POINT('Ctrl Pts',(37.9377854422335,-8.29101433108241,-11.5741690568134));
#63575=CARTESIAN_POINT('Ctrl Pts',(38.007403729675,-8.29775323011155,-11.6139152879921));
#63576=CARTESIAN_POINT('Ctrl Pts',(38.0771462831552,-8.30450415782335,-11.6537324647064));
#63577=CARTESIAN_POINT('Ctrl Pts',(38.1488060997928,-8.31125508553515,-11.6900080934659));
#63578=CARTESIAN_POINT('Ctrl Pts',(38.2219844649816,-8.31800601324695,-11.722575609089));
#63579=CARTESIAN_POINT('Ctrl Pts',(38.2894306676579,-8.3242281314581,-11.7525920661895));
#63580=CARTESIAN_POINT('Ctrl Pts',(38.3581663381352,-8.33045024966925,-11.7794590313155));
#63581=CARTESIAN_POINT('Ctrl Pts',(38.427868318026,-8.3366723678804,-11.8030837583575));
#63582=CARTESIAN_POINT('Ctrl Pts',(38.5035154551363,-8.34342519513398,-11.8287235316973));
#63583=CARTESIAN_POINT('Ctrl Pts',(38.5805812464378,-8.35017802238755,-11.8506387668023));
#63584=CARTESIAN_POINT('Ctrl Pts',(38.6586648020085,-8.35693084964113,-11.8686742836443));
#63585=CARTESIAN_POINT('Ctrl Pts',(38.7366371230947,-8.36367405710662,-11.8866841078624));
#63586=CARTESIAN_POINT('Ctrl Pts',(38.8156238782593,-8.3704172645721,-11.9008250865046));
#63587=CARTESIAN_POINT('Ctrl Pts',(38.8952074722694,-8.37716047203758,-11.9109912949212));
#63588=CARTESIAN_POINT('Ctrl Pts',(38.9746999447843,-8.38389595867624,-11.9211458632488));
#63589=CARTESIAN_POINT('Ctrl Pts',(39.0547874377658,-8.39063144531491,-11.9273346472732));
#63590=CARTESIAN_POINT('Ctrl Pts',(39.1350420370788,-8.39736693195357,-11.9295027360045));
#63591=CARTESIAN_POINT('Ctrl Pts',(39.2152463766714,-8.40409820047043,-11.9316694669628));
#63592=CARTESIAN_POINT('Ctrl Pts',(39.2956171499091,-8.41082946898729,-11.9298204884061));
#63593=CARTESIAN_POINT('Ctrl Pts',(39.3757223731024,-8.41756073750415,-11.9239528115391));
#63594=CARTESIAN_POINT('Ctrl Pts',(39.45580210249,-8.42428986376805,-11.9180870020835));
#63595=CARTESIAN_POINT('Ctrl Pts',(39.535615984925,-8.43101899003195,-11.908205068333));
#63596=CARTESIAN_POINT('Ctrl Pts',(39.6147345538958,-8.43774811629586,-11.8943560716374));
#63597=CARTESIAN_POINT('Ctrl Pts',(39.6938523109022,-8.44447717350124,-11.8805072170688));
#63598=CARTESIAN_POINT('Ctrl Pts',(39.7722743095289,-8.45120623070661,-11.862691462269));
#63599=CARTESIAN_POINT('Ctrl Pts',(39.849580149142,-8.45793528791199,-11.8410091913118));
#63600=CARTESIAN_POINT('Ctrl Pts',(39.9269621003357,-8.46467097022075,-11.8193055730421));
#63601=CARTESIAN_POINT('Ctrl Pts',(40.0032252473015,-8.47140665252953,-11.793727960483));
#63602=CARTESIAN_POINT('Ctrl Pts',(40.0779638258342,-8.47814233483829,-11.7644268161578));
#63603=CARTESIAN_POINT('Ctrl Pts',(40.1527380969901,-8.48488123388166,-11.7351116785947));
#63604=CARTESIAN_POINT('Ctrl Pts',(40.2259859235215,-8.49162013292502,-11.7020696585099));
#63605=CARTESIAN_POINT('Ctrl Pts',(40.2973233541722,-8.49835903196838,-11.6654986336806));
#63606=CARTESIAN_POINT('Ctrl Pts',(40.3687881194565,-8.50510995969337,-11.6288623309458));
#63607=CARTESIAN_POINT('Ctrl Pts',(40.438335270284,-8.51186088741837,-11.5886846704396));
#63608=CARTESIAN_POINT('Ctrl Pts',(40.5056073831098,-8.51861181514336,-11.5452084807191));
#63609=CARTESIAN_POINT('Ctrl Pts',(40.5676099767651,-8.52483393320903,-11.5051378420593));
#63610=CARTESIAN_POINT('Ctrl Pts',(40.6276800916756,-8.5310560512747,-11.4622658551984));
#63611=CARTESIAN_POINT('Ctrl Pts',(40.6855634194983,-8.53727816934038,-11.4168124301972));
#63612=CARTESIAN_POINT('Ctrl Pts',(40.7483838482196,-8.54403099678038,-11.3674821005007));
#63613=CARTESIAN_POINT('Ctrl Pts',(40.808860880547,-8.55078382422039,-11.3149279128816));
#63614=CARTESIAN_POINT('Ctrl Pts',(40.8666454375787,-8.5575366516604,-11.2594007408318));
#63615=CARTESIAN_POINT('Ctrl Pts',(40.9243476772194,-8.56427985931329,-11.2039526703997));
#63616=CARTESIAN_POINT('Ctrl Pts',(40.9793647258058,-8.57102306696619,-11.1455403473925));
#63617=CARTESIAN_POINT('Ctrl Pts',(41.0313796185417,-8.57776627461908,-11.08445555794));
#63618=CARTESIAN_POINT('Ctrl Pts',(41.0833349553559,-8.58450176144576,-11.0234407092439));
#63619=CARTESIAN_POINT('Ctrl Pts',(41.1322946670043,-8.59123724827243,-10.959759828654));
#63620=CARTESIAN_POINT('Ctrl Pts',(41.1779788660801,-8.59797273509911,-10.8937412281876));
#63621=CARTESIAN_POINT('Ctrl Pts',(41.2236344552709,-8.60470400380426,-10.8277639720941));
#63622=CARTESIAN_POINT('Ctrl Pts',(41.2660183391843,-8.61143527250941,-10.7594522847394));
#63623=CARTESIAN_POINT('Ctrl Pts',(41.3048918846036,-8.61816654121456,-10.6891662675623));
#63624=CARTESIAN_POINT('Ctrl Pts',(41.3437530583631,-8.62489566766676,-10.6189026191887));
#63625=CARTESIAN_POINT('Ctrl Pts',(41.379105886766,-8.63162479411896,-10.5466662966233));
#63626=CARTESIAN_POINT('Ctrl Pts',(41.410756698362,-8.63835392057116,-10.4728437450591));
#63627=CARTESIAN_POINT('Ctrl Pts',(41.4424071851363,-8.64508297796458,-10.399021951111));
#63628=CARTESIAN_POINT('Ctrl Pts',(41.4703555481585,-8.651812035358,-10.3236143896706));
#63629=CARTESIAN_POINT('Ctrl Pts',(41.4944560482581,-8.65854109275142,-10.2470279683032));
#63630=CARTESIAN_POINT('Ctrl Pts',(41.5185802765345,-8.66527677524652,-10.170366143681));
#63631=CARTESIAN_POINT('Ctrl Pts',(41.5388489339166,-8.67201245774162,-10.0925235864974));
#63632=CARTESIAN_POINT('Ctrl Pts',(41.5551662165498,-8.67874814023672,-10.0139223218698));
#63633=CARTESIAN_POINT('Ctrl Pts',(41.5714912917648,-8.68548703946577,-9.93528351993889));
#63634=CARTESIAN_POINT('Ctrl Pts',(41.5838611608091,-8.69222593869483,-9.85588575006578));
#63635=CARTESIAN_POINT('Ctrl Pts',(41.5922316478546,-8.69896483792388,-9.77615868968205));
#63636=CARTESIAN_POINT('Ctrl Pts',(41.6006170759006,-8.7057157658313,-9.69628931953318));
#63637=CARTESIAN_POINT('Ctrl Pts',(41.6049888319449,-8.71246669373873,-9.61608995117826));
#63638=CARTESIAN_POINT('Ctrl Pts',(41.6053548816596,-8.71921762164615,-9.53599261918044));
#63639=CARTESIAN_POINT('Ctrl Pts',(41.6056922580852,-8.72543973803089,-9.46216944573941));
#63640=CARTESIAN_POINT('Ctrl Pts',(41.6026275097846,-8.73166185441563,-9.38843322435266));
#63641=CARTESIAN_POINT('Ctrl Pts',(41.5962057755786,-8.73788397080037,-9.3151171148383));
#63642=CARTESIAN_POINT('Ctrl Pts',(41.589236304541,-8.7446367977696,-9.23554756470546));
#63643=CARTESIAN_POINT('Ctrl Pts',(41.5782862902815,-8.75138962473884,-9.15617810952552));
#63644=CARTESIAN_POINT('Ctrl Pts',(41.5633749964623,-8.75814245170807,-9.07743819365742));
#63645=CARTESIAN_POINT('Ctrl Pts',(41.5484849446318,-8.76488565889009,-8.99881044729108));
#63646=CARTESIAN_POINT('Ctrl Pts',(41.5296449068395,-8.7716288660721,-8.92081091354556));
#63647=CARTESIAN_POINT('Ctrl Pts',(41.5069259604112,-8.77837207325411,-8.84386450864681));
#63648=CARTESIAN_POINT('Ctrl Pts',(41.4842330266779,-8.78510755961192,-8.7670062056926));
#63649=CARTESIAN_POINT('Ctrl Pts',(41.4576701422759,-8.79184304596973,-8.69119908015933));
#63650=CARTESIAN_POINT('Ctrl Pts',(41.4273592378361,-8.79857853232755,-8.61685696609709));
#63651=CARTESIAN_POINT('Ctrl Pts',(41.397067315698,-8.80530980056528,-8.54256140902384));
#63652=CARTESIAN_POINT('Ctrl Pts',(41.3630322084855,-8.812041068803,-8.46972947288336));
#63653=CARTESIAN_POINT('Ctrl Pts',(41.3254250170237,-8.81877233704073,-8.39875782293064));
#63654=CARTESIAN_POINT('Ctrl Pts',(41.2878297941888,-8.8255014630276,-8.32780875996649));
#63655=CARTESIAN_POINT('Ctrl Pts',(41.2466649629836,-8.83223058901446,-8.25871921917403));
#63656=CARTESIAN_POINT('Ctrl Pts',(41.2021482609573,-8.83895971500133,-8.19186261565221));
#63657=CARTESIAN_POINT('Ctrl Pts',(41.1576320157731,-8.84568877193213,-8.12500669823043));
#63658=CARTESIAN_POINT('Ctrl Pts',(41.109764227764,-8.85241782886293,-8.06038405990319));
#63659=CARTESIAN_POINT('Ctrl Pts',(41.0588059699817,-8.85914688579374,-7.99833916328465));
#63660=CARTESIAN_POINT('Ctrl Pts',(41.0077975411245,-8.86588256783368,-7.93623318021433));
#63661=CARTESIAN_POINT('Ctrl Pts',(40.9536928610552,-8.87261824987363,-7.87671036975368));
#63662=CARTESIAN_POINT('Ctrl Pts',(40.8967929575717,-8.87935393191357,-7.82008164314675));
#63663=CARTESIAN_POINT('Ctrl Pts',(40.83986588059,-8.88609283069084,-7.76342587254676));
#63664=CARTESIAN_POINT('Ctrl Pts',(40.7801412677275,-8.8928317294681,-7.70966725177175));
#63665=CARTESIAN_POINT('Ctrl Pts',(40.7179547755422,-8.89957062824536,-7.65907764260981));
#63666=CARTESIAN_POINT('Ctrl Pts',(40.6556572827293,-8.90632155571193,-7.60839773283484));
#63667=CARTESIAN_POINT('Ctrl Pts',(40.5908895067894,-8.9130724831785,-7.5608984140266));
#63668=CARTESIAN_POINT('Ctrl Pts',(40.5240175796269,-8.91982341064507,-7.51680917409751));
#63669=CARTESIAN_POINT('Ctrl Pts',(40.4623837976759,-8.9260455311835,-7.47617348860916));
#63670=CARTESIAN_POINT('Ctrl Pts',(40.3989631596466,-8.93226765172192,-7.43843421289083));
#63671=CARTESIAN_POINT('Ctrl Pts',(40.3340593217838,-8.93848977226034,-7.40373566025466));
#63672=CARTESIAN_POINT('Ctrl Pts',(40.2636196054445,-8.94524259952276,-7.36607754502513));
#63673=CARTESIAN_POINT('Ctrl Pts',(40.191171604636,-8.95199542678518,-7.33186203898538));
#63674=CARTESIAN_POINT('Ctrl Pts',(40.1170854580263,-8.9587482540476,-7.30130775351517));
#63675=CARTESIAN_POINT('Ctrl Pts',(40.0431048513928,-8.96549146151925,-7.27079699438167));
#63676=CARTESIAN_POINT('Ctrl Pts',(39.9674911613073,-8.97223466899091,-7.24393727356921));
#63677=CARTESIAN_POINT('Ctrl Pts',(39.8906390569906,-8.97897787646257,-7.22090133949106));
#63678=CARTESIAN_POINT('Ctrl Pts',(39.8138749467179,-8.98571336310341,-7.19789178107321));
#63679=CARTESIAN_POINT('Ctrl Pts',(39.7358756847227,-8.99244884974427,-7.1786974414596));
#63680=CARTESIAN_POINT('Ctrl Pts',(39.6570544575941,-8.99918433638512,-7.16344242771993));
#63681=CARTESIAN_POINT('Ctrl Pts',(39.5782825925599,-9.00591560490174,-7.14819696749085));
#63682=CARTESIAN_POINT('Ctrl Pts',(39.4986902408647,-9.01264687341836,-7.13688602432732));
#63683=CARTESIAN_POINT('Ctrl Pts',(39.4187030896245,-9.01937814193498,-7.12958314630028));
#63684=CARTESIAN_POINT('Ctrl Pts',(39.3387413946417,-9.02610726819624,-7.1222825924458));
#63685=CARTESIAN_POINT('Ctrl Pts',(39.2583856137036,-9.03283639445751,-7.11898761284158));
#63686=CARTESIAN_POINT('Ctrl Pts',(39.1780674571923,-9.03956552071877,-7.11971999385394));
#63687=CARTESIAN_POINT('Ctrl Pts',(39.0977501249847,-9.04629457791913,-7.1204523673499));
#63688=CARTESIAN_POINT('Ctrl Pts',(39.0174708827296,-9.05302363511949,-7.12521201364624));
#63689=CARTESIAN_POINT('Ctrl Pts',(38.9376608845403,-9.05975269231985,-7.13396860478583));
#63690=CARTESIAN_POINT('Ctrl Pts',(38.8577723093407,-9.06648837461994,-7.14273381723563));
#63691=CARTESIAN_POINT('Ctrl Pts',(38.7783543656978,-9.07322405692002,-7.15550378442089));
#63692=CARTESIAN_POINT('Ctrl Pts',(38.6998319524494,-9.07995973922011,-7.17219638120615));
#63693=CARTESIAN_POINT('Ctrl Pts',(38.6212720395694,-9.08669863825278,-7.1888969498074));
#63694=CARTESIAN_POINT('Ctrl Pts',(38.5436089604323,-9.09343753728544,-7.2095237603379));
#63695=CARTESIAN_POINT('Ctrl Pts',(38.4672538433217,-9.10017643631811,-7.23394434500747));
#63696=CARTESIAN_POINT('Ctrl Pts',(38.3907624352322,-9.10692736402916,-7.25840851949158));
#63697=CARTESIAN_POINT('Ctrl Pts',(38.3155840918235,-9.11367829174021,-7.28667983478684));
#63698=CARTESIAN_POINT('Ctrl Pts',(38.2421111166827,-9.12042921945127,-7.31857714124942));
#63699=CARTESIAN_POINT('Ctrl Pts',(38.1743933825736,-9.12665133754095,-7.34797588702892));
#63700=CARTESIAN_POINT('Ctrl Pts',(38.1081243179802,-9.13287345563064,-7.38045414295515));
#63701=CARTESIAN_POINT('Ctrl Pts',(38.043590752109,-9.13909557372032,-7.41583651752828));
#63702=CARTESIAN_POINT('Ctrl Pts',(37.9735684441467,-9.14584689860331,-7.45422825205204));
#63703=CARTESIAN_POINT('Ctrl Pts',(37.9053303526129,-9.15259822348629,-7.49618189473797));
#63704=CARTESIAN_POINT('Ctrl Pts',(37.8392616084537,-9.15934954836928,-7.54150712777384));
#63705=CARTESIAN_POINT('Ctrl Pts',(37.7732801318622,-9.16609195569664,-7.58677249251809));
#63706=CARTESIAN_POINT('Ctrl Pts',(37.7094626957699,-9.17283436302401,-7.63540034608263));
#63707=CARTESIAN_POINT('Ctrl Pts',(37.6481695692668,-9.17957677035136,-7.68715472396333));
#63708=CARTESIAN_POINT('Ctrl Pts',(37.5869385168687,-9.18631234936168,-7.73885668802749));
#63709=CARTESIAN_POINT('Ctrl Pts',(37.5282270519293,-9.19304792837199,-7.79367858954149));
#63710=CARTESIAN_POINT('Ctrl Pts',(37.4723649792722,-9.1997835073823,-7.85134227526805));
#63711=CARTESIAN_POINT('Ctrl Pts',(37.4165349163425,-9.20651522681425,-7.90897291891853));
#63712=CARTESIAN_POINT('Ctrl Pts',(37.3635513307144,-9.21324694624619,-7.96944178262451));
#63713=CARTESIAN_POINT('Ctrl Pts',(37.3137085688905,-9.21997866567814,-8.03243255384461));
#63714=CARTESIAN_POINT('Ctrl Pts',(37.2638848573161,-9.22670781220019,-8.09539924955469));
#63715=CARTESIAN_POINT('Ctrl Pts',(37.2171998715998,-9.23343695872224,-8.16088557055856));
#63716=CARTESIAN_POINT('Ctrl Pts',(37.1739078494426,-9.24016610524428,-8.22854192437635));
#63717=CARTESIAN_POINT('Ctrl Pts',(37.1305984247999,-9.24689795674221,-8.29622547463044));
#63718=CARTESIAN_POINT('Ctrl Pts',(37.0906849460329,-9.25362980824013,-8.36608041073893));
#63719=CARTESIAN_POINT('Ctrl Pts',(37.0543779583574,-9.26036165973806,-8.4377286452695));
#63720=CARTESIAN_POINT('Ctrl Pts',(37.0187301282128,-9.26697129369893,-8.50807609787391));
#63721=CARTESIAN_POINT('Ctrl Pts',(36.9865590682883,-9.27358092765981,-8.58015186205256));
#63722=CARTESIAN_POINT('Ctrl Pts',(36.958019684865,-9.28019056162069,-8.65357747851727));
#63723=CARTESIAN_POINT('Ctrl Pts',(36.960685369651,-8.0104155729454,-8.65458630036363));
#63724=CARTESIAN_POINT('Ctrl Pts',(36.8546210246965,-8.03535198857979,-8.93261473925435));
#63725=CARTESIAN_POINT('Ctrl Pts',(36.7977097135442,-8.06028840421417,-9.23031464669973));
#63726=CARTESIAN_POINT('Ctrl Pts',(36.7950831462415,-8.08522481984856,-9.52713516174327));
#63727=CARTESIAN_POINT('Ctrl Pts',(36.9580196848653,-7.74707540691374,-8.65357747851663));
#63728=CARTESIAN_POINT('Ctrl Pts',(36.9557192832498,-7.74760507592088,-8.65949591074869));
#63729=CARTESIAN_POINT('Ctrl Pts',(36.9534422769949,-7.74813347633361,-8.66542355503469));
#63730=CARTESIAN_POINT('Ctrl Pts',(36.9385689284089,-7.75161289183026,-8.70460560453435));
#63731=CARTESIAN_POINT('Ctrl Pts',(36.9266869243085,-7.75452656133757,-8.73812929403557));
#63732=CARTESIAN_POINT('Ctrl Pts',(36.863934925878,-7.77078488506504,-8.92848245261727));
#63733=CARTESIAN_POINT('Ctrl Pts',(36.828545827178,-7.78351852163012,-9.08996910296661));
#63734=CARTESIAN_POINT('Ctrl Pts',(36.8008855876117,-7.80279450956416,-9.33375563665433));
#63735=CARTESIAN_POINT('Ctrl Pts',(36.7958325908309,-7.80915024552102,-9.41408664139223));
#63736=CARTESIAN_POINT('Ctrl Pts',(36.7941109414962,-7.82005563610156,-9.54992027288729));
#63737=CARTESIAN_POINT('Ctrl Pts',(36.7953233986568,-7.82454801430526,-9.6053288116448));
#63738=CARTESIAN_POINT('Ctrl Pts',(36.7998563183302,-7.83114971608571,-9.6855844017261));
#63739=CARTESIAN_POINT('Ctrl Pts',(36.8016535078935,-7.8332126283415,-9.71050215909714));
#63740=CARTESIAN_POINT('Ctrl Pts',(36.8055272614556,-7.83689135166922,-9.75462162839259));
#63741=CARTESIAN_POINT('Ctrl Pts',(36.807447635962,-7.83850220249299,-9.77383514087833));
#63742=CARTESIAN_POINT('Ctrl Pts',(36.8119976958038,-7.84192430919047,-9.81441551111349));
#63743=CARTESIAN_POINT('Ctrl Pts',(36.814683320022,-7.84373716682399,-9.83577421790203));
#63744=CARTESIAN_POINT('Ctrl Pts',(36.8227343084892,-7.84867274740736,-9.89352977171098));
#63745=CARTESIAN_POINT('Ctrl Pts',(36.8286483929567,-7.85181215800447,-9.92984268068579));
#63746=CARTESIAN_POINT('Ctrl Pts',(36.8731323127851,-7.87268663518829,-10.1683600252124));
#63747=CARTESIAN_POINT('Ctrl Pts',(36.936685525334,-7.89121409677273,-10.3649976786444));
#63748=CARTESIAN_POINT('Ctrl Pts',(37.0651256510204,-7.91821393823356,-10.6373188243089));
#63749=CARTESIAN_POINT('Ctrl Pts',(37.110889416959,-7.92670498690201,-10.7210615521798));
#63750=CARTESIAN_POINT('Ctrl Pts',(37.1721034926394,-7.93669016016827,-10.8187878313208));
#63751=CARTESIAN_POINT('Ctrl Pts',(37.1829077053943,-7.93840744430387,-10.8355685605592));
#63752=CARTESIAN_POINT('Ctrl Pts',(37.2004708255962,-7.94112625358973,-10.862115169617));
#63753=CARTESIAN_POINT('Ctrl Pts',(37.2070950324872,-7.94213585262632,-10.8719683386859));
#63754=CARTESIAN_POINT('Ctrl Pts',(37.2200682466042,-7.94408216118704,-10.8909601018931));
#63755=CARTESIAN_POINT('Ctrl Pts',(37.2264081277018,-7.94501937406278,-10.9001043158043));
#63756=CARTESIAN_POINT('Ctrl Pts',(37.2425585166079,-7.94737296096718,-10.923056750464));
#63757=CARTESIAN_POINT('Ctrl Pts',(37.2524521310074,-7.94878393405045,-10.9368063560044));
#63758=CARTESIAN_POINT('Ctrl Pts',(37.2909028501468,-7.95415624462862,-10.9890695589739));
#63759=CARTESIAN_POINT('Ctrl Pts',(37.3204661500628,-7.95805740334165,-11.026833876662));
#63760=CARTESIAN_POINT('Ctrl Pts',(37.4485437095088,-7.97415993082891,-11.1807289991672));
#63761=CARTESIAN_POINT('Ctrl Pts',(37.5568471653784,-7.98593576459318,-11.2882625770026));
#63762=CARTESIAN_POINT('Ctrl Pts',(37.7653106740694,-8.00712926902897,-11.4592396438754));
#63763=CARTESIAN_POINT('Ctrl Pts',(37.8613299674977,-8.01643513006614,-11.5268923508703));
#63764=CARTESIAN_POINT('Ctrl Pts',(37.9887949419618,-8.02856506107532,-11.6034176554755));
#63765=CARTESIAN_POINT('Ctrl Pts',(38.0160108610134,-8.0311422410835,-11.619040873149));
#63766=CARTESIAN_POINT('Ctrl Pts',(38.0614275172243,-8.03542747858772,-11.6439437420481));
#63767=CARTESIAN_POINT('Ctrl Pts',(38.0794553534316,-8.03712454192942,-11.6535322459264));
#63768=CARTESIAN_POINT('Ctrl Pts',(38.1149484540488,-8.04045950887018,-11.6718341741303));
#63769=CARTESIAN_POINT('Ctrl Pts',(38.1324020566718,-8.04209658794781,-11.6805668424024));
#63770=CARTESIAN_POINT('Ctrl Pts',(38.1709689274312,-8.04570888633528,-11.699279952791));
#63771=CARTESIAN_POINT('Ctrl Pts',(38.1921249206493,-8.04768711216782,-11.7091671188801));
#63772=CARTESIAN_POINT('Ctrl Pts',(38.266274625906,-8.05461157351053,-11.7425140140712));
#63773=CARTESIAN_POINT('Ctrl Pts',(38.3199651512337,-8.05961020241652,-11.7643635105122));
#63774=CARTESIAN_POINT('Ctrl Pts',(38.5572104028629,-8.08165218037708,-11.8510615377907));
#63775=CARTESIAN_POINT('Ctrl Pts',(38.7474500407185,-8.09928992575252,-11.8954255131623));
#63776=CARTESIAN_POINT('Ctrl Pts',(38.9905235047393,-8.12111639917068,-11.9217609499181));
#63777=CARTESIAN_POINT('Ctrl Pts',(39.0402970256571,-8.12554394431615,-11.9255914087887));
#63778=CARTESIAN_POINT('Ctrl Pts',(39.1235724894052,-8.13285038807015,-11.9293982014905));
#63779=CARTESIAN_POINT('Ctrl Pts',(39.1570187879001,-8.13575765596819,-11.9302286426536));
#63780=CARTESIAN_POINT('Ctrl Pts',(39.2049352860259,-8.13987450483956,-11.9304184088523));
#63781=CARTESIAN_POINT('Ctrl Pts',(39.2193974376962,-8.14111075633384,-11.9303452664022));
#63782=CARTESIAN_POINT('Ctrl Pts',(39.2447272762823,-8.14326401399199,-11.9299886832563));
#63783=CARTESIAN_POINT('Ctrl Pts',(39.2555949139665,-8.14418393966456,-11.9297620091198));
#63784=CARTESIAN_POINT('Ctrl Pts',(39.2795586873442,-8.14620369170012,-11.9290996297714));
#63785=CARTESIAN_POINT('Ctrl Pts',(39.2926532760722,-8.14730171598736,-11.9286305892746));
#63786=CARTESIAN_POINT('Ctrl Pts',(39.3308393035071,-8.15048906115418,-11.9269502539552));
#63787=CARTESIAN_POINT('Ctrl Pts',(39.3559174288441,-8.15256380683637,-11.92545284318));
#63788=CARTESIAN_POINT('Ctrl Pts',(39.5022309677506,-8.16458522608844,-11.9144136441816));
#63789=CARTESIAN_POINT('Ctrl Pts',(39.6226431555327,-8.17414908542271,-11.8960804694966));
#63790=CARTESIAN_POINT('Ctrl Pts',(39.8603920576504,-8.1932779224102,-11.8411838736332));
#63791=CARTESIAN_POINT('Ctrl Pts',(39.9773354920761,-8.2028172729783,-11.8045991748579));
#63792=CARTESIAN_POINT('Ctrl Pts',(40.1542850305467,-8.21801628721203,-11.7340353721403));
#63793=CARTESIAN_POINT('Ctrl Pts',(40.2164787761007,-8.22351296900573,-11.7061158854337));
#63794=CARTESIAN_POINT('Ctrl Pts',(40.3014267406593,-8.23129907624866,-11.6635589380572));
#63795=CARTESIAN_POINT('Ctrl Pts',(40.3252504086465,-8.23351423423578,-11.651120080486));
#63796=CARTESIAN_POINT('Ctrl Pts',(40.3660588760584,-8.23736698471357,-11.6289350933298));
#63797=CARTESIAN_POINT('Ctrl Pts',(40.3831426909002,-8.238997938578,-11.6193756837645));
#63798=CARTESIAN_POINT('Ctrl Pts',(40.4180578303322,-8.24236989645333,-11.599275072546));
#63799=CARTESIAN_POINT('Ctrl Pts',(40.4358734093178,-8.24411164480865,-11.5887099634585));
#63800=CARTESIAN_POINT('Ctrl Pts',(40.4815647228206,-8.2486354051167,-11.5608099803201));
#63801=CARTESIAN_POINT('Ctrl Pts',(40.5092250447636,-8.25142957551763,-11.5431327925609));
#63802=CARTESIAN_POINT('Ctrl Pts',(40.6496393209387,-8.26591198361009,-11.4492951232816));
#63803=CARTESIAN_POINT('Ctrl Pts',(40.7561246750734,-8.27792499418585,-11.3642467793816));
#63804=CARTESIAN_POINT('Ctrl Pts',(40.944369117659,-8.30115569241861,-11.1857978445688));
#63805=CARTESIAN_POINT('Ctrl Pts',(41.0272419579355,-8.31230587164552,-11.0941593955072));
#63806=CARTESIAN_POINT('Ctrl Pts',(41.1360829728037,-8.32808246806383,-10.9534290454211));
#63807=CARTESIAN_POINT('Ctrl Pts',(41.1679722742019,-8.33287126147658,-10.9091651492865));
#63808=CARTESIAN_POINT('Ctrl Pts',(41.207922230718,-8.33906469165564,-10.8495369468115));
#63809=CARTESIAN_POINT('Ctrl Pts',(41.2173587760633,-8.34054307246339,-10.8351196241973));
#63810=CARTESIAN_POINT('Ctrl Pts',(41.2327237174883,-8.34297469220922,-10.8110850699198));
#63811=CARTESIAN_POINT('Ctrl Pts',(41.2387405876956,-8.34393335855134,-10.801525501894));
#63812=CARTESIAN_POINT('Ctrl Pts',(41.2509159434523,-8.34588609388394,-10.7818756723839));
#63813=CARTESIAN_POINT('Ctrl Pts',(41.2570677811711,-8.34687975039062,-10.7717817873244));
#63814=CARTESIAN_POINT('Ctrl Pts',(41.273280475595,-8.34951853759041,-10.7447334377515));
#63815=CARTESIAN_POINT('Ctrl Pts',(41.2832080326043,-8.35115554593282,-10.7276994469445));
#63816=CARTESIAN_POINT('Ctrl Pts',(41.3333662098905,-8.35954874560748,-10.6391516692073));
#63817=CARTESIAN_POINT('Ctrl Pts',(41.3701330254643,-8.36612121499884,-10.5657264751803));
#63818=CARTESIAN_POINT('Ctrl Pts',(41.4655602476742,-8.38493811013668,-10.3479932160128));
#63819=CARTESIAN_POINT('Ctrl Pts',(41.5140566899546,-8.39695903170728,-10.1997030342007));
#63820=CARTESIAN_POINT('Ctrl Pts',(41.5654275823018,-8.41572311895518,-9.9689817522342));
#63821=CARTESIAN_POINT('Ctrl Pts',(41.5789906495108,-8.42220318112985,-9.88937407040343));
#63822=CARTESIAN_POINT('Ctrl Pts',(41.5918834934816,-8.43112989149296,-9.78103376744624));
#63823=CARTESIAN_POINT('Ctrl Pts',(41.5947402755858,-8.43346830152467,-9.75276920527259));
#63824=CARTESIAN_POINT('Ctrl Pts',(41.5987411404646,-8.4374663861597,-9.70468755128886));
#63825=CARTESIAN_POINT('Ctrl Pts',(41.6001417552086,-8.43911800571743,-9.6848942791888));
#63826=CARTESIAN_POINT('Ctrl Pts',(41.6023400688019,-8.44227457039063,-9.64721183001717));
#63827=CARTESIAN_POINT('Ctrl Pts',(41.6031831955961,-8.44377799702457,-9.62932654936618));
#63828=CARTESIAN_POINT('Ctrl Pts',(41.6046918816193,-8.44731815310019,-9.58736831309691));
#63829=CARTESIAN_POINT('Ctrl Pts',(41.6051957278988,-8.44935972361859,-9.56329192985939));
#63830=CARTESIAN_POINT('Ctrl Pts',(41.6057079777021,-8.45674998483878,-9.4766010606857));
#63831=CARTESIAN_POINT('Ctrl Pts',(41.6036330747786,-8.46216076257928,-9.41400512831191));
#63832=CARTESIAN_POINT('Ctrl Pts',(41.5835736399115,-8.48649938844244,-9.13652034207096));
#63833=CARTESIAN_POINT('Ctrl Pts',(41.5391821044146,-8.50615426264701,-8.92454779612619));
#63834=CARTESIAN_POINT('Ctrl Pts',(41.450358402793,-8.52968592411832,-8.67395861545585));
#63835=CARTESIAN_POINT('Ctrl Pts',(41.4320636291046,-8.53409618206888,-8.62707053562132));
#63836=CARTESIAN_POINT('Ctrl Pts',(41.4057246551034,-8.53988242761902,-8.56535782749339));
#63837=CARTESIAN_POINT('Ctrl Pts',(41.3989781481434,-8.54132103218477,-8.54999768895353));
#63838=CARTESIAN_POINT('Ctrl Pts',(41.3874573953104,-8.54370544457166,-8.52449578735511));
#63839=CARTESIAN_POINT('Ctrl Pts',(41.3827720796763,-8.54465626377964,-8.51431478333761));
#63840=CARTESIAN_POINT('Ctrl Pts',(41.3729391671339,-8.54661278486869,-8.49333561878766));
#63841=CARTESIAN_POINT('Ctrl Pts',(41.367781908375,-8.54761789973075,-8.48254250136713));
#63842=CARTESIAN_POINT('Ctrl Pts',(41.3536243409231,-8.55032231375158,-8.45347298504391));
#63843=CARTESIAN_POINT('Ctrl Pts',(41.3444717424969,-8.55201277170828,-8.43527114575487));
#63844=CARTESIAN_POINT('Ctrl Pts',(41.287386356406,-8.56222673593459,-8.32525046657764));
#63845=CARTESIAN_POINT('Ctrl Pts',(41.2337882994846,-8.57045334566809,-8.23647666372327));
#63846=CARTESIAN_POINT('Ctrl Pts',(41.0956213723443,-8.58949412233432,-8.03785072479634));
#63847=CARTESIAN_POINT('Ctrl Pts',(41.0069699058512,-8.60022463820565,-7.93130868984514));
#63848=CARTESIAN_POINT('Ctrl Pts',(40.8559193820491,-8.61729879914516,-7.77868410864893));
#63849=CARTESIAN_POINT('Ctrl Pts',(40.7996347986024,-8.62344122677296,-7.7269859398101));
#63850=CARTESIAN_POINT('Ctrl Pts',(40.7195575774502,-8.63197821629589,-7.66017375429541));
#63851=CARTESIAN_POINT('Ctrl Pts',(40.6978150984942,-8.63427697566421,-7.64266582210873));
#63852=CARTESIAN_POINT('Ctrl Pts',(40.6601748804735,-8.63822800299212,-7.61342147181324));
#63853=CARTESIAN_POINT('Ctrl Pts',(40.6444277975249,-8.63987267830823,-7.60149501172627));
#63854=CARTESIAN_POINT('Ctrl Pts',(40.6121239817596,-8.64323125161284,-7.57764925235708));
#63855=CARTESIAN_POINT('Ctrl Pts',(40.5955589716999,-8.64494551318919,-7.56574397389094));
#63856=CARTESIAN_POINT('Ctrl Pts',(40.5532130630552,-8.64930921117664,-7.53611943567535));
#63857=CARTESIAN_POINT('Ctrl Pts',(40.5272350341944,-8.65196918821372,-7.51869033817353));
#63858=CARTESIAN_POINT('Ctrl Pts',(40.4130721215735,-8.66359223010618,-7.44528407932634));
#63859=CARTESIAN_POINT('Ctrl Pts',(40.3216467031703,-8.67273866870194,-7.39458582807992));
#63860=CARTESIAN_POINT('Ctrl Pts',(40.0935723953588,-8.6951689036031,-7.28686897864534));
#63861=CARTESIAN_POINT('Ctrl Pts',(39.9543881480952,-8.70855893992475,-7.23620165720945));
#63862=CARTESIAN_POINT('Ctrl Pts',(39.7700044030205,-8.72552222665956,-7.1877402259859));
#63863=CARTESIAN_POINT('Ctrl Pts',(39.7282844788106,-8.72930920436744,-7.17795839934688));
#63864=CARTESIAN_POINT('Ctrl Pts',(39.6569324128432,-8.73567840210739,-7.16322813821743));
#63865=CARTESIAN_POINT('Ctrl Pts',(39.6274289405675,-8.73828112534517,-7.15771076865525));
#63866=CARTESIAN_POINT('Ctrl Pts',(39.5841491430127,-8.74204732005984,-7.15045272676392));
#63867=CARTESIAN_POINT('Ctrl Pts',(39.5704502120145,-8.74323184566089,-7.1482770489051));
#63868=CARTESIAN_POINT('Ctrl Pts',(39.5470574558826,-8.74524089813474,-7.14476896443429));
#63869=CARTESIAN_POINT('Ctrl Pts',(39.5373733805641,-8.74606857085188,-7.14337705008226));
#63870=CARTESIAN_POINT('Ctrl Pts',(39.5147458032615,-8.74799306535275,-7.14026552989884));
#63871=CARTESIAN_POINT('Ctrl Pts',(39.5017964072842,-8.74908734502324,-7.13859216257249));
#63872=CARTESIAN_POINT('Ctrl Pts',(39.4633426112578,-8.7523176555313,-7.13394104873244));
#63873=CARTESIAN_POINT('Ctrl Pts',(39.4378023597089,-8.7544381621786,-7.13126600511164));
#63874=CARTESIAN_POINT('Ctrl Pts',(39.2956381081665,-8.76612802966791,-7.11867398730389));
#63875=CARTESIAN_POINT('Ctrl Pts',(39.1784378413477,-8.7753459442424,-7.11686908431961));
#63876=CARTESIAN_POINT('Ctrl Pts',(38.9410866157831,-8.79399130468109,-7.13055263126393));
#63877=CARTESIAN_POINT('Ctrl Pts',(38.8213157290546,-8.80339273515776,-7.14655292626023));
#63878=CARTESIAN_POINT('Ctrl Pts',(38.6322370600079,-8.81878162505628,-7.18646063030293));
#63879=CARTESIAN_POINT('Ctrl Pts',(38.5619412705909,-8.82462612617245,-7.20465512849876));
#63880=CARTESIAN_POINT('Ctrl Pts',(38.4663443113245,-8.83281762599381,-7.23407096825798));
#63881=CARTESIAN_POINT('Ctrl Pts',(38.440248653903,-8.83507911984349,-7.24259244109609));
#63882=CARTESIAN_POINT('Ctrl Pts',(38.3957119791689,-8.83898616508868,-7.2579841776568));
#63883=CARTESIAN_POINT('Ctrl Pts',(38.3771984890805,-8.84062455245881,-7.26463773156211));
#63884=CARTESIAN_POINT('Ctrl Pts',(38.3395357914404,-8.84398814799495,-7.27869731171502));
#63885=CARTESIAN_POINT('Ctrl Pts',(38.3203956915924,-8.84571388357338,-7.28612290951717));
#63886=CARTESIAN_POINT('Ctrl Pts',(38.2717369420788,-8.85014462547898,-7.30572082084604));
#63887=CARTESIAN_POINT('Ctrl Pts',(38.2423623175846,-8.85286084099711,-7.31823715853267));
#63888=CARTESIAN_POINT('Ctrl Pts',(38.1053165669283,-8.86573706334251,-7.37988295872333));
#63889=CARTESIAN_POINT('Ctrl Pts',(38.001135476713,-8.87613765481072,-7.4363224881149));
#63890=CARTESIAN_POINT('Ctrl Pts',(37.801439105181,-8.89730863221659,-7.56438209788894));
#63891=CARTESIAN_POINT('Ctrl Pts',(37.7062347971764,-8.90805171406802,-7.63591037150568));
#63892=CARTESIAN_POINT('Ctrl Pts',(37.5784457791295,-8.92321088883573,-7.74764279939344));
#63893=CARTESIAN_POINT('Ctrl Pts',(37.5412468273952,-8.92772253753241,-7.78230801646997));
#63894=CARTESIAN_POINT('Ctrl Pts',(37.4811283027383,-8.93515033605419,-7.8420023476698));
#63895=CARTESIAN_POINT('Ctrl Pts',(37.457589942948,-8.93809595991985,-7.86638354444659));
#63896=CARTESIAN_POINT('Ctrl Pts',(37.4247023173413,-8.94225663751462,-7.90192197359008));
#63897=CARTESIAN_POINT('Ctrl Pts',(37.4149281686698,-8.94349911007786,-7.91267784490645));
#63898=CARTESIAN_POINT('Ctrl Pts',(37.3980108438776,-8.94565910848903,-7.93163679438678));
#63899=CARTESIAN_POINT('Ctrl Pts',(37.3908249745688,-8.94657961861338,-7.93980065271793));
#63900=CARTESIAN_POINT('Ctrl Pts',(37.3751377002543,-8.94859574575634,-7.9578685863311));
#63901=CARTESIAN_POINT('Ctrl Pts',(37.366661209268,-8.94968961053923,-7.96779346792477));
#63902=CARTESIAN_POINT('Ctrl Pts',(37.3417662135749,-8.95291737751067,-7.99742738102724));
#63903=CARTESIAN_POINT('Ctrl Pts',(37.3255810132762,-8.95503579196878,-8.01733142427825));
#63904=CARTESIAN_POINT('Ctrl Pts',(37.2450264833285,-8.9657053935844,-8.11969785772744));
#63905=CARTESIAN_POINT('Ctrl Pts',(37.1857588452718,-8.97397947296573,-8.20604808724587));
#63906=CARTESIAN_POINT('Ctrl Pts',(37.087028361216,-8.98915842577011,-8.37215427388057));
#63907=CARTESIAN_POINT('Ctrl Pts',(37.0460031090574,-8.99606679494006,-8.45075620351427));
#63908=CARTESIAN_POINT('Ctrl Pts',(36.9911539509655,-9.00652134797575,-8.57168736622732));
#63909=CARTESIAN_POINT('Ctrl Pts',(36.9740189001327,-9.01001361398599,-8.61241497730244));
#63910=CARTESIAN_POINT('Ctrl Pts',(36.9580196445751,-9.01353011641035,-8.65357758217454));
#63911=CARTESIAN_POINT('Origin',(39.2,8.05522481984854,-9.525));
#63912=CARTESIAN_POINT('',(36.958019684939,-10.5481760837449,-8.65357747832709));
#63913=CARTESIAN_POINT('',(36.9580196499262,-10.2836033739986,-8.65357756840738));
#63914=CARTESIAN_POINT('',(36.958019684865,8.05522481984854,-8.65357747851728));
#63915=CARTESIAN_POINT('',(36.794620234193,-9.35522481984856,-9.52393856416118));
#63916=CARTESIAN_POINT('Ctrl Pts',(36.958019684939,-10.5481760837449,-8.65357747832709));
#63917=CARTESIAN_POINT('Ctrl Pts',(36.9617940800382,-10.5472770356811,-8.64386678196179));
#63918=CARTESIAN_POINT('Ctrl Pts',(36.9656316767484,-10.5463810343756,-8.63418032043723));
#63919=CARTESIAN_POINT('Ctrl Pts',(36.9744232493849,-10.5443689686419,-8.61240383311359));
#63920=CARTESIAN_POINT('Ctrl Pts',(36.9794130521616,-10.5432548445178,-8.60032856197506));
#63921=CARTESIAN_POINT('Ctrl Pts',(36.9887368682618,-10.5412238092281,-8.57827585147578));
#63922=CARTESIAN_POINT('Ctrl Pts',(36.993040355656,-10.540305287641,-8.56828667307018));
#63923=CARTESIAN_POINT('Ctrl Pts',(37.0032471680292,-10.5381698972795,-8.54503021541096));
#63924=CARTESIAN_POINT('Ctrl Pts',(37.0092030852763,-10.5369561511453,-8.53178668216365));
#63925=CARTESIAN_POINT('Ctrl Pts',(37.0294181743284,-10.5329391486733,-8.48790331687982));
#63926=CARTESIAN_POINT('Ctrl Pts',(37.0442039027969,-10.5301647308001,-8.45750830262123));
#63927=CARTESIAN_POINT('Ctrl Pts',(37.0827314884524,-10.5233007687884,-8.38237538734461));
#63928=CARTESIAN_POINT('Ctrl Pts',(37.107255376584,-10.5192463126082,-8.33805531683175));
#63929=CARTESIAN_POINT('Ctrl Pts',(37.2308012985563,-10.5000738513962,-8.13053189905721));
#63930=CARTESIAN_POINT('Ctrl Pts',(37.3476119881842,-10.4854240899873,-7.97873157066489));
#63931=CARTESIAN_POINT('Ctrl Pts',(37.522672845037,-10.4653892921338,-7.79990533755317));
#63932=CARTESIAN_POINT('Ctrl Pts',(37.5657592104529,-10.4605876239119,-7.75903455987815));
#63933=CARTESIAN_POINT('Ctrl Pts',(37.6281276227031,-10.4537734694143,-7.70411180169745));
#63934=CARTESIAN_POINT('Ctrl Pts',(37.6461758521252,-10.4518167501323,-7.68868656337561));
#63935=CARTESIAN_POINT('Ctrl Pts',(37.6795458159023,-10.4482238036903,-7.66101053822831));
#63936=CARTESIAN_POINT('Ctrl Pts',(37.6947949256035,-10.4465911263317,-7.64867506124427));
#63937=CARTESIAN_POINT('Ctrl Pts',(37.726121059886,-10.4432543619239,-7.62396201354268));
#63938=CARTESIAN_POINT('Ctrl Pts',(37.742207212201,-10.4415498898669,-7.61159865946782));
#63939=CARTESIAN_POINT('Ctrl Pts',(37.7830280507703,-10.4372454530019,-7.58103850562135));
#63940=CARTESIAN_POINT('Ctrl Pts',(37.807957632509,-10.4346355351603,-7.56310967272344));
#63941=CARTESIAN_POINT('Ctrl Pts',(37.9208329336029,-10.422895043784,-7.48516665422902));
#63942=CARTESIAN_POINT('Ctrl Pts',(38.0123488530201,-10.4135720331113,-7.43056298306245));
#63943=CARTESIAN_POINT('Ctrl Pts',(38.1882442185085,-10.3960098730176,-7.34085561649105));
#63944=CARTESIAN_POINT('Ctrl Pts',(38.2716003716131,-10.3878248635031,-7.30414227070433));
#63945=CARTESIAN_POINT('Ctrl Pts',(38.45558357101,-10.370175925564,-7.23528053283743));
#63946=CARTESIAN_POINT('Ctrl Pts',(38.5566702979195,-10.3607320609294,-7.20484853907379));
#63947=CARTESIAN_POINT('Ctrl Pts',(38.6844766904349,-10.3493076526327,-7.17537259514505));
#63948=CARTESIAN_POINT('Ctrl Pts',(38.7096078057195,-10.3470857526408,-7.1699991759541));
#63949=CARTESIAN_POINT('Ctrl Pts',(38.7476376875347,-10.3437647909215,-7.16250303413089));
#63950=CARTESIAN_POINT('Ctrl Pts',(38.7604745014706,-10.3426508774321,-7.16008119883126));
#63951=CARTESIAN_POINT('Ctrl Pts',(38.7840365716084,-10.3406199457246,-7.15583438609));
#63952=CARTESIAN_POINT('Ctrl Pts',(38.7947549822719,-10.3397013202964,-7.15397748512991));
#63953=CARTESIAN_POINT('Ctrl Pts',(38.8198168862019,-10.3375652530155,-7.14981057904506));
#63954=CARTESIAN_POINT('Ctrl Pts',(38.8341692606762,-10.3363509393952,-7.14755770028923));
#63955=CARTESIAN_POINT('Ctrl Pts',(38.8820156119236,-10.332329850656,-7.14049086430308));
#63956=CARTESIAN_POINT('Ctrl Pts',(38.9155926427797,-10.3295519945498,-7.13625332229212));
#63957=CARTESIAN_POINT('Ctrl Pts',(38.9997022074193,-10.3226773067431,-7.12743726084013));
#63958=CARTESIAN_POINT('Ctrl Pts',(39.0503126204247,-10.3186157049019,-7.12374600052062));
#63959=CARTESIAN_POINT('Ctrl Pts',(39.2826908550674,-10.300153916378,-7.11417426852147));
#63960=CARTESIAN_POINT('Ctrl Pts',(39.4646370330087,-10.286177500558,-7.12731600651833));
#63961=CARTESIAN_POINT('Ctrl Pts',(39.7082488838147,-10.2663941915519,-7.17300221878139));
#63962=CARTESIAN_POINT('Ctrl Pts',(39.7725951872106,-10.2610690557433,-7.18783423850404));
#63963=CARTESIAN_POINT('Ctrl Pts',(39.8625284554224,-10.2534300364104,-7.21250096916805));
#63964=CARTESIAN_POINT('Ctrl Pts',(39.888686152377,-10.2511843767762,-7.22015575737469));
#63965=CARTESIAN_POINT('Ctrl Pts',(39.9332770612134,-10.2473117631226,-7.23403166053559));
#63966=CARTESIAN_POINT('Ctrl Pts',(39.9517756756488,-10.2456919317577,-7.24003512766715));
#63967=CARTESIAN_POINT('Ctrl Pts',(39.9896661285934,-10.2423454071276,-7.25284185926933));
#63968=CARTESIAN_POINT('Ctrl Pts',(40.0090475747856,-10.2406180004534,-7.25967062510547));
#63969=CARTESIAN_POINT('Ctrl Pts',(40.0583877829925,-10.2361788523927,-7.27776885795176));
#63970=CARTESIAN_POINT('Ctrl Pts',(40.0882124252737,-10.233455822443,-7.28938915117906));
#63971=CARTESIAN_POINT('Ctrl Pts',(40.2383347973881,-10.2195386369256,-7.35135801289239));
#63972=CARTESIAN_POINT('Ctrl Pts',(40.3546059034522,-10.2080467966561,-7.41082592155569));
#63973=CARTESIAN_POINT('Ctrl Pts',(40.5785310510507,-10.1844926843788,-7.54935309821659));
#63974=CARTESIAN_POINT('Ctrl Pts',(40.6856013191408,-10.1724637933771,-7.62855112747738));
#63975=CARTESIAN_POINT('Ctrl Pts',(40.824604694199,-10.1560849996368,-7.75039986586704));
#63976=CARTESIAN_POINT('Ctrl Pts',(40.8625157233103,-10.151530729951,-7.78586556626632));
#63977=CARTESIAN_POINT('Ctrl Pts',(40.9115761107257,-10.145547882651,-7.83483334931611));
#63978=CARTESIAN_POINT('Ctrl Pts',(40.9237658741182,-10.1440536291517,-7.84726719777123));
#63979=CARTESIAN_POINT('Ctrl Pts',(40.9428896340482,-10.1416984848065,-7.86720237781049));
#63980=CARTESIAN_POINT('Ctrl Pts',(40.9499123870889,-10.1408312233466,-7.87461704981788));
#63981=CARTESIAN_POINT('Ctrl Pts',(40.9647118087771,-10.1389989050201,-7.89044305997697));
#63982=CARTESIAN_POINT('Ctrl Pts',(40.9724760659392,-10.1380348279483,-7.89886569781726));
#63983=CARTESIAN_POINT('Ctrl Pts',(40.992286676239,-10.1355667239808,-7.92066665406841));
#63984=CARTESIAN_POINT('Ctrl Pts',(41.004243889023,-10.1340690510318,-7.9341256921298));
#63985=CARTESIAN_POINT('Ctrl Pts',(41.0571795100254,-10.12739543117,-7.99507466851855));
#63986=CARTESIAN_POINT('Ctrl Pts',(41.0964463891134,-10.1223261527214,-8.04402729016236));
#63987=CARTESIAN_POINT('Ctrl Pts',(41.2202168738326,-10.1057176448463,-8.21133685118462));
#63988=CARTESIAN_POINT('Ctrl Pts',(41.2959066539736,-10.0944725374643,-8.33581226783064));
#63989=CARTESIAN_POINT('Ctrl Pts',(41.4070036138665,-10.0745939711146,-8.56247997881646));
#63990=CARTESIAN_POINT('Ctrl Pts',(41.4476377485976,-10.0660805265843,-8.66161744501087));
#63991=CARTESIAN_POINT('Ctrl Pts',(41.491495524814,-10.0547839971975,-8.79295459457397));
#63992=CARTESIAN_POINT('Ctrl Pts',(41.5008712378666,-10.0522009732421,-8.82297893348488));
#63993=CARTESIAN_POINT('Ctrl Pts',(41.515363171757,-10.0479083883193,-8.87280064987866));
#63994=CARTESIAN_POINT('Ctrl Pts',(41.5208206752382,-10.0462098947368,-8.89249549481313));
#63995=CARTESIAN_POINT('Ctrl Pts',(41.5310541170087,-10.0428551107256,-8.93134253255975));
#63996=CARTESIAN_POINT('Ctrl Pts',(41.5358465787012,-10.0411994950142,-8.95048873268257));
#63997=CARTESIAN_POINT('Ctrl Pts',(41.5468206884597,-10.0371934950487,-8.99674017662814));
#63998=CARTESIAN_POINT('Ctrl Pts',(41.552768922648,-10.0348359477567,-9.02389717416046));
#63999=CARTESIAN_POINT('Ctrl Pts',(41.5730979672251,-10.02602881308,-9.12507025077084));
#64000=CARTESIAN_POINT('Ctrl Pts',(41.5844654080335,-10.019488163995,-9.19963881468357));
#64001=CARTESIAN_POINT('Ctrl Pts',(41.6063421594812,-10.0010026183094,-9.4086567564682));
#64002=CARTESIAN_POINT('Ctrl Pts',(41.6090794607252,-9.98887829976523,-9.54363325619523));
#64003=CARTESIAN_POINT('Ctrl Pts',(41.5936031465559,-9.96704373995819,-9.78627214944001));
#64004=CARTESIAN_POINT('Ctrl Pts',(41.5794011660872,-9.95735461240898,-9.89385662884896));
#64005=CARTESIAN_POINT('Ctrl Pts',(41.5539589993196,-9.94619583057232,-10.0201221711368));
#64006=CARTESIAN_POINT('Ctrl Pts',(41.5496759170829,-9.94443998410839,-10.0400651457396));
#64007=CARTESIAN_POINT('Ctrl Pts',(41.5424777267598,-9.9416746446538,-10.071620786504));
#64008=CARTESIAN_POINT('Ctrl Pts',(41.5397288573405,-9.94065661836519,-10.083269717966));
#64009=CARTESIAN_POINT('Ctrl Pts',(41.5342376778165,-9.93869488463575,-10.105786551795));
#64010=CARTESIAN_POINT('Ctrl Pts',(41.5315061910978,-9.93775067214095,-10.1166565264216));
#64011=CARTESIAN_POINT('Ctrl Pts',(41.5244986800392,-9.93540418742908,-10.1437406522502));
#64012=CARTESIAN_POINT('Ctrl Pts',(41.5201287793553,-9.93400707040984,-10.1599303934326));
#64013=CARTESIAN_POINT('Ctrl Pts',(41.5019945811145,-9.92845835596267,-10.2244259429448));
#64014=CARTESIAN_POINT('Ctrl Pts',(41.4868869044157,-9.92437400293287,-10.272345300723));
#64015=CARTESIAN_POINT('Ctrl Pts',(41.3989475470494,-9.90298886321175,-10.5235499768259));
#64016=CARTESIAN_POINT('Ctrl Pts',(41.3004915580736,-9.88654338108804,-10.7168146022263));
#64017=CARTESIAN_POINT('Ctrl Pts',(41.142025084017,-9.86428891187898,-10.9456641222148));
#64018=CARTESIAN_POINT('Ctrl Pts',(41.1045153843572,-9.85924720532869,-10.9955671974628));
#64019=CARTESIAN_POINT('Ctrl Pts',(41.0499101822128,-9.85215982858639,-11.0626165633304));
#64020=CARTESIAN_POINT('Ctrl Pts',(41.0344307861134,-9.85017659942571,-11.0810514080777));
#64021=CARTESIAN_POINT('Ctrl Pts',(41.0069590010383,-9.84669877990423,-11.1127886303995));
#64022=CARTESIAN_POINT('Ctrl Pts',(40.995089640264,-9.84520923072148,-11.1261954013841));
#64023=CARTESIAN_POINT('Ctrl Pts',(40.9697477932711,-9.84205511770859,-11.1541837775884));
#64024=CARTESIAN_POINT('Ctrl Pts',(40.9562423224549,-9.84038925692244,-11.1687335207685));
#64025=CARTESIAN_POINT('Ctrl Pts',(40.9229560450303,-9.83631829915349,-11.2037150083473));
#64026=CARTESIAN_POINT('Ctrl Pts',(40.9029905055498,-9.83390544839181,-11.2239658034489));
#64027=CARTESIAN_POINT('Ctrl Pts',(40.824829431575,-9.82456438149032,-11.300481428066));
#64028=CARTESIAN_POINT('Ctrl Pts',(40.7641736385596,-9.81752979043384,-11.3541426000984));
#64029=CARTESIAN_POINT('Ctrl Pts',(40.5785047596695,-9.79658175681074,-11.5024035769155));
#64030=CARTESIAN_POINT('Ctrl Pts',(40.4468215228621,-9.78241488299629,-11.58796574652));
#64031=CARTESIAN_POINT('Ctrl Pts',(40.2360295279814,-9.7611736992508,-11.6973325575484));
#64032=CARTESIAN_POINT('Ctrl Pts',(40.1624447608922,-9.7540050842331,-11.7309213887749));
#64033=CARTESIAN_POINT('Ctrl Pts',(40.069012631137,-9.74530382552355,-11.7680018031981));
#64034=CARTESIAN_POINT('Ctrl Pts',(40.0506360904107,-9.74361122996381,-11.7750351909826));
#64035=CARTESIAN_POINT('Ctrl Pts',(40.0210902668807,-9.74092198060536,-11.7859297381599));
#64036=CARTESIAN_POINT('Ctrl Pts',(40.0099757828261,-9.73991754412972,-11.7899352655416));
#64037=CARTESIAN_POINT('Ctrl Pts',(39.9881688247258,-9.73796145018396,-11.7976131750646));
#64038=CARTESIAN_POINT('Ctrl Pts',(39.9774792388317,-9.73700946800847,-11.8012923326884));
#64039=CARTESIAN_POINT('Ctrl Pts',(39.9503965567882,-9.73461396267094,-11.810400652182));
#64040=CARTESIAN_POINT('Ctrl Pts',(39.9339697189982,-9.73317607279061,-11.8157290626079));
#64041=CARTESIAN_POINT('Ctrl Pts',(39.8651005550662,-9.72720479884732,-11.8372513838694));
#64042=CARTESIAN_POINT('Ctrl Pts',(39.8121642880277,-9.72275231909575,-11.8518264601564));
#64043=CARTESIAN_POINT('Ctrl Pts',(39.640287380292,-9.7085921309835,-11.8928764562191));
#64044=CARTESIAN_POINT('Ctrl Pts',(39.5198168892167,-9.69910990610688,-11.9121350400517));
#64045=CARTESIAN_POINT('Ctrl Pts',(39.2720406308413,-9.67961969546622,-11.9326417025696));
#64046=CARTESIAN_POINT('Ctrl Pts',(39.1450701988678,-9.66963364297617,-11.9330915589169));
#64047=CARTESIAN_POINT('Ctrl Pts',(38.9808679185907,-9.65627350106521,-11.9206775558384));
#64048=CARTESIAN_POINT('Ctrl Pts',(38.9431446465176,-9.65317450966836,-11.9169270128237));
#64049=CARTESIAN_POINT('Ctrl Pts',(38.883725001822,-9.64823647720225,-11.909597588981));
#64050=CARTESIAN_POINT('Ctrl Pts',(38.8619609144421,-9.64641572807348,-11.9066097594778));
#64051=CARTESIAN_POINT('Ctrl Pts',(38.8213975626643,-9.64299790976286,-11.9004739230374));
#64052=CARTESIAN_POINT('Ctrl Pts',(38.802588728532,-9.64140326751076,-11.8973997136829));
#64053=CARTESIAN_POINT('Ctrl Pts',(38.7600151002384,-9.6377702863768,-11.8899207899825));
#64054=CARTESIAN_POINT('Ctrl Pts',(38.7362765673883,-9.63572785811218,-11.8853808043069));
#64055=CARTESIAN_POINT('Ctrl Pts',(38.6630789974455,-9.62937562810909,-11.8702350163411));
#64056=CARTESIAN_POINT('Ctrl Pts',(38.6138864504958,-9.62502895838328,-11.8584269938047));
#64057=CARTESIAN_POINT('Ctrl Pts',(38.4971933890948,-9.6145217455718,-11.8264937261181));
#64058=CARTESIAN_POINT('Ctrl Pts',(38.4301358487702,-9.60832272945565,-11.8049381294784));
#64059=CARTESIAN_POINT('Ctrl Pts',(38.2778280882835,-9.59388048457267,-11.7484932153076));
#64060=CARTESIAN_POINT('Ctrl Pts',(38.1934407173553,-9.58560423990945,-11.7115863592595));
#64061=CARTESIAN_POINT('Ctrl Pts',(38.0169567869119,-9.56782316210305,-11.6220154993521));
#64062=CARTESIAN_POINT('Ctrl Pts',(37.9257905002492,-9.55833839139738,-11.5679048657617));
#64063=CARTESIAN_POINT('Ctrl Pts',(37.8173108084081,-9.54687690179493,-11.4934214189966));
#64064=CARTESIAN_POINT('Ctrl Pts',(37.7963753985365,-9.54465661025689,-11.4785481622657));
#64065=CARTESIAN_POINT('Ctrl Pts',(37.7651580285667,-9.54133759851847,-11.4556092258415));
#64066=CARTESIAN_POINT('Ctrl Pts',(37.754697871366,-9.54022404905476,-11.447791004591));
#64067=CARTESIAN_POINT('Ctrl Pts',(37.735957291353,-9.5382271269469,-11.4335444075183));
#64068=CARTESIAN_POINT('Ctrl Pts',(37.7276547833192,-9.53734184818155,-11.427146782176));
#64069=CARTESIAN_POINT('Ctrl Pts',(37.7191393668961,-9.53643311376151,-11.4204959335104));
#64070=CARTESIAN_POINT('Ctrl Pts',(37.7188849673564,-9.53640596442008,-11.4202971557803));
#64071=CARTESIAN_POINT('Ctrl Pts',(37.718393885222,-9.53635355502442,-11.4199132843828));
#64072=CARTESIAN_POINT('Ctrl Pts',(37.7181571973048,-9.53632829450292,-11.4197281975995));
#64073=CARTESIAN_POINT('Ctrl Pts',(37.7176990352709,-9.53627939587673,-11.4193697826603));
#64074=CARTESIAN_POINT('Ctrl Pts',(37.7174775568987,-9.53625575739953,-11.4191964600311));
#64075=CARTESIAN_POINT('Ctrl Pts',(37.7170477493988,-9.53620988273649,-11.4188599834352));
#64076=CARTESIAN_POINT('Ctrl Pts',(37.7168394168242,-9.5361876462497,-11.4186968339557));
#64077=CARTESIAN_POINT('Ctrl Pts',(37.7164341791138,-9.5361443919746,-11.4183793761634));
#64078=CARTESIAN_POINT('Ctrl Pts',(37.7162372711094,-9.53612337393552,-11.4182250714952));
#64079=CARTESIAN_POINT('Ctrl Pts',(37.7158534316952,-9.53608240184531,-11.4179241835369));
#64080=CARTESIAN_POINT('Ctrl Pts',(37.715666497948,-9.53606244759097,-11.41777760329));
#64081=CARTESIAN_POINT('Ctrl Pts',(37.715301373173,-9.53602347148798,-11.417491210864));
#64082=CARTESIAN_POINT('Ctrl Pts',(37.7151231801841,-9.53600444946892,-11.417351401213));
#64083=CARTESIAN_POINT('Ctrl Pts',(37.7147744782518,-9.53596722493105,-11.4170777312097));
#64084=CARTESIAN_POINT('Ctrl Pts',(37.7146039676735,-9.53594902227067,-11.416943872989));
#64085=CARTESIAN_POINT('Ctrl Pts',(37.714269714768,-9.53591333877643,-11.4166813968791));
#64086=CARTESIAN_POINT('Ctrl Pts',(37.7141059710487,-9.535895857822,-11.4165527807812));
#64087=CARTESIAN_POINT('Ctrl Pts',(37.7137844534175,-9.53586153257664,-11.4163001701908));
#64088=CARTESIAN_POINT('Ctrl Pts',(37.7136266783115,-9.53584468818219,-11.4161761772082));
#64089=CARTESIAN_POINT('Ctrl Pts',(37.7133163964864,-9.53581156123753,-11.4159322687716));
#64090=CARTESIAN_POINT('Ctrl Pts',(37.7131638887586,-9.5357952786002,-11.4158123546102));
#64091=CARTESIAN_POINT('Ctrl Pts',(37.7128635209995,-9.53576320895746,-11.4155761218789));
#64092=CARTESIAN_POINT('Ctrl Pts',(37.7127156601183,-9.535747421879,-11.415459804422));
#64093=CARTESIAN_POINT('Ctrl Pts',(37.7124240329479,-9.53571628434737,-11.4152303352028));
#64094=CARTESIAN_POINT('Ctrl Pts',(37.7122802659038,-9.53570093382884,-11.4151171843706));
#64095=CARTESIAN_POINT('Ctrl Pts',(37.7119963299236,-9.53567061644701,-11.414893662106));
#64096=CARTESIAN_POINT('Ctrl Pts',(37.7118561603564,-9.53565564952944,-11.4147832914808));
#64097=CARTESIAN_POINT('Ctrl Pts',(37.7115789705714,-9.5356260514677,-11.4145649800894));
#64098=CARTESIAN_POINT('Ctrl Pts',(37.7114419498324,-9.53561142027915,-11.4144570400269));
#64099=CARTESIAN_POINT('Ctrl Pts',(37.7111706492607,-9.53558245009166,-11.4142432712618));
#64100=CARTESIAN_POINT('Ctrl Pts',(37.7110363689745,-9.53556811105396,-11.4141374431508));
#64101=CARTESIAN_POINT('Ctrl Pts',(37.7107701749681,-9.53553968522004,-11.4139276060386));
#64102=CARTESIAN_POINT('Ctrl Pts',(37.7106382608219,-9.53552559838653,-11.4138235975049));
#64103=CARTESIAN_POINT('Ctrl Pts',(37.7103764532939,-9.53549764005506,-11.4136171292427));
#64104=CARTESIAN_POINT('Ctrl Pts',(37.7102465596171,-9.53548376853252,-11.4135146699557));
#64105=CARTESIAN_POINT('Ctrl Pts',(37.7099884715763,-9.53545620651247,-11.4133110485913));
#64106=CARTESIAN_POINT('Ctrl Pts',(37.7098602769393,-9.53544251599159,-11.4132098868569));
#64107=CARTESIAN_POINT('Ctrl Pts',(37.7096052856644,-9.53541528381059,-11.4130086244448));
#64108=CARTESIAN_POINT('Ctrl Pts',(37.7094784888461,-9.53540174213591,-11.4129085240776));
#64109=CARTESIAN_POINT('Ctrl Pts',(37.7092260089581,-9.53537477730123,-11.412709161307));
#64110=CARTESIAN_POINT('Ctrl Pts',(37.7091003256796,-9.53536135412265,-11.4126098990948));
#64111=CARTESIAN_POINT('Ctrl Pts',(37.7088498023637,-9.53533459739803,-11.4124120000158));
#64112=CARTESIAN_POINT('Ctrl Pts',(37.7087249621897,-9.53532126384019,-11.4123133633073));
#64113=CARTESIAN_POINT('Ctrl Pts',(37.7084758657394,-9.53529465866364,-11.4121165110835));
#64114=CARTESIAN_POINT('Ctrl Pts',(37.7083516094116,-9.53528138704137,-11.4120182957091));
#64115=CARTESIAN_POINT('Ctrl Pts',(37.7081034302298,-9.53525487899175,-11.4118220887161));
#64116=CARTESIAN_POINT('Ctrl Pts',(37.7079795073268,-9.53524164256025,-11.4117240971595));
#64117=CARTESIAN_POINT('Ctrl Pts',(37.707731751225,-9.5352151788554,-11.4115281453052));
#64118=CARTESIAN_POINT('Ctrl Pts',(37.7076079179756,-9.53520195157689,-11.4114301849901));
#64119=CARTESIAN_POINT('Ctrl Pts',(37.707360101928,-9.53517548062033,-11.411234106383));
#64120=CARTESIAN_POINT('Ctrl Pts',(37.7072361191475,-9.5351622369436,-11.411135988051));
#64121=CARTESIAN_POINT('Ctrl Pts',(37.7069877674696,-9.53513570791645,-11.410939405993));
#64122=CARTESIAN_POINT('Ctrl Pts',(37.7068633986696,-9.53512242257502,-11.4108409422139));
#64123=CARTESIAN_POINT('Ctrl Pts',(37.7066140393411,-9.53509578504317,-11.4106434822971));
#64124=CARTESIAN_POINT('Ctrl Pts',(37.7064890489464,-9.53508243286479,-11.4105444860586));
#64125=CARTESIAN_POINT('Ctrl Pts',(37.7062382100754,-9.53505563640113,-11.4103457733642));
#64126=CARTESIAN_POINT('Ctrl Pts',(37.7061123617213,-9.5350421921258,-11.4102460567203));
#64127=CARTESIAN_POINT('Ctrl Pts',(37.7058595679992,-9.53501518593132,-11.4100457130005));
#64128=CARTESIAN_POINT('Ctrl Pts',(37.7057326227893,-9.53500162402505,-11.4099450856842));
#64129=CARTESIAN_POINT('Ctrl Pts',(37.7054773921606,-9.53497435657274,-11.4097427267039));
#64130=CARTESIAN_POINT('Ctrl Pts',(37.7053491069636,-9.53496065104545,-11.4096409947659));
#64131=CARTESIAN_POINT('Ctrl Pts',(37.705090947254,-9.53493306971971,-11.4094362276027));
#64132=CARTESIAN_POINT('Ctrl Pts',(37.7049610730091,-9.53491919394393,-11.4093331920511));
#64133=CARTESIAN_POINT('Ctrl Pts',(37.704699478435,-9.53489124466718,-11.40912561229));
#64134=CARTESIAN_POINT('Ctrl Pts',(37.7045677584072,-9.53487717119138,-11.409021067686));
#64135=CARTESIAN_POINT('Ctrl Pts',(37.7043022059747,-9.53484879803863,-11.4088102565151));
#64136=CARTESIAN_POINT('Ctrl Pts',(37.7041683739216,-9.53483449839102,-11.4087039894918));
#64137=CARTESIAN_POINT('Ctrl Pts',(37.7038983197439,-9.53480564319569,-11.4084895107224));
#64138=CARTESIAN_POINT('Ctrl Pts',(37.703762098019,-9.53479108768116,-11.4083812984475));
#64139=CARTESIAN_POINT('Ctrl Pts',(37.7034869733554,-9.53476168961095,-11.4081626952983));
#64140=CARTESIAN_POINT('Ctrl Pts',(37.7033480708792,-9.53474684709377,-11.4080523038246));
#64141=CARTESIAN_POINT('Ctrl Pts',(37.7030672779629,-9.53471684220376,-11.4078290955249));
#64142=CARTESIAN_POINT('Ctrl Pts',(37.7029253880609,-9.53470167987597,-11.4077162780271));
#64143=CARTESIAN_POINT('Ctrl Pts',(37.7026382955425,-9.5346710006205,-11.4074879560967));
#64144=CARTESIAN_POINT('Ctrl Pts',(37.702493093567,-9.5346554837471,-11.4073724509274));
#64145=CARTESIAN_POINT('Ctrl Pts',(37.7021990317842,-9.53462405847275,-11.4071384753005));
#64146=CARTESIAN_POINT('Ctrl Pts',(37.7020501726482,-9.53460815012737,-11.4070200039668));
#64147=CARTESIAN_POINT('Ctrl Pts',(37.7017484280631,-9.53457590247677,-11.4067797984307));
#64148=CARTESIAN_POINT('Ctrl Pts',(37.7015955433796,-9.534559563235,-11.4066580632445));
#64149=CARTESIAN_POINT('Ctrl Pts',(37.701285352924,-9.53452641154047,-11.4064110107814));
#64150=CARTESIAN_POINT('Ctrl Pts',(37.7011280479947,-9.53450959915693,-11.4062856923767));
#64151=CARTESIAN_POINT('Ctrl Pts',(37.6908226299531,-9.5334081555033,-11.3980736742179));
#64152=CARTESIAN_POINT('Ctrl Pts',(37.6807397676496,-9.53232893322692,-11.3899047407382));
#64153=CARTESIAN_POINT('Ctrl Pts',(37.6551096457665,-9.52958006986955,-11.3687938906684));
#64154=CARTESIAN_POINT('Ctrl Pts',(37.6396582496571,-9.52791759593007,-11.3557364131491));
#64155=CARTESIAN_POINT('Ctrl Pts',(37.5941074697056,-9.52299406482568,-11.3162472001429));
#64156=CARTESIAN_POINT('Ctrl Pts',(37.5645001959115,-9.51976382532131,-11.289255702678));
#64157=CARTESIAN_POINT('Ctrl Pts',(37.4437735190235,-9.50639330777485,-11.1735425343538));
#64158=CARTESIAN_POINT('Ctrl Pts',(37.35908429678,-9.49651381648505,-11.0784020242759));
#64159=CARTESIAN_POINT('Ctrl Pts',(37.2049198972074,-9.47647317360568,-10.8747943171741));
#64160=CARTESIAN_POINT('Ctrl Pts',(37.1358353763201,-9.46634017822809,-10.7665742172343));
#64161=CARTESIAN_POINT('Ctrl Pts',(37.060618810308,-9.45326726000504,-10.6249707271652));
#64162=CARTESIAN_POINT('Ctrl Pts',(37.0461024678045,-9.45062713929764,-10.5962668665065));
#64163=CARTESIAN_POINT('Ctrl Pts',(37.0232486224848,-9.44626525756486,-10.5487333469737));
#64164=CARTESIAN_POINT('Ctrl Pts',(37.0145693018241,-9.44455531067995,-10.5300717058368));
#64165=CARTESIAN_POINT('Ctrl Pts',(36.9980729350458,-9.44119654996351,-10.4933781916159));
#64166=CARTESIAN_POINT('Ctrl Pts',(36.9902352938204,-9.43954858926488,-10.4753573095408));
#64167=CARTESIAN_POINT('Ctrl Pts',(36.9720371232814,-9.43559276228321,-10.4320721704194));
#64168=CARTESIAN_POINT('Ctrl Pts',(36.9618845221947,-9.43327818522174,-10.4067241509388));
#64169=CARTESIAN_POINT('Ctrl Pts',(36.9267506914632,-9.42485891476378,-10.3144862336465));
#64170=CARTESIAN_POINT('Ctrl Pts',(36.9043218158565,-9.41867346592441,-10.2466719443444));
#64171=CARTESIAN_POINT('Ctrl Pts',(36.8249215104112,-9.39299183020817,-9.96516313493678));
#64172=CARTESIAN_POINT('Ctrl Pts',(36.7945377921274,-9.37278413225306,-9.74514521522786));
#64173=CARTESIAN_POINT('Ctrl Pts',(36.7946201670303,-9.35334798476491,-9.52410359447376));
#64174=CARTESIAN_POINT('Ctrl Pts',(36.958019684865,-9.28019056162069,-8.65357747851727));
#64175=CARTESIAN_POINT('Ctrl Pts',(36.9289224805849,-9.28692938518685,-8.72843824652977));
#64176=CARTESIAN_POINT('Ctrl Pts',(36.9036005899486,-9.29366820875302,-8.80470176169028));
#64177=CARTESIAN_POINT('Ctrl Pts',(36.8821687559105,-9.30040703231919,-8.88195158166545));
#64178=CARTESIAN_POINT('Ctrl Pts',(36.8606985388854,-9.30715792466944,-8.95933975092211));
#64179=CARTESIAN_POINT('Ctrl Pts',(36.8431324023123,-9.3139088170197,-9.03771729852912));
#64180=CARTESIAN_POINT('Ctrl Pts',(36.8295340594686,-9.32065970936996,-9.11665679976179));
#64181=CARTESIAN_POINT('Ctrl Pts',(36.8167488311576,-9.32700693130675,-9.19087610410068));
#64182=CARTESIAN_POINT('Ctrl Pts',(36.8074706247743,-9.33335415324353,-9.26559177363659));
#64183=CARTESIAN_POINT('Ctrl Pts',(36.8017103682723,-9.33970137518032,-9.34044706247925));
#64184=CARTESIAN_POINT('Ctrl Pts',(36.7970144018598,-9.3448758567364,-9.40147176200123));
#64185=CARTESIAN_POINT('Ctrl Pts',(36.7946472670224,-9.35005033829248,-9.46267794094415));
#64186=CARTESIAN_POINT('Ctrl Pts',(36.794620234193,-9.35522481984856,-9.52393856416118));
#64187=CARTESIAN_POINT('Ctrl Pts',(36.9580196445751,-9.01353011641035,-8.65357758217454));
#64188=CARTESIAN_POINT('Ctrl Pts',(36.9344154253712,-9.01871812617473,-8.71430610450518));
#64189=CARTESIAN_POINT('Ctrl Pts',(36.9132833758058,-9.02395946760844,-8.77598138396043));
#64190=CARTESIAN_POINT('Ctrl Pts',(36.8858593972149,-9.03180206969371,-8.86806699597638));
#64191=CARTESIAN_POINT('Ctrl Pts',(36.8776119862505,-9.03434065224797,-8.89784655849278));
#64192=CARTESIAN_POINT('Ctrl Pts',(36.8648949952305,-9.0385791582975,-8.94746162913789));
#64193=CARTESIAN_POINT('Ctrl Pts',(36.860099010553,-9.04026858181975,-8.96721038032214));
#64194=CARTESIAN_POINT('Ctrl Pts',(36.8511749069007,-9.04360142395969,-9.00610022573707));
#64195=CARTESIAN_POINT('Ctrl Pts',(36.8470291397489,-9.0452441409354,-9.02523567943694));
#64196=CARTESIAN_POINT('Ctrl Pts',(36.8375154918164,-9.04925763275802,-9.07189285179437));
#64197=CARTESIAN_POINT('Ctrl Pts',(36.8323945090578,-9.0516359449842,-9.09946124091152));
#64198=CARTESIAN_POINT('Ctrl Pts',(36.8159434184982,-9.06012583016564,-9.19754399402646));
#64199=CARTESIAN_POINT('Ctrl Pts',(36.8072739715262,-9.06631723385933,-9.26845922591632));
#64200=CARTESIAN_POINT('Ctrl Pts',(36.7862056400851,-9.0903382419935,-9.5410572169643));
#64201=CARTESIAN_POINT('Ctrl Pts',(36.7960737208553,-9.10873208830279,-9.74359297967492));
#64202=CARTESIAN_POINT('Ctrl Pts',(36.8400888654692,-9.13119095692045,-9.99333444517529));
#64203=CARTESIAN_POINT('Ctrl Pts',(36.8506838196181,-9.13571845453083,-10.0438759546695));
#64204=CARTESIAN_POINT('Ctrl Pts',(36.8669012853634,-9.14163130888702,-10.1104824013506));
#64205=CARTESIAN_POINT('Ctrl Pts',(36.871077766535,-9.14308264206995,-10.1268808315412));
#64206=CARTESIAN_POINT('Ctrl Pts',(36.8783146378802,-9.14548212313217,-10.1540915968782));
#64207=CARTESIAN_POINT('Ctrl Pts',(36.8812782900394,-9.14643541513576,-10.1649287558959));
#64208=CARTESIAN_POINT('Ctrl Pts',(36.887541153998,-9.14839051940489,-10.1872152055491));
#64209=CARTESIAN_POINT('Ctrl Pts',(36.8908496765499,-9.14939180205943,-10.1986614102247));
#64210=CARTESIAN_POINT('Ctrl Pts',(36.8999826216678,-9.1520742513772,-10.2293998053138));
#64211=CARTESIAN_POINT('Ctrl Pts',(36.905964828167,-9.15374682011653,-10.2486447600623));
#64212=CARTESIAN_POINT('Ctrl Pts',(36.9408847256793,-9.16306757444108,-10.3561955425281));
#64213=CARTESIAN_POINT('Ctrl Pts',(36.974682692969,-9.17047846023004,-10.4428538484939));
#64214=CARTESIAN_POINT('Ctrl Pts',(37.0745286436771,-9.18938183345089,-10.6606635654465));
#64215=CARTESIAN_POINT('Ctrl Pts',(37.1477032239511,-9.20073257884713,-10.7881065149531));
#64216=CARTESIAN_POINT('Ctrl Pts',(37.2772019709056,-9.21862531889779,-10.9723675120115));
#64217=CARTESIAN_POINT('Ctrl Pts',(37.3254922330012,-9.22493757626348,-11.0343850744063));
#64218=CARTESIAN_POINT('Ctrl Pts',(37.395097264099,-9.23367082741551,-11.1152743215673));
#64219=CARTESIAN_POINT('Ctrl Pts',(37.4138419100591,-9.23598986623126,-11.1362993039434));
#64220=CARTESIAN_POINT('Ctrl Pts',(37.4463836399599,-9.23996493004659,-11.1715341173834));
#64221=CARTESIAN_POINT('Ctrl Pts',(37.4599952739039,-9.24161312674279,-11.1859119308212));
#64222=CARTESIAN_POINT('Ctrl Pts',(37.4862807812569,-9.24476992453289,-11.2129992527201));
#64223=CARTESIAN_POINT('Ctrl Pts',(37.4989225254221,-9.24627706924369,-11.2257382003176));
#64224=CARTESIAN_POINT('Ctrl Pts',(37.5289868941784,-9.24983650513509,-11.2553631954002));
#64225=CARTESIAN_POINT('Ctrl Pts',(37.5465244697505,-9.25189377398882,-11.272129121169));
#64226=CARTESIAN_POINT('Ctrl Pts',(37.611572031719,-9.25945832746464,-11.3324579566349));
#64227=CARTESIAN_POINT('Ctrl Pts',(37.6605697484187,-9.26503186677864,-11.3743676032643));
#64228=CARTESIAN_POINT('Ctrl Pts',(37.8563925814175,-9.28686185112621,-11.528684318001));
#64229=CARTESIAN_POINT('Ctrl Pts',(38.0142958621842,-9.30361025247569,-11.6259807459587));
#64230=CARTESIAN_POINT('Ctrl Pts',(38.2273307069811,-9.32460528217157,-11.7255224397344));
#64231=CARTESIAN_POINT('Ctrl Pts',(38.273575581874,-9.32907008738731,-11.7453880449763));
#64232=CARTESIAN_POINT('Ctrl Pts',(38.3517252761918,-9.33643034117287,-11.7760919049392));
#64233=CARTESIAN_POINT('Ctrl Pts',(38.3832949506832,-9.339354646512,-11.7877368321361));
#64234=CARTESIAN_POINT('Ctrl Pts',(38.4288006870547,-9.34349097261239,-11.8034456579335));
#64235=CARTESIAN_POINT('Ctrl Pts',(38.4425435453908,-9.34472999517254,-11.808051192705));
#64236=CARTESIAN_POINT('Ctrl Pts',(38.4666673642307,-9.34688625079088,-11.8158937986996));
#64237=CARTESIAN_POINT('Ctrl Pts',(38.4770298073106,-9.34780643222435,-11.8191850996326));
#64238=CARTESIAN_POINT('Ctrl Pts',(38.4999072029813,-9.34982454929236,-11.826280967285));
#64239=CARTESIAN_POINT('Ctrl Pts',(38.5124313225082,-9.35092070520118,-11.8300538720609));
#64240=CARTESIAN_POINT('Ctrl Pts',(38.5497434597968,-9.354162529741,-11.8409630181109));
#64241=CARTESIAN_POINT('Ctrl Pts',(38.5746172301577,-9.35629250864609,-11.8478032253696));
#64242=CARTESIAN_POINT('Ctrl Pts',(38.7032275648562,-9.36716964162247,-11.8809547502022));
#64243=CARTESIAN_POINT('Ctrl Pts',(38.8085395211198,-9.37562660110951,-11.9007252948594));
#64244=CARTESIAN_POINT('Ctrl Pts',(39.0086154395789,-9.39144839220423,-11.9246136583454));
#64245=CARTESIAN_POINT('Ctrl Pts',(39.102976178276,-9.39881074545997,-11.9302775006137));
#64246=CARTESIAN_POINT('Ctrl Pts',(39.2994307137867,-9.41430456385499,-11.9304878335481));
#64247=CARTESIAN_POINT('Ctrl Pts',(39.401327521681,-9.42243554854533,-11.9241083793512));
#64248=CARTESIAN_POINT('Ctrl Pts',(39.5326370092824,-9.43324446802153,-11.9074626451227));
#64249=CARTESIAN_POINT('Ctrl Pts',(39.5626951781424,-9.4357410269147,-11.9030722604324));
#64250=CARTESIAN_POINT('Ctrl Pts',(39.6126083336388,-9.43992875992945,-11.8948135167427));
#64251=CARTESIAN_POINT('Ctrl Pts',(39.6325127778823,-9.44160996348719,-11.8912616900869));
#64252=CARTESIAN_POINT('Ctrl Pts',(39.6716740346309,-9.44494122061502,-11.8837629978567));
#64253=CARTESIAN_POINT('Ctrl Pts',(39.690931945976,-9.44659071079216,-11.8798301532031));
#64254=CARTESIAN_POINT('Ctrl Pts',(39.7335216176593,-9.45026495468826,-11.8705873741876));
#64255=CARTESIAN_POINT('Ctrl Pts',(39.7568263786638,-9.45229312518751,-11.865164468919));
#64256=CARTESIAN_POINT('Ctrl Pts',(39.8390167320672,-9.45951127684508,-11.844741985784));
#64257=CARTESIAN_POINT('Ctrl Pts',(39.897405579748,-9.4647592603458,-11.82786111959));
#64258=CARTESIAN_POINT('Ctrl Pts',(40.1350838547624,-9.48664071325854,-11.7492777377663));
#64259=CARTESIAN_POINT('Ctrl Pts',(40.3073969641814,-9.5038163855517,-11.6686990442503));
#64260=CARTESIAN_POINT('Ctrl Pts',(40.5111444269179,-9.52522670498369,-11.5422457551159));
#64261=CARTESIAN_POINT('Ctrl Pts',(40.5530194624337,-9.52968752121862,-11.5144017163747));
#64262=CARTESIAN_POINT('Ctrl Pts',(40.6213940994178,-9.5370420179428,-11.4657787623434));
#64263=CARTESIAN_POINT('Ctrl Pts',(40.6483849584916,-9.53996450285203,-11.4457198492305));
#64264=CARTESIAN_POINT('Ctrl Pts',(40.686394315102,-9.54409874875633,-11.416215175119));
#64265=CARTESIAN_POINT('Ctrl Pts',(40.6977602814479,-9.54533747605842,-11.4072266257179));
#64266=CARTESIAN_POINT('Ctrl Pts',(40.7175111228534,-9.5474934127188,-11.391314854948));
#64267=CARTESIAN_POINT('Ctrl Pts',(40.7259312508121,-9.54841356736591,-11.3844367380608));
#64268=CARTESIAN_POINT('Ctrl Pts',(40.7443800029017,-9.55043186052524,-11.3691568495542));
#64269=CARTESIAN_POINT('Ctrl Pts',(40.7543870965754,-9.55152821692362,-11.3607300612231));
#64270=CARTESIAN_POINT('Ctrl Pts',(40.7833327016928,-9.55470582553626,-11.335949082968));
#64271=CARTESIAN_POINT('Ctrl Pts',(40.8020861754531,-9.55677263608426,-11.3193798542235));
#64272=CARTESIAN_POINT('Ctrl Pts',(40.9131619938549,-9.56908871980126,-11.2181111696449));
#64273=CARTESIAN_POINT('Ctrl Pts',(40.9990233367886,-9.57892995906961,-11.1265847931235));
#64274=CARTESIAN_POINT('Ctrl Pts',(41.154860317439,-9.5984664254528,-10.9320313635483));
#64275=CARTESIAN_POINT('Ctrl Pts',(41.2247506456372,-9.6081353811315,-10.8294531332533));
#64276=CARTESIAN_POINT('Ctrl Pts',(41.3083526330411,-9.62156262916336,-10.6837252597242));
#64277=CARTESIAN_POINT('Ctrl Pts',(41.3292262521221,-9.62511057235681,-10.6449063352985));
#64278=CARTESIAN_POINT('Ctrl Pts',(41.3651448517381,-9.63160982123405,-10.5734698693304));
#64279=CARTESIAN_POINT('Ctrl Pts',(41.3805481817686,-9.63454886559171,-10.5410465804955));
#64280=CARTESIAN_POINT('Ctrl Pts',(41.4039444249854,-9.63927464161083,-10.4888140115401));
#64281=CARTESIAN_POINT('Ctrl Pts',(41.4124093548565,-9.64104535649277,-10.4692209820813));
#64282=CARTESIAN_POINT('Ctrl Pts',(41.4280501107404,-9.64443843451144,-10.4316532632785));
#64283=CARTESIAN_POINT('Ctrl Pts',(41.4352719504081,-9.64605910535436,-10.4136994412727));
#64284=CARTESIAN_POINT('Ctrl Pts',(41.4514469436813,-9.64981856816897,-10.3720428121556));
#64285=CARTESIAN_POINT('Ctrl Pts',(41.4602436023868,-9.65196232957961,-10.3482822226648));
#64286=CARTESIAN_POINT('Ctrl Pts',(41.4878101753346,-9.65902191197186,-10.2700483023016));
#64287=CARTESIAN_POINT('Ctrl Pts',(41.5049970219363,-9.66398760806054,-10.2150434099349));
#64288=CARTESIAN_POINT('Ctrl Pts',(41.5426964490361,-9.67645043885916,-10.0771825211629));
#64289=CARTESIAN_POINT('Ctrl Pts',(41.5608044380972,-9.68400917891454,-9.99375545354374));
#64290=CARTESIAN_POINT('Ctrl Pts',(41.6021819969037,-9.70714973416176,-9.73826647628879));
#64291=CARTESIAN_POINT('Ctrl Pts',(41.6113085376177,-9.72291560244844,-9.56447720947855));
#64292=CARTESIAN_POINT('Ctrl Pts',(41.6002690151893,-9.74019628992671,-9.36630602395826));
#64293=CARTESIAN_POINT('Ctrl Pts',(41.5984942461151,-9.74235258560614,-9.34142270700628));
#64294=CARTESIAN_POINT('Ctrl Pts',(41.5952004462384,-9.74560936749034,-9.30355367512303));
#64295=CARTESIAN_POINT('Ctrl Pts',(41.5939622219895,-9.74672354689406,-9.29054625901079));
#64296=CARTESIAN_POINT('Ctrl Pts',(41.5914993518288,-9.74875441272202,-9.26673261381967));
#64297=CARTESIAN_POINT('Ctrl Pts',(41.5903073766744,-9.74967271215101,-9.25592408483536));
#64298=CARTESIAN_POINT('Ctrl Pts',(41.5873534570663,-9.75180723904353,-9.23070927653705));
#64299=CARTESIAN_POINT('Ctrl Pts',(41.5855343767785,-9.75302034946539,-9.21631030329359));
#64300=CARTESIAN_POINT('Ctrl Pts',(41.579050542142,-9.75703396569632,-9.1684733605748));
#64301=CARTESIAN_POINT('Ctrl Pts',(41.5738119010657,-9.75980569281046,-9.13511523659956));
#64302=CARTESIAN_POINT('Ctrl Pts',(41.5589770417625,-9.76666155625317,-9.05209689660818));
#64303=CARTESIAN_POINT('Ctrl Pts',(41.5485136017834,-9.7707107051752,-9.00260678332336));
#64304=CARTESIAN_POINT('Ctrl Pts',(41.5097811595432,-9.78365199973941,-8.84426028245814));
#64305=CARTESIAN_POINT('Ctrl Pts',(41.4754391271478,-9.79239790701268,-8.73704407953041));
#64306=CARTESIAN_POINT('Ctrl Pts',(41.3873680148016,-9.81103431007076,-8.51659284458178));
#64307=CARTESIAN_POINT('Ctrl Pts',(41.3320517945614,-9.82091914870271,-8.40436975377723));
#64308=CARTESIAN_POINT('Ctrl Pts',(41.2518987335009,-9.83372037203025,-8.2693751724872));
#64309=CARTESIAN_POINT('Ctrl Pts',(41.2349708596009,-9.83635380046167,-8.24212217063219));
#64310=CARTESIAN_POINT('Ctrl Pts',(41.206308016301,-9.84070727654865,-8.19797180341846));
#64311=CARTESIAN_POINT('Ctrl Pts',(41.1948919232908,-9.84241559597815,-8.18087134152878));
#64312=CARTESIAN_POINT('Ctrl Pts',(41.1721365950787,-9.84577306863913,-8.14771407594685));
#64313=CARTESIAN_POINT('Ctrl Pts',(41.1608169535158,-9.8474213876668,-8.13164574062517));
#64314=CARTESIAN_POINT('Ctrl Pts',(41.1332792310059,-9.85138126940241,-8.09355588032824));
#64315=CARTESIAN_POINT('Ctrl Pts',(41.116880376171,-9.85369958468706,-8.07166922431114));
#64316=CARTESIAN_POINT('Ctrl Pts',(41.0561061641709,-9.86215427564569,-7.99337555530586));
#64317=CARTESIAN_POINT('Ctrl Pts',(41.009589760205,-9.868372332876,-7.93868786556885));
#64318=CARTESIAN_POINT('Ctrl Pts',(40.8782804376939,-9.88529719817478,-7.79761386017638));
#64319=CARTESIAN_POINT('Ctrl Pts',(40.7893026268582,-9.89614207952887,-7.71541463097446));
#64320=CARTESIAN_POINT('Ctrl Pts',(40.6022005687849,-9.91760229513573,-7.5670490247789));
#64321=CARTESIAN_POINT('Ctrl Pts',(40.5046042990956,-9.9281867129792,-7.50070951495733));
#64322=CARTESIAN_POINT('Ctrl Pts',(40.3803034851884,-9.94068756863581,-7.4289572605237));
#64323=CARTESIAN_POINT('Ctrl Pts',(40.3578732834571,-9.94290648671804,-7.41648367261546));
#64324=CARTESIAN_POINT('Ctrl Pts',(40.3237382186541,-9.94622371919711,-7.39820998840165));
#64325=CARTESIAN_POINT('Ctrl Pts',(40.3121796531136,-9.94733684359566,-7.3921428127624));
#64326=CARTESIAN_POINT('Ctrl Pts',(40.2918721734471,-9.94927415600868,-7.38169324980225));
#64327=CARTESIAN_POINT('Ctrl Pts',(40.2831454158522,-9.95010075030636,-7.37726987603079));
#64328=CARTESIAN_POINT('Ctrl Pts',(40.2619787855003,-9.95209156764051,-7.36670287614843));
#64329=CARTESIAN_POINT('Ctrl Pts',(40.2495123686742,-9.95325250933276,-7.36061342810938));
#64330=CARTESIAN_POINT('Ctrl Pts',(40.2098973011235,-9.95690745735638,-7.34168550134192));
#64331=CARTESIAN_POINT('Ctrl Pts',(40.1825591575719,-9.95937926365402,-7.32924671021298));
#64332=CARTESIAN_POINT('Ctrl Pts',(40.115637547872,-9.96532623098157,-7.30029787650304));
#64333=CARTESIAN_POINT('Ctrl Pts',(40.0758306760907,-9.96877725176993,-7.28432759902196));
#64334=CARTESIAN_POINT('Ctrl Pts',(39.896715422316,-9.98401715607191,-7.21797124708811));
#64335=CARTESIAN_POINT('Ctrl Pts',(39.753352482418,-9.99546803917869,-7.17945097993236));
#64336=CARTESIAN_POINT('Ctrl Pts',(39.5047537849347,-10.0153450547201,-7.13673394022701));
#64337=CARTESIAN_POINT('Ctrl Pts',(39.4011346862367,-10.0236325808985,-7.12578556124515));
#64338=CARTESIAN_POINT('Ctrl Pts',(39.2659092406184,-10.0346756155144,-7.12031998038202));
#64339=CARTESIAN_POINT('Ctrl Pts',(39.2346563370499,-10.0372430319197,-7.11966659659776));
#64340=CARTESIAN_POINT('Ctrl Pts',(39.1830064712796,-10.0415164391197,-7.11959356833189));
#64341=CARTESIAN_POINT('Ctrl Pts',(39.162613087625,-10.0432115614634,-7.11982411310598));
#64342=CARTESIAN_POINT('Ctrl Pts',(39.1224746869288,-10.0465647348121,-7.120788466116));
#64343=CARTESIAN_POINT('Ctrl Pts',(39.1027308734574,-10.0482221595811,-7.12150630516188));
#64344=CARTESIAN_POINT('Ctrl Pts',(39.0550998320814,-10.052241306479,-7.12382589514023));
#64345=CARTESIAN_POINT('Ctrl Pts',(39.0272280011592,-10.0546103157471,-7.12567033619452));
#64346=CARTESIAN_POINT('Ctrl Pts',(38.9231233594639,-10.0635273776686,-7.13438281886791));
#64347=CARTESIAN_POINT('Ctrl Pts',(38.8472086339259,-10.0701695500691,-7.14440202120306));
#64348=CARTESIAN_POINT('Ctrl Pts',(38.635221156407,-10.089127689256,-7.1827420198866));
#64349=CARTESIAN_POINT('Ctrl Pts',(38.5009438561124,-10.1016359384576,-7.21925489642919));
#64350=CARTESIAN_POINT('Ctrl Pts',(38.2740423966006,-10.1233335438638,-7.30260639305684));
#64351=CARTESIAN_POINT('Ctrl Pts',(38.179862504395,-10.1325146704086,-7.34423048354423));
#64352=CARTESIAN_POINT('Ctrl Pts',(38.0705633385727,-10.1431913812666,-7.40117311910755));
#64353=CARTESIAN_POINT('Ctrl Pts',(38.0526192474599,-10.1449447697072,-7.41081332768427));
#64354=CARTESIAN_POINT('Ctrl Pts',(38.0243352861874,-10.1477070103589,-7.42647468893905));
#64355=CARTESIAN_POINT('Ctrl Pts',(38.0139146940803,-10.1487243672929,-7.43234673995433));
#64356=CARTESIAN_POINT('Ctrl Pts',(37.9938151877964,-10.1506854280061,-7.4438712787138));
#64357=CARTESIAN_POINT('Ctrl Pts',(37.9841313322134,-10.1516296311222,-7.4495140454382));
#64358=CARTESIAN_POINT('Ctrl Pts',(37.9600500222372,-10.153976928477,-7.46377257541043));
#64359=CARTESIAN_POINT('Ctrl Pts',(37.9457021943752,-10.1553748567722,-7.47247192292882));
#64360=CARTESIAN_POINT('Ctrl Pts',(37.8886789585346,-10.1609333343494,-7.50786743237705));
#64361=CARTESIAN_POINT('Ctrl Pts',(37.8467514365339,-10.1650263304812,-7.53575240065824));
#64362=CARTESIAN_POINT('Ctrl Pts',(37.630315254609,-10.1863664489294,-7.68971230660831));
#64363=CARTESIAN_POINT('Ctrl Pts',(37.472439723281,-10.2027647859929,-7.83747490581266));
#64364=CARTESIAN_POINT('Ctrl Pts',(37.2965956220547,-10.2249978555818,-8.05297620016607));
#64365=CARTESIAN_POINT('Ctrl Pts',(37.2587918025823,-10.2300738902301,-8.10320122378667));
#64366=CARTESIAN_POINT('Ctrl Pts',(37.2092736239237,-10.2371987324867,-8.17465109891706));
#64367=CARTESIAN_POINT('Ctrl Pts',(37.1958458164185,-10.2391840930391,-8.19466185397618));
#64368=CARTESIAN_POINT('Ctrl Pts',(37.1729669221607,-10.2426642930727,-8.22988974196906));
#64369=CARTESIAN_POINT('Ctrl Pts',(37.1633807808665,-10.2441540693138,-8.2450172660976));
#64370=CARTESIAN_POINT('Ctrl Pts',(37.1435335308567,-10.2473072885702,-8.27712493463417));
#64371=CARTESIAN_POINT('Ctrl Pts',(37.133311854702,-10.2489720165361,-8.29412771694485));
#64372=CARTESIAN_POINT('Ctrl Pts',(37.1089788465773,-10.2530373991254,-8.33576108067051));
#64373=CARTESIAN_POINT('Ctrl Pts',(37.095091320872,-10.2554457618124,-8.36051815146242));
#64374=CARTESIAN_POINT('Ctrl Pts',(37.0435060037021,-10.2647448590642,-8.45641751422547));
#64375=CARTESIAN_POINT('Ctrl Pts',(37.0089550976382,-10.2717407321173,-8.52918173924758));
#64376=CARTESIAN_POINT('Ctrl Pts',(36.9712314234316,-10.2804210444538,-8.62014259324087));
#64377=CARTESIAN_POINT('Ctrl Pts',(36.9645309575376,-10.2820103420603,-8.63682539037184));
#64378=CARTESIAN_POINT('Ctrl Pts',(36.9580196499262,-10.2836033739986,-8.65357756840738));
#64379=CARTESIAN_POINT('Origin',(39.2,8.05522481984854,-9.525));
#64380=CARTESIAN_POINT('',(36.9580196917093,-11.8220201063326,-8.65357746090844));
#64381=CARTESIAN_POINT('',(36.9580196848654,-11.5570870138823,-8.65357747851634));
#64382=CARTESIAN_POINT('',(36.958019684865,8.05522481984854,-8.65357747851728));
#64383=CARTESIAN_POINT('Ctrl Pts',(36.9580196917093,-11.8220201063326,-8.65357746090844));
#64384=CARTESIAN_POINT('Ctrl Pts',(37.0195222368154,-11.8071546836758,-8.49534481388361));
#64385=CARTESIAN_POINT('Ctrl Pts',(37.0976042895335,-11.7918150351386,-8.34406686960644));
#64386=CARTESIAN_POINT('Ctrl Pts',(37.2243281706615,-11.7711587714622,-8.15158924554521));
#64387=CARTESIAN_POINT('Ctrl Pts',(37.2596109124396,-11.7657471775599,-8.10217621399113));
#64388=CARTESIAN_POINT('Ctrl Pts',(37.3045735023623,-11.7592799084008,-8.04399494539265));
#64389=CARTESIAN_POINT('Ctrl Pts',(37.3125007825056,-11.7581547439394,-8.03390499971234));
#64390=CARTESIAN_POINT('Ctrl Pts',(37.3362178562845,-11.7548336594147,-8.00420984006869));
#64391=CARTESIAN_POINT('Ctrl Pts',(37.3522358010931,-11.7526488305522,-7.9847876118182));
#64392=CARTESIAN_POINT('Ctrl Pts',(37.3688690972522,-11.7504410356872,-7.96525233010145));
#64393=CARTESIAN_POINT('Ctrl Pts',(37.3691817017606,-11.7503995641396,-7.96488540946997));
#64394=CARTESIAN_POINT('Ctrl Pts',(37.3697839232714,-11.7503197121562,-7.96417898014284));
#64395=CARTESIAN_POINT('Ctrl Pts',(37.3700735244568,-11.75028133074,-7.96383945807921));
#64396=CARTESIAN_POINT('Ctrl Pts',(37.3706319534729,-11.7502073566368,-7.96318513705621));
#64397=CARTESIAN_POINT('Ctrl Pts',(37.3709007680591,-11.7501717631295,-7.96287032693173));
#64398=CARTESIAN_POINT('Ctrl Pts',(37.3714195888865,-11.750103097176,-7.96226305075639));
#64399=CARTESIAN_POINT('Ctrl Pts',(37.3716695840387,-11.7500700240347,-7.96197057528958));
#64400=CARTESIAN_POINT('Ctrl Pts',(37.3721525125285,-11.7500061614658,-7.96140585978445));
#64401=CARTESIAN_POINT('Ctrl Pts',(37.3723854364694,-11.749975371457,-7.96113361186337));
#64402=CARTESIAN_POINT('Ctrl Pts',(37.3819792837052,-11.7487076597144,-7.94992512951868));
#64403=CARTESIAN_POINT('Ctrl Pts',(37.3914385004635,-11.747476956279,-7.93907266648057));
#64404=CARTESIAN_POINT('Ctrl Pts',(37.4081823772785,-11.7453327514335,-7.92020724389243));
#64405=CARTESIAN_POINT('Ctrl Pts',(37.4154244249836,-11.7444163577425,-7.91215772084796));
#64406=CARTESIAN_POINT('Ctrl Pts',(37.431526990034,-11.7424029053641,-7.89450101638728));
#64407=CARTESIAN_POINT('Ctrl Pts',(37.4404117415958,-11.7413076556525,-7.88491679848045));
#64408=CARTESIAN_POINT('Ctrl Pts',(37.4670098820244,-11.7380732117081,-7.85668963548916));
#64409=CARTESIAN_POINT('Ctrl Pts',(37.4849453534326,-11.7359495871312,-7.83825700165438));
#64410=CARTESIAN_POINT('Ctrl Pts',(37.5847524841808,-11.7244162263516,-7.73892169664024));
#64411=CARTESIAN_POINT('Ctrl Pts',(37.6720654790745,-11.7153454391813,-7.66367683318644));
#64412=CARTESIAN_POINT('Ctrl Pts',(37.8616071265024,-11.6968157202338,-7.5226960349588));
#64413=CARTESIAN_POINT('Ctrl Pts',(37.9640843881882,-11.6873845172794,-7.45786979289354));
#64414=CARTESIAN_POINT('Ctrl Pts',(38.1362960797734,-11.6718615008937,-7.36633037895077));
#64415=CARTESIAN_POINT('Ctrl Pts',(38.2031474330634,-11.6659101500289,-7.33465674946773));
#64416=CARTESIAN_POINT('Ctrl Pts',(38.296862276295,-11.6575912792807,-7.29543494156573));
#64417=CARTESIAN_POINT('Ctrl Pts',(38.3225602408113,-11.6553127294249,-7.2851970088896));
#64418=CARTESIAN_POINT('Ctrl Pts',(38.3668955358238,-11.651382461485,-7.26841412360326));
#64419=CARTESIAN_POINT('Ctrl Pts',(38.3854478718677,-11.649738062565,-7.26165123155069));
#64420=CARTESIAN_POINT('Ctrl Pts',(38.4234660880219,-11.64636748542,-7.24832039560665));
#64421=CARTESIAN_POINT('Ctrl Pts',(38.4429369975882,-11.6446408279038,-7.24177191415941));
#64422=CARTESIAN_POINT('Ctrl Pts',(38.4927768647658,-11.6402185146263,-7.22571729865245));
#64423=CARTESIAN_POINT('Ctrl Pts',(38.523253968771,-11.6375118177066,-7.21656327676573));
#64424=CARTESIAN_POINT('Ctrl Pts',(38.664175965299,-11.6249782284927,-7.17726674543057));
#64425=CARTESIAN_POINT('Ctrl Pts',(38.7764852118321,-11.6149282994709,-7.15443343461381));
#64426=CARTESIAN_POINT('Ctrl Pts',(39.026615993977,-11.5924443976172,-7.12192345211543));
#64427=CARTESIAN_POINT('Ctrl Pts',(39.1645252726663,-11.5799772490267,-7.11593805667749));
#64428=CARTESIAN_POINT('Ctrl Pts',(39.3633490766828,-11.5622878086934,-7.12439224120074));
#64429=CARTESIAN_POINT('Ctrl Pts',(39.4243966546015,-11.5568986809718,-7.12932717255241));
#64430=CARTESIAN_POINT('Ctrl Pts',(39.5029757819074,-11.5500646614959,-7.13871014658836));
#64431=CARTESIAN_POINT('Ctrl Pts',(39.5207325836487,-11.548527223667,-7.14103182541052));
#64432=CARTESIAN_POINT('Ctrl Pts',(39.5498109836354,-11.5460224885509,-7.14516458398484));
#64433=CARTESIAN_POINT('Ctrl Pts',(39.5611481033032,-11.5450491832041,-7.14685862529736));
#64434=CARTESIAN_POINT('Ctrl Pts',(39.5826078660378,-11.5432135096309,-7.15022224146873));
#64435=CARTESIAN_POINT('Ctrl Pts',(39.5927326732926,-11.5423502429387,-7.15187563723592));
#64436=CARTESIAN_POINT('Ctrl Pts',(39.620206445833,-11.5400146197291,-7.15654279369386));
#64437=CARTESIAN_POINT('Ctrl Pts',(39.637533886892,-11.5385490123967,-7.15968244220655));
#64438=CARTESIAN_POINT('Ctrl Pts',(39.7074110032163,-11.5326628278137,-7.17313803008069));
#64439=CARTESIAN_POINT('Ctrl Pts',(39.7596486613197,-11.5283180062888,-7.18501811655564));
#64440=CARTESIAN_POINT('Ctrl Pts',(39.9533989118675,-11.5122595782045,-7.23594252906467));
#64441=CARTESIAN_POINT('Ctrl Pts',(40.0916442762226,-11.5009005542583,-7.28616743490815));
#64442=CARTESIAN_POINT('Ctrl Pts',(40.329224786239,-11.4802516527406,-7.39800380030746));
#64443=CARTESIAN_POINT('Ctrl Pts',(40.4302806875294,-11.4710616282955,-7.45481521743878));
#64444=CARTESIAN_POINT('Ctrl Pts',(40.5529540547388,-11.4590608071579,-7.53594289813821));
#64445=CARTESIAN_POINT('Ctrl Pts',(40.5787231066101,-11.4564896875235,-7.55371736125102));
#64446=CARTESIAN_POINT('Ctrl Pts',(40.620710760708,-11.4522109894795,-7.58390480255449));
#64447=CARTESIAN_POINT('Ctrl Pts',(40.6371318001931,-11.4505143131566,-7.59603090577427));
#64448=CARTESIAN_POINT('Ctrl Pts',(40.6689673515638,-11.4471774759012,-7.62017198771938));
#64449=CARTESIAN_POINT('Ctrl Pts',(40.6843937191474,-11.4455381153245,-7.63216876748468));
#64450=CARTESIAN_POINT('Ctrl Pts',(40.7179837501729,-11.4419175238457,-7.65895422361889));
#64451=CARTESIAN_POINT('Ctrl Pts',(40.7360807990141,-11.4399332453863,-7.67382275271356));
#64452=CARTESIAN_POINT('Ctrl Pts',(40.7985070376105,-11.4329671290314,-7.72665782777859));
#64453=CARTESIAN_POINT('Ctrl Pts',(40.841665473089,-11.4279320845181,-7.76596828980467));
#64454=CARTESIAN_POINT('Ctrl Pts',(41.0421755785805,-11.403430760465,-7.96241191243846));
#64455=CARTESIAN_POINT('Ctrl Pts',(41.1786505420858,-11.3831518322833,-8.13928504758494));
#64456=CARTESIAN_POINT('Ctrl Pts',(41.3137051728022,-11.3590453381884,-8.37582095550486));
#64457=CARTESIAN_POINT('Ctrl Pts',(41.3371797435689,-11.3546548590138,-8.42009015976991));
#64458=CARTESIAN_POINT('Ctrl Pts',(41.3666384748711,-11.3488898535286,-8.4801022567753));
#64459=CARTESIAN_POINT('Ctrl Pts',(41.3738633161429,-11.347453247059,-8.49521754417655));
#64460=CARTESIAN_POINT('Ctrl Pts',(41.3856551655224,-11.3450711785047,-8.52056486679085));
#64461=CARTESIAN_POINT('Ctrl Pts',(41.3903095596056,-11.3441207238461,-8.53075531402184));
#64462=CARTESIAN_POINT('Ctrl Pts',(41.3997866770966,-11.3421644541308,-8.55189433930267));
#64463=CARTESIAN_POINT('Ctrl Pts',(41.4045992022457,-11.3411592316009,-8.56284698290802));
#64464=CARTESIAN_POINT('Ctrl Pts',(41.4173950150876,-11.3384527280887,-8.59256862531486));
#64465=CARTESIAN_POINT('Ctrl Pts',(41.4252218816092,-11.3367603257791,-8.61140458410712));
#64466=CARTESIAN_POINT('Ctrl Pts',(41.4735975747839,-11.3260429539613,-8.73213594129483));
#64467=CARTESIAN_POINT('Ctrl Pts',(41.5073837384875,-11.3173526131309,-8.83661993110928));
#64468=CARTESIAN_POINT('Ctrl Pts',(41.5553543782027,-11.3017676870822,-9.02901063007428));
#64469=CARTESIAN_POINT('Ctrl Pts',(41.5720209596351,-11.2948618796711,-9.11607906777508));
#64470=CARTESIAN_POINT('Ctrl Pts',(41.5989223045068,-11.2790101483759,-9.31577503321823));
#64471=CARTESIAN_POINT('Ctrl Pts',(41.606096997276,-11.2700413059539,-9.42858939908781));
#64472=CARTESIAN_POINT('Ctrl Pts',(41.6051103870479,-11.2582897474402,-9.5725917650785));
#64473=CARTESIAN_POINT('Ctrl Pts',(41.6042936235563,-11.2557340979116,-9.60369525065076));
#64474=CARTESIAN_POINT('Ctrl Pts',(41.6019448565877,-11.2514756369124,-9.65510865733092));
#64475=CARTESIAN_POINT('Ctrl Pts',(41.6007577412977,-11.2497835576421,-9.67543128407569));
#64476=CARTESIAN_POINT('Ctrl Pts',(41.5979261762536,-11.2464518162339,-9.71522265886003));
#64477=CARTESIAN_POINT('Ctrl Pts',(41.5963021745664,-11.2448129153817,-9.73469131303294));
#64478=CARTESIAN_POINT('Ctrl Pts',(41.5917890010068,-11.2408201578185,-9.78185309414413));
#64479=CARTESIAN_POINT('Ctrl Pts',(41.588655846342,-11.2384589336017,-9.80951932264566));
#64480=CARTESIAN_POINT('Ctrl Pts',(41.5759554407952,-11.2301053614676,-9.90656743512703));
#64481=CARTESIAN_POINT('Ctrl Pts',(41.5638400520901,-11.2240364975671,-9.97557306420601));
#64482=CARTESIAN_POINT('Ctrl Pts',(41.5047640422709,-11.1999937477026,-10.2429497519612));
#64483=CARTESIAN_POINT('Ctrl Pts',(41.4356905819047,-11.1814334847706,-10.4355268394577));
#64484=CARTESIAN_POINT('Ctrl Pts',(41.3196780700855,-11.1588007556919,-10.663199214008));
#64485=CARTESIAN_POINT('Ctrl Pts',(41.2946908038853,-11.1542602388255,-10.7085556906512));
#64486=CARTESIAN_POINT('Ctrl Pts',(41.259613007265,-11.1483339703858,-10.7676318165868));
#64487=CARTESIAN_POINT('Ctrl Pts',(41.2508154771883,-11.1468817937277,-10.7820980472147));
#64488=CARTESIAN_POINT('Ctrl Pts',(41.2359282272724,-11.1444816548536,-10.8060056057672));
#64489=CARTESIAN_POINT('Ctrl Pts',(41.2299239398314,-11.143528533282,-10.8154991012039));
#64490=CARTESIAN_POINT('Ctrl Pts',(41.217415886543,-11.1415738445939,-10.8349725034995));
#64491=CARTESIAN_POINT('Ctrl Pts',(41.2109041376472,-11.1405728049616,-10.84494673657));
#64492=CARTESIAN_POINT('Ctrl Pts',(41.1931917250614,-11.1378927764832,-10.871642012258));
#64493=CARTESIAN_POINT('Ctrl Pts',(41.1818545231596,-11.1362223535868,-10.8882720538359));
#64494=CARTESIAN_POINT('Ctrl Pts',(41.1174879701893,-11.1269725938104,-10.9801881435499));
#64495=CARTESIAN_POINT('Ctrl Pts',(41.0603708219234,-11.1196261435177,-11.0525332709065));
#64496=CARTESIAN_POINT('Ctrl Pts',(40.9014456362142,-11.1007300890364,-11.2316476080352));
#64497=CARTESIAN_POINT('Ctrl Pts',(40.7937363377978,-11.089327744614,-11.3326415028221));
#64498=CARTESIAN_POINT('Ctrl Pts',(40.6153230183019,-11.071366618117,-11.4715134424039));
#64499=CARTESIAN_POINT('Ctrl Pts',(40.5508517925976,-11.0650399920595,-11.5167959093007));
#64500=CARTESIAN_POINT('Ctrl Pts',(40.4604401461102,-11.0562893734585,-11.5738871800599));
#64501=CARTESIAN_POINT('Ctrl Pts',(40.4363364277138,-11.053967832134,-11.58852129645));
#64502=CARTESIAN_POINT('Ctrl Pts',(40.3948678220516,-11.0499890690345,-11.6127108014208));
#64503=CARTESIAN_POINT('Ctrl Pts',(40.3776314688782,-11.0483396961033,-11.6224817226459));
#64504=CARTESIAN_POINT('Ctrl Pts',(40.3445484759961,-11.0451810084547,-11.6406994421413));
#64505=CARTESIAN_POINT('Ctrl Pts',(40.3287240207539,-11.0436731548696,-11.649183935298));
#64506=CARTESIAN_POINT('Ctrl Pts',(40.2871589904224,-11.0397193906007,-11.6708739931416));
#64507=CARTESIAN_POINT('Ctrl Pts',(40.2612733555155,-11.0372637940236,-11.6837933140816));
#64508=CARTESIAN_POINT('Ctrl Pts',(40.163583322238,-11.02801680778,-11.7303680519948));
#64509=CARTESIAN_POINT('Ctrl Pts',(40.0903699814951,-11.0211247214396,-11.7609292011787));
#64510=CARTESIAN_POINT('Ctrl Pts',(39.8361762735025,-10.9973065390112,-11.8525710098921));
#64511=CARTESIAN_POINT('Ctrl Pts',(39.649515633545,-10.9799374337163,-11.895702646915));
#64512=CARTESIAN_POINT('Ctrl Pts',(39.4076359026872,-10.9583827891825,-11.9219744241546));
#64513=CARTESIAN_POINT('Ctrl Pts',(39.3553625440727,-10.9537852750119,-11.9259295356887));
#64514=CARTESIAN_POINT('Ctrl Pts',(39.2859992675856,-10.9477963348357,-11.9289023516445));
#64515=CARTESIAN_POINT('Ctrl Pts',(39.2689937542405,-10.946336942828,-11.9294505200274));
#64516=CARTESIAN_POINT('Ctrl Pts',(39.2407277277163,-10.943927423039,-11.9300615251131));
#64517=CARTESIAN_POINT('Ctrl Pts',(39.229470296981,-10.9429720734464,-11.9302258130321));
#64518=CARTESIAN_POINT('Ctrl Pts',(39.2078022050263,-10.9411419438774,-11.9303898710122));
#64519=CARTESIAN_POINT('Ctrl Pts',(39.1973921092614,-10.9402665093473,-11.930401113665));
#64520=CARTESIAN_POINT('Ctrl Pts',(39.1685312025315,-10.9378492171314,-11.9302449147077));
#64521=CARTESIAN_POINT('Ctrl Pts',(39.1500813325842,-10.9363149756565,-11.9299327590745));
#64522=CARTESIAN_POINT('Ctrl Pts',(39.0692034001497,-10.9296304803071,-11.9276331756873));
#64523=CARTESIAN_POINT('Ctrl Pts',(39.006856311245,-10.9245847574778,-11.9234268236468));
#64524=CARTESIAN_POINT('Ctrl Pts',(38.7915986559681,-10.9073130463647,-11.9004535848222));
#64525=CARTESIAN_POINT('Ctrl Pts',(38.6403769544948,-10.8954217297262,-11.8694399865349));
#64526=CARTESIAN_POINT('Ctrl Pts',(38.3972836927085,-10.8753551150544,-11.7947045784404));
#64527=CARTESIAN_POINT('Ctrl Pts',(38.3033645998504,-10.8673559082107,-11.759267906401));
#64528=CARTESIAN_POINT('Ctrl Pts',(38.1843612714501,-10.8566956605179,-11.7056526227532));
#64529=CARTESIAN_POINT('Ctrl Pts',(38.1570210968949,-10.8542093514122,-11.6927090972907));
#64530=CARTESIAN_POINT('Ctrl Pts',(38.1118448482176,-10.8500336717585,-11.6702690363627));
#64531=CARTESIAN_POINT('Ctrl Pts',(38.0938707171895,-10.8483541407158,-11.6610568415827));
#64532=CARTESIAN_POINT('Ctrl Pts',(38.0586145450799,-10.8450222671022,-11.6424228569449));
#64533=CARTESIAN_POINT('Ctrl Pts',(38.0413279078921,-10.8433704514099,-11.6330131037533));
#64534=CARTESIAN_POINT('Ctrl Pts',(38.0032061280026,-10.8396860013776,-11.6116514463966));
#64535=CARTESIAN_POINT('Ctrl Pts',(37.9824309105439,-10.8376498872258,-11.5995976123797));
#64536=CARTESIAN_POINT('Ctrl Pts',(37.9089609177217,-10.8303452151844,-11.555486458818));
#64537=CARTESIAN_POINT('Ctrl Pts',(37.8573275130777,-10.8250166660665,-11.52171888788));
#64538=CARTESIAN_POINT('Ctrl Pts',(37.6302323351314,-10.8006576014357,-11.3604082176992));
#64539=CARTESIAN_POINT('Ctrl Pts',(37.4712198005621,-10.7808839185243,-11.2114720860351));
#64540=CARTESIAN_POINT('Ctrl Pts',(37.3026515652698,-10.7572476118606,-11.0043391704961));
#64541=CARTESIAN_POINT('Ctrl Pts',(37.2721740260759,-10.752845264629,-10.9643969091811));
#64542=CARTESIAN_POINT('Ctrl Pts',(37.2332182424327,-10.7470674178816,-10.9098839657391));
#64543=CARTESIAN_POINT('Ctrl Pts',(37.2236120549459,-10.745629521514,-10.8961399710529));
#64544=CARTESIAN_POINT('Ctrl Pts',(37.2078263716079,-10.7432458307098,-10.8730440519958));
#64545=CARTESIAN_POINT('Ctrl Pts',(37.2015672474306,-10.7422950327158,-10.8637475820482));
#64546=CARTESIAN_POINT('Ctrl Pts',(37.1887591683886,-10.7403380799546,-10.8444341465707));
#64547=CARTESIAN_POINT('Ctrl Pts',(37.1822196160994,-10.7393325167499,-10.8344115057756));
#64548=CARTESIAN_POINT('Ctrl Pts',(37.1647394034661,-10.7366259473597,-10.8071790411262));
#64549=CARTESIAN_POINT('Ctrl Pts',(37.1539420023191,-10.7349338057897,-10.7898776795524));
#64550=CARTESIAN_POINT('Ctrl Pts',(37.0874577471661,-10.7243699231704,-10.6802661583647));
#64551=CARTESIAN_POINT('Ctrl Pts',(37.0378009606188,-10.7158208738665,-10.5844230280174));
#64552=CARTESIAN_POINT('Ctrl Pts',(36.9407480131908,-10.6967109946233,-10.3616073506474));
#64553=CARTESIAN_POINT('Ctrl Pts',(36.8973065566811,-10.6862163689718,-10.2333310587889));
#64554=CARTESIAN_POINT('Ctrl Pts',(36.8525937228548,-10.6713925919154,-10.0524047612069));
#64555=CARTESIAN_POINT('Ctrl Pts',(36.8419050820114,-10.6672909083432,-10.0023465784628));
#64556=CARTESIAN_POINT('Ctrl Pts',(36.8256923288185,-10.6598905226161,-9.91246479852545));
#64557=CARTESIAN_POINT('Ctrl Pts',(36.8195545181075,-10.6566102317367,-9.87277122553581));
#64558=CARTESIAN_POINT('Ctrl Pts',(36.8115700151325,-10.6514683029081,-9.81091688774761));
#64559=CARTESIAN_POINT('Ctrl Pts',(36.8090318658065,-10.649628100642,-9.78885142111596));
#64560=CARTESIAN_POINT('Ctrl Pts',(36.8048686574815,-10.6461781952384,-9.74763861086654));
#64561=CARTESIAN_POINT('Ctrl Pts',(36.8031667693101,-10.6445710138068,-9.72850065783374));
#64562=CARTESIAN_POINT('Ctrl Pts',(36.7998617855699,-10.6409473874819,-9.68550321698142));
#64563=CARTESIAN_POINT('Ctrl Pts',(36.7983848922809,-10.6389272034291,-9.66163643975376));
#64564=CARTESIAN_POINT('Ctrl Pts',(36.7954814940953,-10.6336653214152,-9.59976554608665));
#64565=CARTESIAN_POINT('Ctrl Pts',(36.7946001050408,-10.6304073900687,-9.56174407021846));
#64566=CARTESIAN_POINT('Ctrl Pts',(36.7947067641619,-10.6130956163816,-9.36132361716306));
#64567=CARTESIAN_POINT('Ctrl Pts',(36.8112388358979,-10.5985869402844,-9.19938264598348));
#64568=CARTESIAN_POINT('Ctrl Pts',(36.8679872736717,-10.5732732082353,-8.92349507448723));
#64569=CARTESIAN_POINT('Ctrl Pts',(36.9006948735118,-10.5625511509026,-8.80855498415655));
#64570=CARTESIAN_POINT('Ctrl Pts',(36.9470719552065,-10.5508228197936,-8.68214641616852));
#64571=CARTESIAN_POINT('Ctrl Pts',(36.9524776905052,-10.5494961679529,-8.66783582272116));
#64572=CARTESIAN_POINT('Ctrl Pts',(36.958019684939,-10.5481760837449,-8.65357747832709));
#64573=CARTESIAN_POINT('Ctrl Pts',(36.9580196499262,-10.2836033739986,-8.65357756840738));
#64574=CARTESIAN_POINT('Ctrl Pts',(36.9084867414416,-10.2957219083884,-8.78101496670975));
#64575=CARTESIAN_POINT('Ctrl Pts',(36.8699012361887,-10.3080770742071,-8.91246580418143));
#64576=CARTESIAN_POINT('Ctrl Pts',(36.8261576094698,-10.3277553664387,-9.12796664229451));
#64577=CARTESIAN_POINT('Ctrl Pts',(36.8138532195428,-10.335133254408,-9.2102459589881));
#64578=CARTESIAN_POINT('Ctrl Pts',(36.8039287097411,-10.3440412841354,-9.31266661688286));
#64579=CARTESIAN_POINT('Ctrl Pts',(36.8022657951861,-10.3457406691889,-9.33235043669171));
#64580=CARTESIAN_POINT('Ctrl Pts',(36.7999950071111,-10.3484379371115,-9.36385133724607));
#64581=CARTESIAN_POINT('Ctrl Pts',(36.7992315479296,-10.349443683289,-9.37565571453295));
#64582=CARTESIAN_POINT('Ctrl Pts',(36.797909668938,-10.3513998356577,-9.39873663268032));
#64583=CARTESIAN_POINT('Ctrl Pts',(36.7973435069549,-10.3523505877009,-9.41001224593019));
#64584=CARTESIAN_POINT('Ctrl Pts',(36.7961150936825,-10.3547393658493,-9.43847720714928));
#64585=CARTESIAN_POINT('Ctrl Pts',(36.7955577835264,-10.3561718214584,-9.45567095255194));
#64586=CARTESIAN_POINT('Ctrl Pts',(36.794009009724,-10.3620865381518,-9.52711755760656));
#64587=CARTESIAN_POINT('Ctrl Pts',(36.7946688482976,-10.3664897904078,-9.58139523367149));
#64588=CARTESIAN_POINT('Ctrl Pts',(36.8028873106598,-10.3808162537491,-9.75992956150876));
#64589=CARTESIAN_POINT('Ctrl Pts',(36.8182501684603,-10.3904986983501,-9.88362769426369));
#64590=CARTESIAN_POINT('Ctrl Pts',(36.8701406366574,-10.4108615187152,-10.1381061228902));
#64591=CARTESIAN_POINT('Ctrl Pts',(36.9082857402076,-10.4215245235867,-10.2680892633524));
#64592=CARTESIAN_POINT('Ctrl Pts',(36.969015255277,-10.4352192103108,-10.4247995537014));
#64593=CARTESIAN_POINT('Ctrl Pts',(36.9815116166847,-10.4379144720478,-10.4551834506818));
#64594=CARTESIAN_POINT('Ctrl Pts',(37.0028968720256,-10.4423430987306,-10.5042956751161));
#64595=CARTESIAN_POINT('Ctrl Pts',(37.0114128592375,-10.4440639088899,-10.5231825713195));
#64596=CARTESIAN_POINT('Ctrl Pts',(37.0284468290345,-10.4474267113169,-10.5596945883188));
#64597=CARTESIAN_POINT('Ctrl Pts',(37.0369381201021,-10.4490676831488,-10.5773304238024));
#64598=CARTESIAN_POINT('Ctrl Pts',(37.0575892724685,-10.4529781452075,-10.6189152486571));
#64599=CARTESIAN_POINT('Ctrl Pts',(37.0699366337988,-10.455253946288,-10.6427675191933));
#64600=CARTESIAN_POINT('Ctrl Pts',(37.1149603467756,-10.4633433974374,-10.7262868891846));
#64601=CARTESIAN_POINT('Ctrl Pts',(37.1497624147167,-10.469229585653,-10.7847636541255));
#64602=CARTESIAN_POINT('Ctrl Pts',(37.2540020574395,-10.4859235625733,-10.9441303991183));
#64603=CARTESIAN_POINT('Ctrl Pts',(37.3287281318592,-10.4968876624622,-11.0413027638943));
#64604=CARTESIAN_POINT('Ctrl Pts',(37.4918609597442,-10.5188273743655,-11.222920277095));
#64605=CARTESIAN_POINT('Ctrl Pts',(37.5799744628514,-10.5297706570977,-11.3071884702292));
#64606=CARTESIAN_POINT('Ctrl Pts',(37.6935144391638,-10.5425606736771,-11.4003626414968));
#64607=CARTESIAN_POINT('Ctrl Pts',(37.7131797625734,-10.5447322115027,-11.4159916748559));
#64608=CARTESIAN_POINT('Ctrl Pts',(37.7434706469762,-10.5480071633345,-11.4393006132146));
#64609=CARTESIAN_POINT('Ctrl Pts',(37.7539193318076,-10.5491244918161,-11.447205847394));
#64610=CARTESIAN_POINT('Ctrl Pts',(37.7731542373874,-10.5511581700227,-11.4615129147173));
#64611=CARTESIAN_POINT('Ctrl Pts',(37.7819196790074,-10.5520761678913,-11.4679408928559));
#64612=CARTESIAN_POINT('Ctrl Pts',(37.802448949461,-10.5542062207974,-11.4827827139772));
#64613=CARTESIAN_POINT('Ctrl Pts',(37.814245527631,-10.5554152046499,-11.4911502152087));
#64614=CARTESIAN_POINT('Ctrl Pts',(37.8535776650137,-10.5593995323423,-11.5185192578973));
#64615=CARTESIAN_POINT('Ctrl Pts',(37.8814357331471,-10.5621466670681,-11.5370538623808));
#64616=CARTESIAN_POINT('Ctrl Pts',(37.9517972183045,-10.5689261483888,-11.5817775940225));
#64617=CARTESIAN_POINT('Ctrl Pts',(37.994747418289,-10.5729245033001,-11.6072370728988));
#64618=CARTESIAN_POINT('Ctrl Pts',(38.2080392924415,-10.5922685059288,-11.7248563759732));
#64619=CARTESIAN_POINT('Ctrl Pts',(38.3882851470639,-10.6071229143317,-11.797548351));
#64620=CARTESIAN_POINT('Ctrl Pts',(38.6315881828157,-10.6273047431252,-11.8629817157395));
#64621=CARTESIAN_POINT('Ctrl Pts',(38.6884036098759,-10.6320209547872,-11.8760675443641));
#64622=CARTESIAN_POINT('Ctrl Pts',(38.7687798267058,-10.6387336432129,-11.891528608507));
#64623=CARTESIAN_POINT('Ctrl Pts',(38.7919889046969,-10.640676582182,-11.8956402846765));
#64624=CARTESIAN_POINT('Ctrl Pts',(38.8345699440263,-10.6442520436382,-11.9025400579212));
#64625=CARTESIAN_POINT('Ctrl Pts',(38.8539229053777,-10.6458811369632,-11.9054340885575));
#64626=CARTESIAN_POINT('Ctrl Pts',(38.8934589456214,-10.6492187323971,-11.9108539771598));
#64627=CARTESIAN_POINT('Ctrl Pts',(38.9136430033449,-10.6509276935298,-11.9133605746287));
#64628=CARTESIAN_POINT('Ctrl Pts',(38.9646467842253,-10.6552602751684,-11.9190387727834));
#64629=CARTESIAN_POINT('Ctrl Pts',(38.9954995406788,-10.6578941303377,-11.921871325597));
#64630=CARTESIAN_POINT('Ctrl Pts',(39.1367650399096,-10.6700198009259,-11.9320935161316));
#64631=CARTESIAN_POINT('Ctrl Pts',(39.2475338716148,-10.6797207201588,-11.9324531828017));
#64632=CARTESIAN_POINT('Ctrl Pts',(39.445286252741,-10.6973684454969,-11.9194422924778));
#64633=CARTESIAN_POINT('Ctrl Pts',(39.5322723603936,-10.7052441766121,-11.9089280761907));
#64634=CARTESIAN_POINT('Ctrl Pts',(39.7211448505958,-10.7224742174449,-11.8755591855773));
#64635=CARTESIAN_POINT('Ctrl Pts',(39.8225262277717,-10.731808167891,-11.8507657428578));
#64636=CARTESIAN_POINT('Ctrl Pts',(39.9464372578176,-10.743122127395,-11.8117753046892));
#64637=CARTESIAN_POINT('Ctrl Pts',(39.9707630614893,-10.7453382799188,-11.8036913650251));
#64638=CARTESIAN_POINT('Ctrl Pts',(40.0072707178494,-10.7486522588533,-11.7909075814864));
#64639=CARTESIAN_POINT('Ctrl Pts',(40.0195501544948,-10.7497648534031,-11.7864952461642));
#64640=CARTESIAN_POINT('Ctrl Pts',(40.0419994857473,-10.7517943590197,-11.7782217200871));
#64641=CARTESIAN_POINT('Ctrl Pts',(40.0521795753056,-10.7527128648811,-11.7743913033801));
#64642=CARTESIAN_POINT('Ctrl Pts',(40.0759072994248,-10.7548498428737,-11.7652791681621));
#64643=CARTESIAN_POINT('Ctrl Pts',(40.0894335555238,-10.756065173785,-11.7599434739442));
#64644=CARTESIAN_POINT('Ctrl Pts',(40.1343532266901,-10.7600943241237,-11.7417516196986));
#64645=CARTESIAN_POINT('Ctrl Pts',(40.1655248383629,-10.7628790641116,-11.7283533149218));
#64646=CARTESIAN_POINT('Ctrl Pts',(40.2427461466651,-10.7697754406884,-11.6932079616155));
#64647=CARTESIAN_POINT('Ctrl Pts',(40.2884097048502,-10.7738515595481,-11.6706491791863));
#64648=CARTESIAN_POINT('Ctrl Pts',(40.4360521967061,-10.7871373044353,-11.5917829224825));
#64649=CARTESIAN_POINT('Ctrl Pts',(40.5346613037689,-10.7961893457013,-11.5295194305981));
#64650=CARTESIAN_POINT('Ctrl Pts',(40.7253424041157,-10.8148061066151,-11.3887885875116));
#64651=CARTESIAN_POINT('Ctrl Pts',(40.8167812176551,-10.8243531609113,-11.3100460841137));
#64652=CARTESIAN_POINT('Ctrl Pts',(40.92452973377,-10.8367867671987,-11.2021622242884));
#64653=CARTESIAN_POINT('Ctrl Pts',(40.9466769911781,-10.8394124476964,-11.1790844065265));
#64654=CARTESIAN_POINT('Ctrl Pts',(40.9822815989904,-10.8437565776157,-11.1404712057185));
#64655=CARTESIAN_POINT('Ctrl Pts',(40.9960121827993,-10.8454634022954,-11.1251922069943));
#64656=CARTESIAN_POINT('Ctrl Pts',(41.022502515718,-10.8488204646873,-11.0949440545143));
#64657=CARTESIAN_POINT('Ctrl Pts',(41.0352776930479,-10.8504698925187,-11.0799905126656));
#64658=CARTESIAN_POINT('Ctrl Pts',(41.0654188628578,-10.8544367223528,-11.0438209383249));
#64659=CARTESIAN_POINT('Ctrl Pts',(41.0826078785501,-10.8567609377225,-11.0224618588037));
#64660=CARTESIAN_POINT('Ctrl Pts',(41.1437855434125,-10.8652672820721,-10.9437239671596));
#64661=CARTESIAN_POINT('Ctrl Pts',(41.1855419730588,-10.8715324270427,-10.8846693403957));
#64662=CARTESIAN_POINT('Ctrl Pts',(41.2897916053692,-10.888491048448,-10.7221686343017));
#64663=CARTESIAN_POINT('Ctrl Pts',(41.3472545971897,-10.8993200646208,-10.6157490115158));
#64664=CARTESIAN_POINT('Ctrl Pts',(41.4443014108719,-10.9207168285928,-10.3983435042842));
#64665=CARTESIAN_POINT('Ctrl Pts',(41.4842273844128,-10.9312539053336,-10.2878425800484));
#64666=CARTESIAN_POINT('Ctrl Pts',(41.5228670610808,-10.9437110362452,-10.1501404901966));
#64667=CARTESIAN_POINT('Ctrl Pts',(41.5294072050516,-10.9459308670538,-10.1253117937378));
#64668=CARTESIAN_POINT('Ctrl Pts',(41.5386719509606,-10.9492491928116,-10.0877049862597));
#64669=CARTESIAN_POINT('Ctrl Pts',(41.5416918082754,-10.9503625111018,-10.0750026320766));
#64670=CARTESIAN_POINT('Ctrl Pts',(41.5467934001117,-10.9522999563364,-10.0527398900864));
#64671=CARTESIAN_POINT('Ctrl Pts',(41.5489203725474,-10.9531264921375,-10.0431908399045));
#64672=CARTESIAN_POINT('Ctrl Pts',(41.5539219056732,-10.9551169174535,-10.0200726883061));
#64673=CARTESIAN_POINT('Ctrl Pts',(41.5567374648022,-10.9562775286216,-10.0064912829887));
#64674=CARTESIAN_POINT('Ctrl Pts',(41.5652734111053,-10.9599306815867,-9.96344655767705));
#64675=CARTESIAN_POINT('Ctrl Pts',(41.5705602424409,-10.9624010495705,-9.9338986166187));
#64676=CARTESIAN_POINT('Ctrl Pts',(41.5820485305772,-10.9683438481892,-9.86194736065849));
#64677=CARTESIAN_POINT('Ctrl Pts',(41.5876728879078,-10.9717921789487,-9.81946125311835));
#64678=CARTESIAN_POINT('Ctrl Pts',(41.6076393388287,-10.9870075235218,-9.62980887855387));
#64679=CARTESIAN_POINT('Ctrl Pts',(41.6095306903536,-10.9984375474365,-9.48165181689282));
#64680=CARTESIAN_POINT('Ctrl Pts',(41.5895254900321,-11.0183151823196,-9.23017599949378));
#64681=CARTESIAN_POINT('Ctrl Pts',(41.5744801152151,-11.0266261326242,-9.12676281801236));
#64682=CARTESIAN_POINT('Ctrl Pts',(41.5462617575271,-11.0376953917936,-8.99406967398162));
#64683=CARTESIAN_POINT('Ctrl Pts',(41.5391599541552,-11.0402643627764,-8.96360729170602));
#64684=CARTESIAN_POINT('Ctrl Pts',(41.5264490211558,-11.0445395322422,-8.91352315235615));
#64685=CARTESIAN_POINT('Ctrl Pts',(41.5211803938592,-11.0462348399066,-8.89381816489547));
#64686=CARTESIAN_POINT('Ctrl Pts',(41.5103178428527,-11.0495877526568,-8.85516827798776));
#64687=CARTESIAN_POINT('Ctrl Pts',(41.5047398724836,-11.0512447256363,-8.83622054232609));
#64688=CARTESIAN_POINT('Ctrl Pts',(41.4907178594649,-11.0552616691938,-8.79066786067397));
#64689=CARTESIAN_POINT('Ctrl Pts',(41.482043032499,-11.0576289101027,-8.76413768701433));
#64690=CARTESIAN_POINT('Ctrl Pts',(41.4479111557556,-11.0665304887987,-8.6655918782574));
#64691=CARTESIAN_POINT('Ctrl Pts',(41.419493070404,-11.0731585308123,-8.5946588186566));
#64692=CARTESIAN_POINT('Ctrl Pts',(41.3302585507642,-11.0920503395271,-8.39939569306689));
#64693=CARTESIAN_POINT('Ctrl Pts',(41.2620240332296,-11.1045045809736,-8.27879140406469));
#64694=CARTESIAN_POINT('Ctrl Pts',(41.1252113916338,-11.1262220760604,-8.07926372538336));
#64695=CARTESIAN_POINT('Ctrl Pts',(41.0611372446436,-11.1354750028157,-7.9976605204486));
#64696=CARTESIAN_POINT('Ctrl Pts',(40.978401595812,-11.1462198305567,-7.90526061308855));
#64697=CARTESIAN_POINT('Ctrl Pts',(40.9646197924781,-11.1479734971254,-7.89025690395843));
#64698=CARTESIAN_POINT('Ctrl Pts',(40.9424460428653,-11.1507360063675,-7.86672445441237));
#64699=CARTESIAN_POINT('Ctrl Pts',(40.9341786524732,-11.1517533583101,-7.85808056045626));
#64700=CARTESIAN_POINT('Ctrl Pts',(40.9180411779184,-11.1537142768979,-7.84145818909626));
#64701=CARTESIAN_POINT('Ctrl Pts',(40.9101793057365,-11.1546583440911,-7.83347250408296));
#64702=CARTESIAN_POINT('Ctrl Pts',(40.8904116176671,-11.1570050538713,-7.81367220510285));
#64703=CARTESIAN_POINT('Ctrl Pts',(40.8784371573212,-11.1584025348881,-7.80192628807131));
#64704=CARTESIAN_POINT('Ctrl Pts',(40.8300705285717,-11.1639570157993,-7.75546549099086));
#64705=CARTESIAN_POINT('Ctrl Pts',(40.7927133037988,-11.168046577823,-7.7217674433887));
#64706=CARTESIAN_POINT('Ctrl Pts',(40.5889342179779,-11.1895000061557,-7.54922722663526));
#64707=CARTESIAN_POINT('Ctrl Pts',(40.405373956332,-11.206003068983,-7.43217787512118));
#64708=CARTESIAN_POINT('Ctrl Pts',(40.1525624862095,-11.2282730897704,-7.31540989973278));
#64709=CARTESIAN_POINT('Ctrl Pts',(40.0955493997673,-11.2332610788826,-7.29169443044493));
#64710=CARTESIAN_POINT('Ctrl Pts',(40.0151766737935,-11.2402889462241,-7.26183477666319));
#64711=CARTESIAN_POINT('Ctrl Pts',(39.9925384884744,-11.2422679293991,-7.25380813272534));
#64712=CARTESIAN_POINT('Ctrl Pts',(39.9511412189918,-11.2458883806525,-7.23982450275232));
#64713=CARTESIAN_POINT('Ctrl Pts',(39.9324217437083,-11.2475260948706,-7.23375611834104));
#64714=CARTESIAN_POINT('Ctrl Pts',(39.894349171778,-11.2508594217414,-7.22192817682606));
#64715=CARTESIAN_POINT('Ctrl Pts',(39.874993841179,-11.2525552946411,-7.21618128553747));
#64716=CARTESIAN_POINT('Ctrl Pts',(39.8264830836253,-11.2568102955336,-7.20243982466638));
#64717=CARTESIAN_POINT('Ctrl Pts',(39.7972458360909,-11.2593789056762,-7.19475021628325));
#64718=CARTESIAN_POINT('Ctrl Pts',(39.6705748379916,-11.2705311119887,-7.16397523146468));
#64719=CARTESIAN_POINT('Ctrl Pts',(39.571911203467,-11.2792833309542,-7.1464384690286));
#64720=CARTESIAN_POINT('Ctrl Pts',(39.3201977297819,-11.3017738485723,-7.11774238386917));
#64721=CARTESIAN_POINT('Ctrl Pts',(39.1666401786788,-11.3156599356947,-7.11497513495131));
#64722=CARTESIAN_POINT('Ctrl Pts',(38.9508263075888,-11.3349265170344,-7.13172532438285));
#64723=CARTESIAN_POINT('Ctrl Pts',(38.8879944091471,-11.3405009498216,-7.13910279687247));
#64724=CARTESIAN_POINT('Ctrl Pts',(38.8071905235519,-11.3475720191562,-7.15183798004175));
#64725=CARTESIAN_POINT('Ctrl Pts',(38.7888942573365,-11.3491665098539,-7.15493894777457));
#64726=CARTESIAN_POINT('Ctrl Pts',(38.7592486012549,-11.3517375014518,-7.16031713274855));
#64727=CARTESIAN_POINT('Ctrl Pts',(38.7478770216168,-11.352720670949,-7.16246498688973));
#64728=CARTESIAN_POINT('Ctrl Pts',(38.7252332551786,-11.3546718214504,-7.16691140775319));
#64729=CARTESIAN_POINT('Ctrl Pts',(38.7139611885625,-11.3556398252072,-7.16920893092704));
#64730=CARTESIAN_POINT('Ctrl Pts',(38.6848789464987,-11.3581298717878,-7.17535423369443));
#64731=CARTESIAN_POINT('Ctrl Pts',(38.6670947500283,-11.359645346537,-7.17932376844657));
#64732=CARTESIAN_POINT('Ctrl Pts',(38.5857779917595,-11.3665489807708,-7.19844674428742));
#64733=CARTESIAN_POINT('Ctrl Pts',(38.5228270631866,-11.3718212782781,-7.21598342055357));
#64734=CARTESIAN_POINT('Ctrl Pts',(38.3081413857634,-11.3898042757577,-7.28532805048672));
#64735=CARTESIAN_POINT('Ctrl Pts',(38.1609219435414,-11.4021644674764,-7.34971513679241));
#64736=CARTESIAN_POINT('Ctrl Pts',(37.941235538372,-11.4220918536305,-7.47322529008722));
#64737=CARTESIAN_POINT('Ctrl Pts',(37.8639219058059,-11.4294249864097,-7.52271146340682));
#64738=CARTESIAN_POINT('Ctrl Pts',(37.7652077726044,-11.4393786760974,-7.59416259753143));
#64739=CARTESIAN_POINT('Ctrl Pts',(37.7411220416127,-11.4418569256409,-7.61229595873185));
#64740=CARTESIAN_POINT('Ctrl Pts',(37.7030816107448,-11.4458561599467,-7.6420719097457));
#64741=CARTESIAN_POINT('Ctrl Pts',(37.6889063963383,-11.4473659777947,-7.65342875091646));
#64742=CARTESIAN_POINT('Ctrl Pts',(37.659685460767,-11.4505204633043,-7.67738823890888));
#64743=CARTESIAN_POINT('Ctrl Pts',(37.6446627183865,-11.4521660767446,-7.69001662371618));
#64744=CARTESIAN_POINT('Ctrl Pts',(37.6092371505462,-11.4561053771815,-7.72054355289071));
#64745=CARTESIAN_POINT('Ctrl Pts',(37.588979910956,-11.4584056218504,-7.73860596290142));
#64746=CARTESIAN_POINT('Ctrl Pts',(37.5175036837037,-11.4666989912739,-7.80454247878495));
#64747=CARTESIAN_POINT('Ctrl Pts',(37.4680827200657,-11.4727696434315,-7.85430302754183));
#64748=CARTESIAN_POINT('Ctrl Pts',(37.339063270394,-11.4895916436224,-7.99609291303347));
#64749=CARTESIAN_POINT('Ctrl Pts',(37.2641647155925,-11.5004891065534,-8.0921085710049));
#64750=CARTESIAN_POINT('Ctrl Pts',(37.1307908826643,-11.5221406781137,-8.29273923816963));
#64751=CARTESIAN_POINT('Ctrl Pts',(37.072207700021,-11.5328631560084,-8.39690475642306));
#64752=CARTESIAN_POINT('Ctrl Pts',(37.0106895824316,-11.5454994911493,-8.52828832563821));
#64753=CARTESIAN_POINT('Ctrl Pts',(37.0001581503638,-11.5477231729444,-8.55175272190109));
#64754=CARTESIAN_POINT('Ctrl Pts',(36.9848465490632,-11.5510460987544,-8.58738663269681));
#64755=CARTESIAN_POINT('Ctrl Pts',(36.979786344245,-11.5521602228075,-8.59943261452653));
#64756=CARTESIAN_POINT('Ctrl Pts',(36.9706968990618,-11.5541905416767,-8.62157388130927));
#64757=CARTESIAN_POINT('Ctrl Pts',(36.9666377179502,-11.5551083543723,-8.63165572388229));
#64758=CARTESIAN_POINT('Ctrl Pts',(36.9610940144708,-11.5563777321211,-8.64569867865025));
#64759=CARTESIAN_POINT('Ctrl Pts',(36.9595516596191,-11.556732665845,-8.64963604120397));
#64760=CARTESIAN_POINT('Ctrl Pts',(36.9580196848654,-11.5570870138823,-8.65357747851634));
#64761=CARTESIAN_POINT('Origin',(39.2,5.9,-9.525));
#64762=CARTESIAN_POINT('',(36.0897704597331,5.287170157044,-9.52330892006467));
#64763=CARTESIAN_POINT('',(40.6132835138381,5.69998730739364,-6.75441154943334));
#64764=CARTESIAN_POINT('Ctrl Pts',(36.0897704597335,5.28717015708686,-9.52330891940844));
#64765=CARTESIAN_POINT('Ctrl Pts',(36.0898186087208,5.29295414852404,-9.43475346949347));
#64766=CARTESIAN_POINT('Ctrl Pts',(36.093648521948,5.29873813996121,-9.34629745832044));
#64767=CARTESIAN_POINT('Ctrl Pts',(36.1012366733098,5.30452213139838,-9.25817328083612));
#64768=CARTESIAN_POINT('Ctrl Pts',(36.1095595677739,5.31086617331557,-9.16151624357196));
#64769=CARTESIAN_POINT('Ctrl Pts',(36.1224233930836,5.31721021523276,-9.0650837361024));
#64770=CARTESIAN_POINT('Ctrl Pts',(36.1398093077089,5.32355425714994,-8.96933501125699));
#64771=CARTESIAN_POINT('Ctrl Pts',(36.1571717859258,5.32988974722729,-8.87371535676938));
#64772=CARTESIAN_POINT('Ctrl Pts',(36.1790441594873,5.33622523730464,-8.77877807778213));
#64773=CARTESIAN_POINT('Ctrl Pts',(36.2053557432597,5.34256072738198,-8.68497831666542));
#64774=CARTESIAN_POINT('Ctrl Pts',(36.2316396524023,5.34888955376535,-8.59127721451519));
#64775=CARTESIAN_POINT('Ctrl Pts',(36.2623533713891,5.35521838014872,-8.4987116686923));
#64776=CARTESIAN_POINT('Ctrl Pts',(36.2973751696389,5.3615472065321,-8.40772664621805));
#64777=CARTESIAN_POINT('Ctrl Pts',(36.3323715300516,5.36787143601689,-8.31680771007555));
#64778=CARTESIAN_POINT('Ctrl Pts',(36.3716695917911,5.37419566550169,-8.22746742000405));
#64779=CARTESIAN_POINT('Ctrl Pts',(36.4150980812374,5.38051989498649,-8.14013467955456));
#64780=CARTESIAN_POINT('Ctrl Pts',(36.4585103955461,5.38684176898338,-8.05283446657974));
#64781=CARTESIAN_POINT('Ctrl Pts',(36.5060498866431,5.39316364298027,-7.96754070695239));
#64782=CARTESIAN_POINT('Ctrl Pts',(36.5574979048968,5.39948551697716,-7.88466060515663));
#64783=CARTESIAN_POINT('Ctrl Pts',(36.6089405603399,5.40580673199799,-7.80178914257183));
#64784=CARTESIAN_POINT('Ctrl Pts',(36.664290702917,5.41212794701881,-7.72133120751426));
#64785=CARTESIAN_POINT('Ctrl Pts',(36.7232851845049,5.41844916203964,-7.64366686214077));
#64786=CARTESIAN_POINT('Ctrl Pts',(36.7822893395842,5.4247714135679,-7.56598978192578));
#64787=CARTESIAN_POINT('Ctrl Pts',(36.84493875699,5.43109366509616,-7.49110754802284));
#64788=CARTESIAN_POINT('Ctrl Pts',(36.9109293061056,5.43741591662442,-7.41936802568588));
#64789=CARTESIAN_POINT('Ctrl Pts',(36.9769880025767,5.44374469703791,-7.34755441912344));
#64790=CARTESIAN_POINT('Ctrl Pts',(37.0463944240091,5.45007347745141,-7.2788903247904));
#64791=CARTESIAN_POINT('Ctrl Pts',(37.1188069345913,5.4564022578649,-7.21368736917858));
#64792=CARTESIAN_POINT('Ctrl Pts',(37.1912605533614,5.46273463109256,-7.14844739820395));
#64793=CARTESIAN_POINT('Ctrl Pts',(37.2667233231194,5.46906700432022,-7.08667275512045));
#64794=CARTESIAN_POINT('Ctrl Pts',(37.3448214302059,5.47539937754789,-7.02863401579883));
#64795=CARTESIAN_POINT('Ctrl Pts',(37.423041153471,5.4817416116936,-6.97050489721));
#64796=CARTESIAN_POINT('Ctrl Pts',(37.5039040477082,5.48808384583931,-6.91612354267705));
#64797=CARTESIAN_POINT('Ctrl Pts',(37.5870083665495,5.49442607998502,-6.86571651693195));
#64798=CARTESIAN_POINT('Ctrl Pts',(37.6337516315119,5.49799336427614,-6.83736433267458));
#64799=CARTESIAN_POINT('Ctrl Pts',(37.6812035684037,5.50156064856726,-6.81026865835675));
#64800=CARTESIAN_POINT('Ctrl Pts',(37.7292897654297,5.50512793285838,-6.78446318053741));
#64801=CARTESIAN_POINT('Ctrl Pts',(37.8143208444197,5.51143598072031,-6.7388312163036));
#64802=CARTESIAN_POINT('Ctrl Pts',(37.9016290082981,5.51774402858223,-6.6970792600513));
#64803=CARTESIAN_POINT('Ctrl Pts',(37.9908238206751,5.52405207644415,-6.6594418309423));
#64804=CARTESIAN_POINT('Ctrl Pts',(38.0799001524758,5.53035174510636,-6.62185439694147));
#64805=CARTESIAN_POINT('Ctrl Pts',(38.170857749694,5.53665141376857,-6.58837079902755));
#64806=CARTESIAN_POINT('Ctrl Pts',(38.2632811158576,5.54295108243077,-6.55917998101857));
#64807=CARTESIAN_POINT('Ctrl Pts',(38.3592770146033,5.54949425847089,-6.52886082119773));
#64808=CARTESIAN_POINT('Ctrl Pts',(38.4568538782844,5.55603743451101,-6.50317327731934));
#64809=CARTESIAN_POINT('Ctrl Pts',(38.5555224272059,5.56258061055113,-6.48227436151968));
#64810=CARTESIAN_POINT('Ctrl Pts',(38.6503563799917,5.56886949646706,-6.46218764882469));
#64811=CARTESIAN_POINT('Ctrl Pts',(38.7461982684,5.57515838238298,-6.44652438776735));
#64812=CARTESIAN_POINT('Ctrl Pts',(38.8425989931736,5.58144726829891,-6.43537297182663));
#64813=CARTESIAN_POINT('Ctrl Pts',(38.9389691045005,5.58773415708801,-6.42422509717958));
#64814=CARTESIAN_POINT('Ctrl Pts',(39.0358972618107,5.5940210458771,-6.41758627158632));
#64815=CARTESIAN_POINT('Ctrl Pts',(39.1329269213326,5.6003079346662,-6.41549331002198));
#64816=CARTESIAN_POINT('Ctrl Pts',(39.2299525855833,5.60659456458779,-6.41340043463695));
#64817=CARTESIAN_POINT('Ctrl Pts',(39.3270793027399,5.61288119450939,-6.41585305997413));
#64818=CARTESIAN_POINT('Ctrl Pts',(39.4238492929252,5.61916782443098,-6.42283589296813));
#64819=CARTESIAN_POINT('Ctrl Pts',(39.5206420447427,5.62545593305437,-6.42982036842044));
#64820=CARTESIAN_POINT('Ctrl Pts',(39.6170774631422,5.63174404167775,-6.44133713569765));
#64821=CARTESIAN_POINT('Ctrl Pts',(39.7127027584188,5.63803215030114,-6.45731902988435));
#64822=CARTESIAN_POINT('Ctrl Pts',(39.8084320099681,5.64432709485985,-6.47331829832484));
#64823=CARTESIAN_POINT('Ctrl Pts',(39.9033489454962,5.65062203941857,-6.49379230721495));
#64824=CARTESIAN_POINT('Ctrl Pts',(39.9970111559666,5.65691698397728,-6.51862279975302));
#64825=CARTESIAN_POINT('Ctrl Pts',(40.0907338317231,5.6632159923481,-6.54346932205198));
#64826=CARTESIAN_POINT('Ctrl Pts',(40.1831997504376,5.66951500071891,-6.57267779281377));
#64827=CARTESIAN_POINT('Ctrl Pts',(40.2739838418386,5.67581400908973,-6.60608078899577));
#64828=CARTESIAN_POINT('Ctrl Pts',(40.3649048763921,5.68212251919207,-6.63953417188681));
#64829=CARTESIAN_POINT('Ctrl Pts',(40.4541386166821,5.68843102929442,-6.6771945337928));
#64830=CARTESIAN_POINT('Ctrl Pts',(40.5412823371517,5.69473953939677,-6.71884741239094));
#64831=CARTESIAN_POINT('Ctrl Pts',(40.5654459943908,5.69648879539572,-6.73039713595159));
#64832=CARTESIAN_POINT('Ctrl Pts',(40.5894491185416,5.69823805139468,-6.74225356980704));
#64833=CARTESIAN_POINT('Ctrl Pts',(40.6132835138381,5.69998730739364,-6.75441154943334));
#64834=CARTESIAN_POINT('',(37.7868905613917,5.7,-6.75432276015119));
#64835=CARTESIAN_POINT('Origin',(39.2,5.7,-9.525));
#64836=CARTESIAN_POINT('',(36.0893719342297,5.47782984291316,-9.52215481026634));
#64837=CARTESIAN_POINT('Ctrl Pts',(37.7868905613917,5.7,-6.75432276015119));
#64838=CARTESIAN_POINT('Ctrl Pts',(36.8702811367888,5.63313139951334,-7.22181475481399));
#64839=CARTESIAN_POINT('Ctrl Pts',(36.1407178101623,5.55907468048439,-8.27832117013194));
#64840=CARTESIAN_POINT('Ctrl Pts',(36.0859047902816,5.48501796145545,-9.41200135228371));
#64841=CARTESIAN_POINT('Ctrl Pts',(36.0866947581083,5.47782984291316,-9.52215236154092));
#64842=CARTESIAN_POINT('',(36.090096854374,4.20782989897492,-9.52397950441223));
#64843=CARTESIAN_POINT('Ctrl Pts',(36.0897713010337,5.47782984291316,-9.52215517555409));
#64844=CARTESIAN_POINT('Ctrl Pts',(36.0896845820882,5.47163671312522,-9.61696445391203));
#64845=CARTESIAN_POINT('Ctrl Pts',(36.0939371013632,5.46544358333727,-9.71197140607672));
#64846=CARTESIAN_POINT('Ctrl Pts',(36.1025565077274,5.45925045354932,-9.8067347424057));
#64847=CARTESIAN_POINT('Ctrl Pts',(36.111164773093,5.45306532868048,-9.90137559254964));
#64848=CARTESIAN_POINT('Ctrl Pts',(36.1241286777308,5.44688020381164,-9.99577300073165));
#64849=CARTESIAN_POINT('Ctrl Pts',(36.1414238647493,5.44069507894279,-10.08948443537));
#64850=CARTESIAN_POINT('Ctrl Pts',(36.1587018744572,5.43451609704374,-10.1831027972695));
#64851=CARTESIAN_POINT('Ctrl Pts',(36.180302538393,5.42833711514468,-10.276036091567));
#64852=CARTESIAN_POINT('Ctrl Pts',(36.206149703286,5.42215813324563,-10.3678469930927));
#64853=CARTESIAN_POINT('Ctrl Pts',(36.2319831605192,5.41598242827781,-10.4596092040711));
#64854=CARTESIAN_POINT('Ctrl Pts',(36.2620585261269,5.40980672330998,-10.550249764139));
#64855=CARTESIAN_POINT('Ctrl Pts',(36.2962488119258,5.40363101834216,-10.6393427168774));
#64856=CARTESIAN_POINT('Ctrl Pts',(36.3304311027509,5.39745675748626,-10.728414836335));
#64857=CARTESIAN_POINT('Ctrl Pts',(36.368726239351,5.39128249663036,-10.8159396400812));
#64858=CARTESIAN_POINT('Ctrl Pts',(36.4109581736926,5.38510823577446,-10.901508751882));
#64859=CARTESIAN_POINT('Ctrl Pts',(36.4531927534159,5.37893358816677,-10.987083223678));
#64860=CARTESIAN_POINT('Ctrl Pts',(36.4993644161621,5.37275894055907,-11.070701350939));
#64861=CARTESIAN_POINT('Ctrl Pts',(36.5492506059328,5.36658429295137,-11.1519782735957));
#64862=CARTESIAN_POINT('Ctrl Pts',(36.5991859844777,5.36040355701846,-11.2333353369127));
#64863=CARTESIAN_POINT('Ctrl Pts',(36.6528429610527,5.35422282108556,-11.312346197209));
#64864=CARTESIAN_POINT('Ctrl Pts',(36.709955245206,5.34804208515265,-11.3886544132491));
#64865=CARTESIAN_POINT('Ctrl Pts',(36.7670975456727,5.34185810083089,-11.4650027343447));
#64866=CARTESIAN_POINT('Ctrl Pts',(36.8276984744866,5.33567411650914,-11.5386452336246));
#64867=CARTESIAN_POINT('Ctrl Pts',(36.8914525110087,5.32949013218739,-11.6092598551936));
#64868=CARTESIAN_POINT('Ctrl Pts',(36.9553103802596,5.32329607634698,-11.679989482953));
#64869=CARTESIAN_POINT('Ctrl Pts',(37.022331284959,5.31710202050658,-11.747681066423));
#64870=CARTESIAN_POINT('Ctrl Pts',(37.092174261948,5.31090796466618,-11.8120507888776));
#64871=CARTESIAN_POINT('Ctrl Pts',(37.1377268961641,5.30686810880413,-11.8540336846242));
#64872=CARTESIAN_POINT('Ctrl Pts',(37.1844793126437,5.30282825294209,-11.8946043393667));
#64873=CARTESIAN_POINT('Ctrl Pts',(37.2323302861203,5.29878839708004,-11.9336939510824));
#64874=CARTESIAN_POINT('Ctrl Pts',(37.3074239402655,5.2924485565949,-11.9950381948787));
#64875=CARTESIAN_POINT('Ctrl Pts',(37.3855179670266,5.28610871610976,-12.0529727414287));
#64876=CARTESIAN_POINT('Ctrl Pts',(37.4662702301628,5.27976887562462,-12.10719126675));
#64877=CARTESIAN_POINT('Ctrl Pts',(37.5469137842503,5.27343756986037,-12.1613368028563));
#64878=CARTESIAN_POINT('Ctrl Pts',(37.6302081027073,5.26710626409612,-12.2117760199869));
#64879=CARTESIAN_POINT('Ctrl Pts',(37.7157778598847,5.26077495833187,-12.2582426331542));
#64880=CARTESIAN_POINT('Ctrl Pts',(37.8012578484924,5.2544502945435,-12.3046604996434));
#64881=CARTESIAN_POINT('Ctrl Pts',(37.8890081486045,5.24812563075512,-12.3471138408602));
#64882=CARTESIAN_POINT('Ctrl Pts',(37.9786251560617,5.24180096696674,-12.3853800697626));
#64883=CARTESIAN_POINT('Ctrl Pts',(38.0681776933297,5.23548085312132,-12.4236187700619));
#64884=CARTESIAN_POINT('Ctrl Pts',(38.1595938679232,5.22916073927589,-12.4576761763042));
#64885=CARTESIAN_POINT('Ctrl Pts',(38.2524470688899,5.22284062543047,-12.4873764270674));
#64886=CARTESIAN_POINT('Ctrl Pts',(38.345266110195,5.21652283668475,-12.5170657514382));
#64887=CARTESIAN_POINT('Ctrl Pts',(38.4395207123484,5.21020504793904,-12.5424009729244));
#64888=CARTESIAN_POINT('Ctrl Pts',(38.5347668204555,5.20388725919333,-12.5632553332024));
#64889=CARTESIAN_POINT('Ctrl Pts',(38.6300035147641,5.19757009487617,-12.5841076323071));
#64890=CARTESIAN_POINT('Ctrl Pts',(38.7262310940903,5.19125293055902,-12.6004798577207));
#64891=CARTESIAN_POINT('Ctrl Pts',(38.8229939761624,5.18493576624186,-12.6122960840985));
#64892=CARTESIAN_POINT('Ctrl Pts',(38.9197733282269,5.17861752668133,-12.6241143217141));
#64893=CARTESIAN_POINT('Ctrl Pts',(39.0170877310747,5.17229928712079,-12.6313749672716));
#64894=CARTESIAN_POINT('Ctrl Pts',(39.1144761579347,5.16598104756026,-12.6340539276987));
#64895=CARTESIAN_POINT('Ctrl Pts',(39.2119664658373,5.15965619829409,-12.6367356906689));
#64896=CARTESIAN_POINT('Ctrl Pts',(39.3095305156666,5.15333134902793,-12.6348261872233));
#64897=CARTESIAN_POINT('Ctrl Pts',(39.4067071575398,5.14700649976176,-12.628353477115));
#64898=CARTESIAN_POINT('Ctrl Pts',(39.5039396160097,5.14067801761063,-12.621877049193));
#64899=CARTESIAN_POINT('Ctrl Pts',(39.6007837901789,5.1343495354595,-12.6108322441893));
#64900=CARTESIAN_POINT('Ctrl Pts',(39.6967855871465,5.12802105330837,-12.5952988019578));
#64901=CARTESIAN_POINT('Ctrl Pts',(39.7929384685036,5.12168261160552,-12.5797409137189));
#64902=CARTESIAN_POINT('Ctrl Pts',(39.8882458988043,5.11534416990267,-12.5596803719045));
#64903=CARTESIAN_POINT('Ctrl Pts',(39.9822659189178,5.10900572819981,-12.5352476119083));
#64904=CARTESIAN_POINT('Ctrl Pts',(40.0357801837033,5.10539801733989,-12.5213409866354));
#64905=CARTESIAN_POINT('Ctrl Pts',(40.0888776682847,5.10179030647997,-12.506018824456));
#64906=CARTESIAN_POINT('Ctrl Pts',(40.1414797165299,5.09818259562005,-12.4893121624186));
#64907=CARTESIAN_POINT('Ctrl Pts',(40.2339622594588,5.09183968150153,-12.4599392645826));
#64908=CARTESIAN_POINT('Ctrl Pts',(40.3252235287212,5.08549676738301,-12.4261851533917));
#64909=CARTESIAN_POINT('Ctrl Pts',(40.4148198060276,5.07915385326449,-12.3881701821203));
#64910=CARTESIAN_POINT('Ctrl Pts',(40.504298514821,5.07281926233756,-12.3502050942123));
#64911=CARTESIAN_POINT('Ctrl Pts',(40.5921161766902,5.06648467141063,-12.3079904287888));
#64912=CARTESIAN_POINT('Ctrl Pts',(40.6778446151691,5.06015008048369,-12.2616961735486));
#64913=CARTESIAN_POINT('Ctrl Pts',(40.7634859526157,5.05382192557051,-12.2154489537788));
#64914=CARTESIAN_POINT('Ctrl Pts',(40.8470419056743,5.04749377065732,-12.1651305912952));
#64915=CARTESIAN_POINT('Ctrl Pts',(40.9281055745149,5.04116561574414,-12.1109585797593));
#64916=CARTESIAN_POINT('Ctrl Pts',(41.0091147299018,5.03484171636965,-12.0568229976558));
#64917=CARTESIAN_POINT('Ctrl Pts',(41.0876345718574,5.02851781699517,-11.9988391599899));
#64918=CARTESIAN_POINT('Ctrl Pts',(41.1632848624888,5.02219391762068,-11.9372693053683));
#64919=CARTESIAN_POINT('Ctrl Pts',(41.238909503085,5.01587216243151,-11.8757203266605));
#64920=CARTESIAN_POINT('Ctrl Pts',(41.311666188255,5.00955040724233,-11.8105880219351));
#64921=CARTESIAN_POINT('Ctrl Pts',(41.3812063787698,5.00322865205315,-11.7421759934913));
#64922=CARTESIAN_POINT('Ctrl Pts',(41.4507416429264,4.99690734470903,-11.6737688114845));
#64923=CARTESIAN_POINT('Ctrl Pts',(41.5170605551517,4.99058603736491,-11.6020826734505));
#64924=CARTESIAN_POINT('Ctrl Pts',(41.5798509405664,4.9842647300208,-11.5274585273072));
#64925=CARTESIAN_POINT('Ctrl Pts',(41.6426537189718,4.97794217503499,-11.452819652534));
#64926=CARTESIAN_POINT('Ctrl Pts',(41.701926306672,4.97161962004918,-11.3752419510508));
#64927=CARTESIAN_POINT('Ctrl Pts',(41.7573970375836,4.96529706506337,-11.2950991624931));
#64928=CARTESIAN_POINT('Ctrl Pts',(41.8129278532602,4.95896766161487,-11.2148695649004));
#64929=CARTESIAN_POINT('Ctrl Pts',(41.8646483422961,4.95263825816637,-11.1320696919911));
#64930=CARTESIAN_POINT('Ctrl Pts',(41.9123305013042,4.94630885471787,-11.0471018049378));
#64931=CARTESIAN_POINT('Ctrl Pts',(41.9600410945071,4.93997567687043,-10.9620832491752));
#64932=CARTESIAN_POINT('Ctrl Pts',(42.0037083670312,4.93364249902299,-10.8748944939855));
#64933=CARTESIAN_POINT('Ctrl Pts',(42.0431514999804,4.92730932117555,-10.7859600315075));
#64934=CARTESIAN_POINT('Ctrl Pts',(42.0826577742244,4.9209660050602,-10.6968832011014));
#64935=CARTESIAN_POINT('Ctrl Pts',(42.117926248496,4.91462268894484,-10.6060554889158));
#64936=CARTESIAN_POINT('Ctrl Pts',(42.1488252210036,4.90827937282948,-10.5139188383651));
#64937=CARTESIAN_POINT('Ctrl Pts',(42.16620302351,4.90471184660635,-10.4621005289865));
#64938=CARTESIAN_POINT('Ctrl Pts',(42.1821996577844,4.90114432038321,-10.4098684426213));
#64939=CARTESIAN_POINT('Ctrl Pts',(42.196798807768,4.89757679416008,-10.3573025643722));
#64940=CARTESIAN_POINT('Ctrl Pts',(42.2226830905886,4.89125157263462,-10.2641032986035));
#64941=CARTESIAN_POINT('Ctrl Pts',(42.2442615259797,4.88492635110916,-10.169529793704));
#64942=CARTESIAN_POINT('Ctrl Pts',(42.261390504317,4.8786011295837,-10.0740162410875));
#64943=CARTESIAN_POINT('Ctrl Pts',(42.2784961340242,4.8722845300119,-9.97863288366201));
#64944=CARTESIAN_POINT('Ctrl Pts',(42.291164283726,4.8659679304401,-9.88231245299431));
#64945=CARTESIAN_POINT('Ctrl Pts',(42.2993012966942,4.8596513308683,-9.78550359922624));
#64946=CARTESIAN_POINT('Ctrl Pts',(42.3074296686005,4.85334143917913,-9.68879755115629));
#64947=CARTESIAN_POINT('Ctrl Pts',(42.3110364326971,4.84703154748996,-9.59160454565647));
#64948=CARTESIAN_POINT('Ctrl Pts',(42.310079287173,4.84072165580079,-9.49438169832463));
#64949=CARTESIAN_POINT('Ctrl Pts',(42.3091228371721,4.83441634928264,-9.39722949933418));
#64950=CARTESIAN_POINT('Ctrl Pts',(42.3036090748728,4.82811104276449,-9.30004793881186));
#64951=CARTESIAN_POINT('Ctrl Pts',(42.2935477251791,4.82180573624634,-9.20329652637949));
#64952=CARTESIAN_POINT('Ctrl Pts',(42.2834901108703,4.81550277064146,-9.10658103395573));
#64953=CARTESIAN_POINT('Ctrl Pts',(42.2688883089752,4.80919980503657,-9.0102958080121));
#64954=CARTESIAN_POINT('Ctrl Pts',(42.2498040233362,4.80289683943168,-8.91489667092989));
#64955=CARTESIAN_POINT('Ctrl Pts',(42.2307216194919,4.79659449532698,-8.81950694062298));
#64956=CARTESIAN_POINT('Ctrl Pts',(42.2071576968169,4.79029215122228,-8.72500355541852));
#64957=CARTESIAN_POINT('Ctrl Pts',(42.1792251473581,4.78398980711758,-8.63183250493014));
#64958=CARTESIAN_POINT('Ctrl Pts',(42.1512877362539,4.77768636609325,-8.53864523807026));
#64959=CARTESIAN_POINT('Ctrl Pts',(42.1189803143276,4.77138292506893,-8.44679118646755));
#64960=CARTESIAN_POINT('Ctrl Pts',(42.0824654273109,4.76507948404461,-8.3567005036133));
#64961=CARTESIAN_POINT('Ctrl Pts',(42.0459115304473,4.7587693088828,-8.26651357443237));
#64962=CARTESIAN_POINT('Ctrl Pts',(42.0051413596025,4.752459133721,-8.17809418206875));
#64963=CARTESIAN_POINT('Ctrl Pts',(41.9603652649566,4.7461489585592,-8.09185162773666));
#64964=CARTESIAN_POINT('Ctrl Pts',(41.9155630444213,4.73983510154573,-8.00555875272652));
#64965=CARTESIAN_POINT('Ctrl Pts',(41.8667504660697,4.73352124453225,-7.92144562385831));
#64966=CARTESIAN_POINT('Ctrl Pts',(41.8141823393613,4.72720738751878,-7.83989426163472));
#64967=CARTESIAN_POINT('Ctrl Pts',(41.7615294415422,4.72088334880958,-7.75821139007305));
#64968=CARTESIAN_POINT('Ctrl Pts',(41.7051091568404,4.71455931010037,-7.67909889090502));
#64969=CARTESIAN_POINT('Ctrl Pts',(41.6452178075563,4.70823527139117,-7.60290725340594));
#64970=CARTESIAN_POINT('Ctrl Pts',(41.6096586298144,4.70448051182747,-7.55767013631543));
#64971=CARTESIAN_POINT('Ctrl Pts',(41.5728766039077,4.70072575226378,-7.513461999658));
#64972=CARTESIAN_POINT('Ctrl Pts',(41.5349397866914,4.69697099270009,-7.47034994575101));
#64973=CARTESIAN_POINT('Ctrl Pts',(41.470942430499,4.69063691665347,-7.39762224552403));
#64974=CARTESIAN_POINT('Ctrl Pts',(41.4034330822141,4.68430284060685,-7.32776149494582));
#64975=CARTESIAN_POINT('Ctrl Pts',(41.3326984783807,4.67796876456024,-7.26112547759101));
#64976=CARTESIAN_POINT('Ctrl Pts',(41.2620589909275,4.67164320590614,-7.1945790652727));
#64977=CARTESIAN_POINT('Ctrl Pts',(41.188203183454,4.66531764725203,-7.13124906469978));
#64978=CARTESIAN_POINT('Ctrl Pts',(41.1114571080781,4.65899208859793,-7.07145921638181));
#64979=CARTESIAN_POINT('Ctrl Pts',(41.034791305441,4.65267314617684,-7.01173190539693));
#64980=CARTESIAN_POINT('Ctrl Pts',(40.9552415880006,4.64635420375576,-6.95553765238175));
#64981=CARTESIAN_POINT('Ctrl Pts',(40.8731690713976,4.64003526133468,-6.9031617304993));
#64982=CARTESIAN_POINT('Ctrl Pts',(40.7911548182755,4.63372080474631,-6.85082299041221));
#64983=CARTESIAN_POINT('Ctrl Pts',(40.7066216939506,4.62740634815794,-6.80229742691731));
#64984=CARTESIAN_POINT('Ctrl Pts',(40.6199611695792,4.62109189156957,-6.75782799056738));
#64985=CARTESIAN_POINT('Ctrl Pts',(40.5333319751213,4.61477971781275,-6.71337463101373));
#64986=CARTESIAN_POINT('Ctrl Pts',(40.4445772973412,4.60846754405593,-6.67297468417212));
#64987=CARTESIAN_POINT('Ctrl Pts',(40.3541138485031,4.60215537029911,-6.636825511228));
#64988=CARTESIAN_POINT('Ctrl Pts',(40.2636586344952,4.59584377113545,-6.60067962892009));
#64989=CARTESIAN_POINT('Ctrl Pts',(40.1714953646493,4.58953217197179,-6.56878391315326));
#64990=CARTESIAN_POINT('Ctrl Pts',(40.0780604265547,4.58322057280813,-6.54128745683861));
#64991=CARTESIAN_POINT('Ctrl Pts',(39.9846087204924,4.57690784095586,-6.51378606597057));
#64992=CARTESIAN_POINT('Ctrl Pts',(39.8898853122176,4.57059510910359,-6.49068562596634));
#64993=CARTESIAN_POINT('Ctrl Pts',(39.794340414305,4.56428237725131,-6.47208497910214));
#64994=CARTESIAN_POINT('Ctrl Pts',(39.6986936174699,4.55796291285144,-6.45346449459184));
#64995=CARTESIAN_POINT('Ctrl Pts',(39.6022240115942,4.55164344845157,-6.43935346793963));
#64996=CARTESIAN_POINT('Ctrl Pts',(39.5053904357368,4.5453239840517,-6.4297993062387));
#64997=CARTESIAN_POINT('Ctrl Pts',(39.4085002460812,4.53900082497383,-6.42023955869238));
#64998=CARTESIAN_POINT('Ctrl Pts',(39.3112460990197,4.53267766589596,-6.41524200372406));
#64999=CARTESIAN_POINT('Ctrl Pts',(39.2140882719303,4.52635450681809,-6.4148019076763));
#65000=CARTESIAN_POINT('Ctrl Pts',(39.1167750937143,4.52002123728473,-6.41436110793415));
#65001=CARTESIAN_POINT('Ctrl Pts',(39.019558979423,4.51368796775138,-6.41849229985226));
#65002=CARTESIAN_POINT('Ctrl Pts',(38.9228964794896,4.50735469821802,-6.42713875523439));
#65003=CARTESIAN_POINT('Ctrl Pts',(38.8669867995618,4.50369152922538,-6.4321398730749));
#65004=CARTESIAN_POINT('Ctrl Pts',(38.811262184866,4.50002836023275,-6.43865059954992));
#65005=CARTESIAN_POINT('Ctrl Pts',(38.7558092127628,4.49636519124011,-6.44665219680531));
#65006=CARTESIAN_POINT('Ctrl Pts',(38.6599291495522,4.4900314482279,-6.46048722893314));
#65007=CARTESIAN_POINT('Ctrl Pts',(38.5645302463999,4.48369770521569,-6.47882995958531));
#65008=CARTESIAN_POINT('Ctrl Pts',(38.4700688058746,4.47736396220348,-6.50163579687419));
#65009=CARTESIAN_POINT('Ctrl Pts',(38.3757341241126,4.47103871850515,-6.5244110307791));
#65010=CARTESIAN_POINT('Ctrl Pts',(38.2823348259906,4.46471347480681,-6.55163736586205));
#65011=CARTESIAN_POINT('Ctrl Pts',(38.1903201893549,4.45838823110848,-6.58321868031024));
#65012=CARTESIAN_POINT('Ctrl Pts',(38.0984015320586,4.4520695851943,-6.6147670526765));
#65013=CARTESIAN_POINT('Ctrl Pts',(38.0078650761294,4.44575093928013,-6.65066123217911));
#65014=CARTESIAN_POINT('Ctrl Pts',(37.9191470452254,4.43943229336595,-6.69075471048375));
#65015=CARTESIAN_POINT('Ctrl Pts',(37.8304915911859,4.43311810428028,-6.73081990903357));
#65016=CARTESIAN_POINT('Ctrl Pts',(37.7436524094708,4.42680391519462,-6.7750783383247));
#65017=CARTESIAN_POINT('Ctrl Pts',(37.6590468694962,4.42048972610895,-6.82333493887741));
#65018=CARTESIAN_POINT('Ctrl Pts',(37.5744716754993,4.41417780177145,-6.87157423094508));
#65019=CARTESIAN_POINT('Ctrl Pts',(37.4921289106524,4.40786587743394,-6.92380862841624));
#65020=CARTESIAN_POINT('Ctrl Pts',(37.4124115565431,4.40155395309643,-6.97979701993741));
#65021=CARTESIAN_POINT('Ctrl Pts',(37.3327012260753,4.39524258488242,-7.03578047850027));
#65022=CARTESIAN_POINT('Ctrl Pts',(37.2556162040234,4.3889312166684,-7.09551702208044));
#65023=CARTESIAN_POINT('Ctrl Pts',(37.1815197986723,4.38261984845438,-7.15872268536673));
#65024=CARTESIAN_POINT('Ctrl Pts',(37.1074098738343,4.37630732868032,-7.22193988103615));
#65025=CARTESIAN_POINT('Ctrl Pts',(37.0362899812941,4.36999480890626,-7.28862716988691));
#65026=CARTESIAN_POINT('Ctrl Pts',(36.9684888985377,4.3636822891322,-7.35846154962566));
#65027=CARTESIAN_POINT('Ctrl Pts',(36.9006151772389,4.35736300645382,-7.42837074627515));
#65028=CARTESIAN_POINT('Ctrl Pts',(36.8360676692771,4.35104372377543,-7.50143345093607));
#65029=CARTESIAN_POINT('Ctrl Pts',(36.7751367898097,4.34472444109705,-7.57729132959634));
#65030=CARTESIAN_POINT('Ctrl Pts',(36.7141701232154,4.33840144685282,-7.65319376260332));
#65031=CARTESIAN_POINT('Ctrl Pts',(36.6568245722978,4.3320784526086,-7.73189428560719));
#65032=CARTESIAN_POINT('Ctrl Pts',(36.6033476688481,4.32575545836437,-7.81300487032726));
#65033=CARTESIAN_POINT('Ctrl Pts',(36.5497850149696,4.31942232517357,-7.89424551619452));
#65034=CARTESIAN_POINT('Ctrl Pts',(36.5001036187132,4.31308919198277,-7.97790356498957));
#65035=CARTESIAN_POINT('Ctrl Pts',(36.4545054296171,4.30675605879197,-8.06356569874036));
#65036=CARTESIAN_POINT('Ctrl Pts',(36.4281136380704,4.30309050245469,-8.11314611459069));
#65037=CARTESIAN_POINT('Ctrl Pts',(36.4030888281374,4.29942494611741,-8.16339749101763));
#65038=CARTESIAN_POINT('Ctrl Pts',(36.3794626743309,4.29575938978012,-8.21423692171043));
#65039=CARTESIAN_POINT('Ctrl Pts',(36.3352160404628,4.288894602117,-8.30944808872224));
#65040=CARTESIAN_POINT('Ctrl Pts',(36.2957430807869,4.28202981445388,-8.40701169084998));
#65041=CARTESIAN_POINT('Ctrl Pts',(36.2612786271195,4.27516502679075,-8.50644840804449));
#65042=CARTESIAN_POINT('Ctrl Pts',(36.2269374637337,4.26832479665038,-8.60552940856349));
#65043=CARTESIAN_POINT('Ctrl Pts',(36.1975691938129,4.26148456651002,-8.70646986597188));
#65044=CARTESIAN_POINT('Ctrl Pts',(36.1733603994216,4.25464433636965,-8.80877141839319));
#65045=CARTESIAN_POINT('Ctrl Pts',(36.1492076389944,4.24781993870753,-8.91083618242152));
#65046=CARTESIAN_POINT('Ctrl Pts',(36.1301906402494,4.2409955410454,-9.01425545804629));
#65047=CARTESIAN_POINT('Ctrl Pts',(36.1164468242244,4.23417114338327,-9.11851449587413));
#65048=CARTESIAN_POINT('Ctrl Pts',(36.1027487584133,4.22736946267633,-9.22242647774091));
#65049=CARTESIAN_POINT('Ctrl Pts',(36.0942889360373,4.22056778196938,-9.3271723358877));
#65050=CARTESIAN_POINT('Ctrl Pts',(36.0911539354075,4.21376610126243,-9.43222716147583));
#65051=CARTESIAN_POINT('Ctrl Pts',(36.0902419066779,4.21178736857714,-9.46278952188274));
#65052=CARTESIAN_POINT('Ctrl Pts',(36.0897802097724,4.20980863589185,-9.493377948687));
#65053=CARTESIAN_POINT('Ctrl Pts',(36.0897701674737,4.20782990320657,-9.52397933185991));
#65054=CARTESIAN_POINT('',(36.0897712272353,2.93782984291316,-9.52776296339717));
#65055=CARTESIAN_POINT('Ctrl Pts',(36.0944248666917,4.20782984291316,-9.5239817904194));
#65056=CARTESIAN_POINT('Ctrl Pts',(36.0961127382952,4.17027109138215,-10.1039645708521));
#65057=CARTESIAN_POINT('Ctrl Pts',(36.529553577299,4.0658437393645,-11.7188971193403));
#65058=CARTESIAN_POINT('Ctrl Pts',(39.123431789966,3.89454778686015,-13.194039457166));
#65059=CARTESIAN_POINT('Ctrl Pts',(42.230539573114,3.69394198540018,-11.5947102098393));
#65060=CARTESIAN_POINT('Ctrl Pts',(42.5896834516285,3.49333618394021,-8.11861111471374));
#65061=CARTESIAN_POINT('Ctrl Pts',(39.8751829600439,3.29273038248021,-5.91779011158274));
#65062=CARTESIAN_POINT('Ctrl Pts',(36.8044545844578,3.10756161888526,-6.9054988491143));
#65063=CARTESIAN_POINT('Ctrl Pts',(36.0968354029096,2.98926145577694,-8.73662212930356));
#65064=CARTESIAN_POINT('Ctrl Pts',(36.0896823919881,2.9378298931553,-9.52776226947597));
#65065=CARTESIAN_POINT('',(36.0897704721981,1.66782984286977,-9.52328614782123));
#65066=CARTESIAN_POINT('Ctrl Pts',(36.0897712272353,2.93782984291316,-9.52776296339717));
#65067=CARTESIAN_POINT('Ctrl Pts',(36.0898865823914,2.92938781562177,-9.657616629196));
#65068=CARTESIAN_POINT('Ctrl Pts',(36.0981377832265,2.92094578833037,-9.78711742420437));
#65069=CARTESIAN_POINT('Ctrl Pts',(36.114371081634,2.91250376103898,-9.91541622794557));
#65070=CARTESIAN_POINT('Ctrl Pts',(36.1278218581146,2.90550876721274,-10.0217235530829));
#65071=CARTESIAN_POINT('Ctrl Pts',(36.1467519556812,2.8985137733865,-10.1272063727662));
#65072=CARTESIAN_POINT('Ctrl Pts',(36.1710500170942,2.89151877956026,-10.2313941208384));
#65073=CARTESIAN_POINT('Ctrl Pts',(36.19304725805,2.88518615235742,-10.3257161722989));
#65074=CARTESIAN_POINT('Ctrl Pts',(36.2194927104237,2.87885352515457,-10.4191735792048));
#65075=CARTESIAN_POINT('Ctrl Pts',(36.2503030538065,2.87252089795173,-10.5113156586593));
#65076=CARTESIAN_POINT('Ctrl Pts',(36.2810719318078,2.86619679336739,-10.603333730847));
#65077=CARTESIAN_POINT('Ctrl Pts',(36.3161938876909,2.85987268878306,-10.6940395827062));
#65078=CARTESIAN_POINT('Ctrl Pts',(36.3555348578463,2.85354858419872,-10.7829939220729));
#65079=CARTESIAN_POINT('Ctrl Pts',(36.394834650207,2.84723109899053,-10.8718551538345));
#65080=CARTESIAN_POINT('Ctrl Pts',(36.4383445016696,2.84091361378234,-10.9589681199301));
#65081=CARTESIAN_POINT('Ctrl Pts',(36.4858812591661,2.83459612857415,-11.0439108313374));
#65082=CARTESIAN_POINT('Ctrl Pts',(36.5333842740557,2.82828312765204,-11.128793248592));
#65083=CARTESIAN_POINT('Ctrl Pts',(36.584908299381,2.82197012672992,-11.2115080932165));
#65084=CARTESIAN_POINT('Ctrl Pts',(36.6402234176746,2.8156571258078,-11.2916563054195));
#65085=CARTESIAN_POINT('Ctrl Pts',(36.6955185471165,2.8093464061723,-11.3717755550029));
#65086=CARTESIAN_POINT('Ctrl Pts',(36.7546017992502,2.80303568653681,-11.4493296555402));
#65087=CARTESIAN_POINT('Ctrl Pts',(36.8171994548306,2.79672496690131,-11.5239477769167));
#65088=CARTESIAN_POINT('Ctrl Pts',(36.8797914444659,2.79041481847235,-11.5985591443314));
#65089=CARTESIAN_POINT('Ctrl Pts',(36.9458969238692,2.78410467004339,-11.6702347260536));
#65090=CARTESIAN_POINT('Ctrl Pts',(37.0152020108701,2.77779452161443,-11.7386369168394));
#65091=CARTESIAN_POINT('Ctrl Pts',(37.0845195957786,2.77148323526536,-11.8070514427118));
#65092=CARTESIAN_POINT('Ctrl Pts',(37.1570376229935,2.7651719489163,-11.8721910980819));
#65093=CARTESIAN_POINT('Ctrl Pts',(37.2324062670082,2.75886066256724,-11.9337560181121));
#65094=CARTESIAN_POINT('Ctrl Pts',(37.3078555124955,2.75254262674058,-11.9953867775014));
#65095=CARTESIAN_POINT('Ctrl Pts',(37.3861611217752,2.74622459091391,-12.0534348921755));
#65096=CARTESIAN_POINT('Ctrl Pts',(37.4669413473052,2.73990655508725,-12.1076417403929));
#65097=CARTESIAN_POINT('Ctrl Pts',(37.5477689074287,2.73358481709641,-12.1618803520661));
#65098=CARTESIAN_POINT('Ctrl Pts',(37.631073597226,2.72726307910557,-12.2122729889631));
#65099=CARTESIAN_POINT('Ctrl Pts',(37.7164477520338,2.72094134111473,-12.2586062958031));
#65100=CARTESIAN_POINT('Ctrl Pts',(37.8019587970218,2.71460946675586,-12.3050138941514));
#65101=CARTESIAN_POINT('Ctrl Pts',(37.889545539423,2.708277592397,-12.3473489753417));
#65102=CARTESIAN_POINT('Ctrl Pts',(37.9787790179551,2.70194571803814,-12.3854457634979));
#65103=CARTESIAN_POINT('Ctrl Pts',(38.0306062077465,2.69826813805885,-12.4075725426249));
#65104=CARTESIAN_POINT('Ctrl Pts',(38.0829885683538,2.69459055807955,-12.4282705229668));
#65105=CARTESIAN_POINT('Ctrl Pts',(38.1358399153893,2.69091297810026,-12.447515007185));
#65106=CARTESIAN_POINT('Ctrl Pts',(38.2268474624822,2.6845803574212,-12.4806531087094));
#65107=CARTESIAN_POINT('Ctrl Pts',(38.3195624478393,2.67824773674214,-12.5095937395124));
#65108=CARTESIAN_POINT('Ctrl Pts',(38.4135619344936,2.67191511606308,-12.5341603184315));
#65109=CARTESIAN_POINT('Ctrl Pts',(38.5074349132907,2.66559101805048,-12.5586938347737));
#65110=CARTESIAN_POINT('Ctrl Pts',(38.6025885379292,2.65926692003788,-12.5788648897886));
#65111=CARTESIAN_POINT('Ctrl Pts',(38.6985816725519,2.65294282202529,-12.5945456200876));
#65112=CARTESIAN_POINT('Ctrl Pts',(38.7944743314453,2.64662534342732,-12.6102099374127));
#65113=CARTESIAN_POINT('Ctrl Pts',(38.8912043240746,2.64030786482936,-12.6213932037357));
#65114=CARTESIAN_POINT('Ctrl Pts',(38.9883181706112,2.63399038623139,-12.6280181204767));
#65115=CARTESIAN_POINT('Ctrl Pts',(39.085363083138,2.62767739194897,-12.6346383346743));
#65116=CARTESIAN_POINT('Ctrl Pts',(39.1827908728243,2.62136439766654,-12.6367066022538));
#65117=CARTESIAN_POINT('Ctrl Pts',(39.2801416979861,2.61505140338411,-12.6341973178208));
#65118=CARTESIAN_POINT('Ctrl Pts',(39.3774573438581,2.60874069040392,-12.6316889401581));
#65119=CARTESIAN_POINT('Ctrl Pts',(39.4746956437448,2.60242997742373,-12.6246063085977));
#65120=CARTESIAN_POINT('Ctrl Pts',(39.5713964520392,2.59611926444353,-12.6129759274179));
#65121=CARTESIAN_POINT('Ctrl Pts',(39.6680885074651,2.58980912267719,-12.6013465989615));
#65122=CARTESIAN_POINT('Ctrl Pts',(39.7642427338712,2.58349898091085,-12.5851703917463));
#65123=CARTESIAN_POINT('Ctrl Pts',(39.8594048536913,2.57718883914451,-12.5645256030881));
#65124=CARTESIAN_POINT('Ctrl Pts',(39.9545841342963,2.57087755945706,-12.5438770915119));
#65125=CARTESIAN_POINT('Ctrl Pts',(40.0487705256217,2.5645662797696,-12.5187584907639));
#65126=CARTESIAN_POINT('Ctrl Pts',(40.1415217058894,2.55825500008215,-12.4892988260698));
#65127=CARTESIAN_POINT('Ctrl Pts',(40.2343720777595,2.55193697087471,-12.4598076561018));
#65128=CARTESIAN_POINT('Ctrl Pts',(40.3257837568097,2.54561894166727,-12.425966286297));
#65129=CARTESIAN_POINT('Ctrl Pts',(40.4153315082647,2.53930091245983,-12.3879530170645));
#65130=CARTESIAN_POINT('Ctrl Pts',(40.5049317320566,2.53297918107393,-12.3499174731793));
#65131=CARTESIAN_POINT('Ctrl Pts',(40.5926654594737,2.52665744968802,-12.3077053515008));
#65132=CARTESIAN_POINT('Ctrl Pts',(40.6781311942546,2.52033571830212,-12.2615413984574));
#65133=CARTESIAN_POINT('Ctrl Pts',(40.763733967387,2.51400385046037,-12.2153034247316));
#65134=CARTESIAN_POINT('Ctrl Pts',(40.8470611119474,2.50767198261862,-12.1651011923231));
#65135=CARTESIAN_POINT('Ctrl Pts',(40.9277393326589,2.50134011477686,-12.1112032888548));
#65136=CARTESIAN_POINT('Ctrl Pts',(40.9745984817717,2.49766246873134,-12.0798985591122));
#65137=CARTESIAN_POINT('Ctrl Pts',(41.0205646165812,2.49398482268582,-12.0473478859908));
#65138=CARTESIAN_POINT('Ctrl Pts',(41.0655699423,2.49030717664029,-12.013609941973));
#65139=CARTESIAN_POINT('Ctrl Pts',(41.1430655829285,2.48397455862786,-11.9555158488098));
#65140=CARTESIAN_POINT('Ctrl Pts',(41.2179796614594,2.47764194061542,-11.893697564131));
#65141=CARTESIAN_POINT('Ctrl Pts',(41.2899331267851,2.47130932260298,-11.8284127242999));
#65142=CARTESIAN_POINT('Ctrl Pts',(41.3617897538102,2.46498522732066,-11.7632157478247));
#65143=CARTESIAN_POINT('Ctrl Pts',(41.4306933659334,2.45866113203834,-11.6945617803698));
#65144=CARTESIAN_POINT('Ctrl Pts',(41.4962957594979,2.45233703675603,-11.6227503278064));
#65145=CARTESIAN_POINT('Ctrl Pts',(41.5618294865846,2.44601956094786,-11.5510140407858));
#65146=CARTESIAN_POINT('Ctrl Pts',(41.6240685712259,2.4397020851397,-11.4761271602531));
#65147=CARTESIAN_POINT('Ctrl Pts',(41.6827004043077,2.43338460933153,-11.3984271684137));
#65148=CARTESIAN_POINT('Ctrl Pts',(41.7412906182062,2.42707161791641,-11.3207823310873));
#65149=CARTESIAN_POINT('Ctrl Pts',(41.7962784084439,2.42075862650128,-11.2403287004153));
#65150=CARTESIAN_POINT('Ctrl Pts',(41.8473909752809,2.41444563508615,-11.157437342412));
#65151=CARTESIAN_POINT('Ctrl Pts',(41.8984850713801,2.40813492502014,-11.0745759391662));
#65152=CARTESIAN_POINT('Ctrl Pts',(41.9457064974003,2.40182421495412,-10.989278930866));
#65153=CARTESIAN_POINT('Ctrl Pts',(41.9888259231194,2.39551350488811,-10.9019461221984));
#65154=CARTESIAN_POINT('Ctrl Pts',(42.0319414455877,2.38920336607934,-10.8146212190596));
#65155=CARTESIAN_POINT('Ctrl Pts',(42.0709555126086,2.38289322727057,-10.7252612741663));
#65156=CARTESIAN_POINT('Ctrl Pts',(42.1056853720536,2.3765830884618,-10.6342894895083));
#65157=CARTESIAN_POINT('Ctrl Pts',(42.1404214941901,2.37027181177188,-10.5433013002859));
#65158=CARTESIAN_POINT('Ctrl Pts',(42.1708717184259,2.36396053508196,-10.4507011025792));
#65159=CARTESIAN_POINT('Ctrl Pts',(42.1969023064928,2.35764925839203,-10.3569298156925));
#65160=CARTESIAN_POINT('Ctrl Pts',(42.2229607324854,2.35133123222525,-10.2630582468561));
#65161=CARTESIAN_POINT('Ctrl Pts',(42.2445899689501,2.34501320605846,-10.1680135105659));
#65162=CARTESIAN_POINT('Ctrl Pts',(42.2617068798173,2.33869517989168,-10.0722491525615));
#65163=CARTESIAN_POINT('Ctrl Pts',(42.2788338206155,2.33237345157523,-9.97642867988201));
#65164=CARTESIAN_POINT('Ctrl Pts',(42.2914431141386,2.32605172325879,-9.87988817925913));
#65165=CARTESIAN_POINT('Ctrl Pts',(42.2995034932724,2.31972999494234,-9.78308670653901));
#65166=CARTESIAN_POINT('Ctrl Pts',(42.307576796649,2.31339813018564,-9.68613001956475));
#65167=CARTESIAN_POINT('Ctrl Pts',(42.3110866053107,2.30706626542893,-9.58891196167446));
#65168=CARTESIAN_POINT('Ctrl Pts',(42.3100537791399,2.30073440067222,-9.49189193818005));
#65169=CARTESIAN_POINT('Ctrl Pts',(42.3094538928027,2.29705672550825,-9.43554074551828));
#65170=CARTESIAN_POINT('Ctrl Pts',(42.3073225134909,2.29337905034427,-9.37925629083746));
#65171=CARTESIAN_POINT('Ctrl Pts',(42.3036717148399,2.2897013751803,-9.32312741790204));
#65172=CARTESIAN_POINT('Ctrl Pts',(42.2973853725387,2.28336875397506,-9.22647861801376));
#65173=CARTESIAN_POINT('Ctrl Pts',(42.2865693255086,2.27703613276983,-9.1299558590541));
#65174=CARTESIAN_POINT('Ctrl Pts',(42.2712321176497,2.27070351156459,-9.0340173807386));
#65175=CARTESIAN_POINT('Ctrl Pts',(42.2559155511875,2.26437941304139,-8.93820802006958));
#65176=CARTESIAN_POINT('Ctrl Pts',(42.2360899860721,2.25805531451819,-8.84298180532608));
#65177=CARTESIAN_POINT('Ctrl Pts',(42.2118158887524,2.25173121599499,-8.74879403174244));
#65178=CARTESIAN_POINT('Ctrl Pts',(42.1875671991186,2.24541373690265,-8.65470484445572));
#65179=CARTESIAN_POINT('Ctrl Pts',(42.1588793427473,2.23909625781031,-8.56165235869884));
#65180=CARTESIAN_POINT('Ctrl Pts',(42.1258640434083,2.23277877871797,-8.47008282202319));
#65181=CARTESIAN_POINT('Ctrl Pts',(42.0928721793498,2.22646578396769,-8.37857828423685));
#65182=CARTESIAN_POINT('Ctrl Pts',(42.0555591270576,2.2201527892174,-8.28855501303765));
#65183=CARTESIAN_POINT('Ctrl Pts',(42.0140864933062,2.21383979446712,-8.20044427784569));
#65184=CARTESIAN_POINT('Ctrl Pts',(41.9726288464674,2.20752908103568,-8.11236538311758));
#65185=CARTESIAN_POINT('Ctrl Pts',(41.92701479098,2.20121836760425,-8.02619804638502));
#65186=CARTESIAN_POINT('Ctrl Pts',(41.8774537600952,2.19490765417281,-7.9423528455615));
#65187=CARTESIAN_POINT('Ctrl Pts',(41.8278972153596,2.18859751197247,-7.85851523421045));
#65188=CARTESIAN_POINT('Ctrl Pts',(41.7743946282699,2.18228736977213,-7.77699971720841));
#65189=CARTESIAN_POINT('Ctrl Pts',(41.7172004849958,2.17597722757179,-7.69819065821384));
#65190=CARTESIAN_POINT('Ctrl Pts',(41.6599960279446,2.16966594746824,-7.61936738764078));
#65191=CARTESIAN_POINT('Ctrl Pts',(41.5990989494367,2.1633546673647,-7.54325189831572));
#65192=CARTESIAN_POINT('Ctrl Pts',(41.5348053636789,2.15704338726115,-7.47019719519463));
#65193=CARTESIAN_POINT('Ctrl Pts',(41.4704430202524,2.15072535766771,-7.39706436497859));
#65194=CARTESIAN_POINT('Ctrl Pts',(41.4026772072064,2.14440732807428,-7.32699918476624));
#65195=CARTESIAN_POINT('Ctrl Pts',(41.3318422719954,2.13808929848084,-7.26031918800166));
#65196=CARTESIAN_POINT('Ctrl Pts',(41.2609658297919,2.13176756672539,-7.19360011890483));
#65197=CARTESIAN_POINT('Ctrl Pts',(41.1870170163125,2.12544583496994,-7.13027046749327));
#65198=CARTESIAN_POINT('Ctrl Pts',(41.1103631456135,2.11912410321448,-7.07060734502775));
#65199=CARTESIAN_POINT('Ctrl Pts',(41.0335863661418,2.11279223503299,-7.01084855718895));
#65200=CARTESIAN_POINT('Ctrl Pts',(40.9540962256173,2.10646036685149,-6.95476828958038));
#65201=CARTESIAN_POINT('Ctrl Pts',(40.8722888243246,2.10012849867,-6.90260019429931));
#65202=CARTESIAN_POINT('Ctrl Pts',(40.8247738891365,2.09645085702011,-6.87230020154806));
#65203=CARTESIAN_POINT('Ctrl Pts',(40.7764777108262,2.09277321537021,-6.84331910900542));
#65204=CARTESIAN_POINT('Ctrl Pts',(40.7274812829116,2.08909557372032,-6.81569536905595));
#65205=CARTESIAN_POINT('Ctrl Pts',(40.6431131484773,2.08276295360239,-6.76812938302743));
#65206=CARTESIAN_POINT('Ctrl Pts',(40.5563745365518,2.07643033348445,-6.72442538258168));
#65207=CARTESIAN_POINT('Ctrl Pts',(40.4676538386611,2.07009771336651,-6.68482669574058));
#65208=CARTESIAN_POINT('Ctrl Pts',(40.3790525446178,2.06377361594085,-6.64528130238878));
#65209=CARTESIAN_POINT('Ctrl Pts',(40.2884748624991,2.05744951851519,-6.60983041799162));
#65210=CARTESIAN_POINT('Ctrl Pts',(40.1963351000381,2.05112542108953,-6.57867228208874));
#65211=CARTESIAN_POINT('Ctrl Pts',(40.1042917803644,2.04480794310337,-6.54754675943986));
#65212=CARTESIAN_POINT('Ctrl Pts',(40.0106900429605,2.03849046511721,-6.52070519189233));
#65213=CARTESIAN_POINT('Ctrl Pts',(39.9159646374313,2.03217298713105,-6.49829795142503));
#65214=CARTESIAN_POINT('Ctrl Pts',(39.82130647106,2.02585999349519,-6.47590661634208));
#65215=CARTESIAN_POINT('Ctrl Pts',(39.7255266466333,2.01954699985933,-6.45794345104749));
#65216=CARTESIAN_POINT('Ctrl Pts',(39.6290746383508,2.01323400622348,-6.44450886908854));
#65217=CARTESIAN_POINT('Ctrl Pts',(39.5326574848847,2.00692329391114,-6.43107914197811));
#65218=CARTESIAN_POINT('Ctrl Pts',(39.4355690629136,2.0006125815988,-6.42217480674485));
#65219=CARTESIAN_POINT('Ctrl Pts',(39.3382676628183,1.99430186928646,-6.41784491756225));
#65220=CARTESIAN_POINT('Ctrl Pts',(39.2409750702715,1.98799172820849,-6.41351542031346));
#65221=CARTESIAN_POINT('Ctrl Pts',(39.1434699748185,1.98168158713053,-6.41375956508012));
#65222=CARTESIAN_POINT('Ctrl Pts',(39.0462133422926,1.97537144605256,-6.41857435034875));
#65223=CARTESIAN_POINT('Ctrl Pts',(38.9489391715773,1.96906016707328,-6.4233900038627));
#65224=CARTESIAN_POINT('Ctrl Pts',(38.851913989548,1.962748888094,-6.43277791322323));
#65225=CARTESIAN_POINT('Ctrl Pts',(38.7555952575182,1.95643760911472,-6.44668307710858));
#65226=CARTESIAN_POINT('Ctrl Pts',(38.659173518999,1.95011958064156,-6.46060311164357));
#65227=CARTESIAN_POINT('Ctrl Pts',(38.5634601723352,1.94380155216841,-6.47904998274993));
#65228=CARTESIAN_POINT('Ctrl Pts',(38.468903874672,1.93748352369525,-6.50191728389209));
#65229=CARTESIAN_POINT('Ctrl Pts',(38.3742921700424,1.93116179305946,-6.5247979845414));
#65230=CARTESIAN_POINT('Ctrl Pts',(38.2808392840599,1.92484006242367,-6.5521041504863));
#65231=CARTESIAN_POINT('Ctrl Pts',(38.1889780452493,1.91851833178789,-6.58367967403887));
#65232=CARTESIAN_POINT('Ctrl Pts',(38.0969695135832,1.91218646471404,-6.61530582666079));
#65233=CARTESIAN_POINT('Ctrl Pts',(38.0065581313407,1.90585459764019,-6.65121484504372));
#65234=CARTESIAN_POINT('Ctrl Pts',(37.9181560702437,1.89952273056634,-6.69120276084421));
#65235=CARTESIAN_POINT('Ctrl Pts',(37.8668106959715,1.89584507779768,-6.71442840148728));
#65236=CARTESIAN_POINT('Ctrl Pts',(37.8161427060572,1.89216742502901,-6.73902918483806));
#65237=CARTESIAN_POINT('Ctrl Pts',(37.7662285731077,1.88848977226034,-6.76495830677739));
#65238=CARTESIAN_POINT('Ctrl Pts',(37.6802804830955,1.88215715236861,-6.80960615248134));
#65239=CARTESIAN_POINT('Ctrl Pts',(37.5962706002101,1.87582453247687,-6.85835002622903));
#65240=CARTESIAN_POINT('Ctrl Pts',(37.5146149849758,1.86949191258514,-6.91099770389696));
#65241=CARTESIAN_POINT('Ctrl Pts',(37.4330692652116,1.86316781539252,-6.96357452616485));
#65242=CARTESIAN_POINT('Ctrl Pts',(37.3538718800542,1.85684371819989,-7.02004447501155));
#65243=CARTESIAN_POINT('Ctrl Pts',(37.2774153000616,1.85051962100727,-7.08016897834167));
#65244=CARTESIAN_POINT('Ctrl Pts',(37.201038747334,1.84420214326063,-7.14023054922626));
#65245=CARTESIAN_POINT('Ctrl Pts',(37.1273976383947,1.83788466551399,-7.20393880094852));
#65246=CARTESIAN_POINT('Ctrl Pts',(37.0568555343101,1.83156718776735,-7.27101187845124));
#65247=CARTESIAN_POINT('Ctrl Pts',(36.9863635033928,1.82525419437972,-7.33803734521896));
#65248=CARTESIAN_POINT('Ctrl Pts',(36.9189664200622,1.81894120099208,-7.40842258887038));
#65249=CARTESIAN_POINT('Ctrl Pts',(36.8549940598641,1.81262820760444,-7.48184611601883));
#65250=CARTESIAN_POINT('Ctrl Pts',(36.7910448173821,1.80631749554562,-7.55524311007945));
#65251=CARTESIAN_POINT('Ctrl Pts',(36.7305181259069,1.80000678348679,-7.6316758766227));
#65252=CARTESIAN_POINT('Ctrl Pts',(36.67370557269,1.79369607142797,-7.71078746574647));
#65253=CARTESIAN_POINT('Ctrl Pts',(36.6168981620889,1.78738593060851,-7.789891893768));
#65254=CARTESIAN_POINT('Ctrl Pts',(36.5638044762192,1.78107578978905,-7.87167430692623));
#65255=CARTESIAN_POINT('Ctrl Pts',(36.5146739743187,1.7747656489696,-7.95574706031865));
#65256=CARTESIAN_POINT('Ctrl Pts',(36.465534612801,1.76845437025352,-8.03983497440311));
#65257=CARTESIAN_POINT('Ctrl Pts',(36.4203600752962,1.76214309153745,-8.12621367143539));
#65258=CARTESIAN_POINT('Ctrl Pts',(36.3793543617298,1.75583181282138,-8.2144700170514));
#65259=CARTESIAN_POINT('Ctrl Pts',(36.3383047953098,1.74951378461706,-8.3028207468951));
#65260=CARTESIAN_POINT('Ctrl Pts',(36.3014331381041,1.74319575641274,-8.39305273697286));
#65261=CARTESIAN_POINT('Ctrl Pts',(36.2688955317398,1.73687772820842,-8.48473212630355));
#65262=CARTESIAN_POINT('Ctrl Pts',(36.2363388593963,1.73055599784504,-8.5764652367749));
#65263=CARTESIAN_POINT('Ctrl Pts',(36.2081214216448,1.72423426748166,-8.66964701699669));
#65264=CARTESIAN_POINT('Ctrl Pts',(36.1843490890647,1.71791253711828,-8.76382969298902));
#65265=CARTESIAN_POINT('Ctrl Pts',(36.1605386392775,1.71158067031984,-8.85816338405539));
#65266=CARTESIAN_POINT('Ctrl Pts',(36.1411876137695,1.7052488035214,-8.95350074722008));
#65267=CARTESIAN_POINT('Ctrl Pts',(36.1263505140941,1.69891693672297,-9.04938514458597));
#65268=CARTESIAN_POINT('Ctrl Pts',(36.1177328757093,1.69523928141543,-9.10507642396817));
#65269=CARTESIAN_POINT('Ctrl Pts',(36.1106370296069,1.69156162610789,-9.16095215353144));
#65270=CARTESIAN_POINT('Ctrl Pts',(36.1050655842624,1.68788397080035,-9.21692271232171));
#65271=CARTESIAN_POINT('Ctrl Pts',(36.0949386176573,1.68119926150462,-9.3186578895869));
#65272=CARTESIAN_POINT('Ctrl Pts',(36.0898268905567,1.67451455220889,-9.42090043518689));
#65273=CARTESIAN_POINT('Ctrl Pts',(36.0897704721985,1.66782984291316,-9.52328614715663));
#65274=CARTESIAN_POINT('',(36.08977020096,0.397829842977112,-9.52388193753632));
#65275=CARTESIAN_POINT('Ctrl Pts',(36.0897704721981,1.66782984286977,-9.52328614782123));
#65276=CARTESIAN_POINT('Ctrl Pts',(36.0897177166195,1.66157911429467,-9.61902483550123));
#65277=CARTESIAN_POINT('Ctrl Pts',(36.094089700507,1.65532838571958,-9.71493781111452));
#65278=CARTESIAN_POINT('Ctrl Pts',(36.1029083362522,1.64907765714449,-9.8105763982615));
#65279=CARTESIAN_POINT('Ctrl Pts',(36.1117161895845,1.64283457124101,-9.90609804954951));
#65280=CARTESIAN_POINT('Ctrl Pts',(36.1249598533129,1.63659148533753,-10.0013455349007));
#65281=CARTESIAN_POINT('Ctrl Pts',(36.1426092124648,1.63034839943405,-10.0958697094739));
#65282=CARTESIAN_POINT('Ctrl Pts',(36.1602423302137,1.6241110585819,-10.1903069004235));
#65283=CARTESIAN_POINT('Ctrl Pts',(36.1822730039185,1.61787371772975,-10.2840216636972));
#65284=CARTESIAN_POINT('Ctrl Pts',(36.2086193831783,1.61163637687759,-10.3765707006487));
#65285=CARTESIAN_POINT('Ctrl Pts',(36.2349529388969,1.60540207191878,-10.4690746913199));
#65286=CARTESIAN_POINT('Ctrl Pts',(36.2655979066875,1.59916776695996,-10.5604136509191));
#65287=CARTESIAN_POINT('Ctrl Pts',(36.3004217192847,1.59293346200114,-10.650156187782));
#65288=CARTESIAN_POINT('Ctrl Pts',(36.3352385865237,1.58670040042946,-10.7398808261434));
#65289=CARTESIAN_POINT('Ctrl Pts',(36.374232480264,1.58046733885778,-10.8280092555743));
#65290=CARTESIAN_POINT('Ctrl Pts',(36.4172219193474,1.5742342772861,-10.9141280742752));
#65291=CARTESIAN_POINT('Ctrl Pts',(36.4602151348599,1.56800066816797,-11.0002544581274));
#65292=CARTESIAN_POINT('Ctrl Pts',(36.5072043906412,1.56176705904983,-11.0843704793567));
#65293=CARTESIAN_POINT('Ctrl Pts',(36.5579618411616,1.5555334499317,-11.1660865364574));
#65294=CARTESIAN_POINT('Ctrl Pts',(36.6087696800298,1.54929365253459,-11.2478837153848));
#65295=CARTESIAN_POINT('Ctrl Pts',(36.6633529439873,1.54305385513747,-11.327275791583));
#65296=CARTESIAN_POINT('Ctrl Pts',(36.7214401637571,1.53681405774035,-11.4039017513068));
#65297=CARTESIAN_POINT('Ctrl Pts',(36.7795583433284,1.53057093460498,-11.4805685517613));
#65298=CARTESIAN_POINT('Ctrl Pts',(36.8411839074336,1.52432781146962,-11.5544659570656));
#65299=CARTESIAN_POINT('Ctrl Pts',(36.906006215445,1.51808468833425,-11.6252674042424));
#65300=CARTESIAN_POINT('Ctrl Pts',(36.9709326194122,1.51183153957822,-11.6961825490727));
#65301=CARTESIAN_POINT('Ctrl Pts',(37.0390656975799,1.50557839082219,-11.7639914937854));
#65302=CARTESIAN_POINT('Ctrl Pts',(37.1100593558897,1.49932524206616,-11.8284059036557));
#65303=CARTESIAN_POINT('Ctrl Pts',(37.1556505611154,1.49530955115757,-11.8697720009918));
#65304=CARTESIAN_POINT('Ctrl Pts',(37.2024208073046,1.49129386024897,-11.9097389989716));
#65305=CARTESIAN_POINT('Ctrl Pts',(37.2502721211606,1.48727816934038,-11.9482399491954));
#65306=CARTESIAN_POINT('Ctrl Pts',(37.3257321603814,1.48094554920851,-12.0089547547003));
#65307=CARTESIAN_POINT('Ctrl Pts',(37.4041619730563,1.47461292907664,-12.0662469089251));
#65308=CARTESIAN_POINT('Ctrl Pts',(37.4852181569681,1.46828030894477,-12.1198128802879));
#65309=CARTESIAN_POINT('Ctrl Pts',(37.5661652522127,1.46195621150737,-12.1733067604155));
#65310=CARTESIAN_POINT('Ctrl Pts',(37.6497313315992,1.45563211406997,-12.2230841858521));
#65311=CARTESIAN_POINT('Ctrl Pts',(37.735540056303,1.44930801663257,-12.2688818717662));
#65312=CARTESIAN_POINT('Ctrl Pts',(37.8212589648937,1.44299053863687,-12.3146316211778));
#65313=CARTESIAN_POINT('Ctrl Pts',(37.9092154683211,1.43667306064118,-12.3564097076499));
#65314=CARTESIAN_POINT('Ctrl Pts',(37.9990052376984,1.43035558264549,-12.39399672949));
#65315=CARTESIAN_POINT('Ctrl Pts',(38.0887312713447,1.42404258900342,-12.4315570708259));
#65316=CARTESIAN_POINT('Ctrl Pts',(38.1802875816035,1.41772959536135,-12.4649320935326));
#65317=CARTESIAN_POINT('Ctrl Pts',(38.2732471482195,1.41141660171928,-12.4939492761947));
#65318=CARTESIAN_POINT('Ctrl Pts',(38.3661731220506,1.4051058894028,-12.5229559729216));
#65319=CARTESIAN_POINT('Ctrl Pts',(38.4605009276115,1.39879517708631,-12.5476078285589));
#65320=CARTESIAN_POINT('Ctrl Pts',(38.5557864532949,1.39248446476983,-12.5677815496913));
#65321=CARTESIAN_POINT('Ctrl Pts',(38.6510633538717,1.38617432368981,-12.5879534447279));
#65322=CARTESIAN_POINT('Ctrl Pts',(38.7472973743376,1.37986418260979,-12.603647920822));
#65323=CARTESIAN_POINT('Ctrl Pts',(38.8440332560997,1.37355404152977,-12.6147926030944));
#65324=CARTESIAN_POINT('Ctrl Pts',(38.9407865821129,1.36724276255051,-12.6259392950724));
#65325=CARTESIAN_POINT('Ctrl Pts',(39.038041514729,1.36093148357126,-12.6325345136804));
#65326=CARTESIAN_POINT('Ctrl Pts',(39.1353377543829,1.354620204592,-12.6345577574459));
#65327=CARTESIAN_POINT('Ctrl Pts',(39.2327380458558,1.34830217612211,-12.6365831649352));
#65328=CARTESIAN_POINT('Ctrl Pts',(39.3301792946209,1.34198414765222,-12.6340268270135));
#65329=CARTESIAN_POINT('Ctrl Pts',(39.4272014857098,1.33566611918233,-12.6269203951409));
#65330=CARTESIAN_POINT('Ctrl Pts',(39.524280528672,1.32934438855162,-12.6198097991286));
#65331=CARTESIAN_POINT('Ctrl Pts',(39.6209395910218,1.32302265792092,-12.6081438523935));
#65332=CARTESIAN_POINT('Ctrl Pts',(39.7167261508899,1.31670092729021,-12.5920058261905));
#65333=CARTESIAN_POINT('Ctrl Pts',(39.8126662975388,1.31036906022431,-12.5758419238365));
#65334=CARTESIAN_POINT('Ctrl Pts',(39.9077307210829,1.30403719315842,-12.5551917162477));
#65335=CARTESIAN_POINT('Ctrl Pts',(40.0014794568133,1.29770532609252,-12.5301890677969));
#65336=CARTESIAN_POINT('Ctrl Pts',(40.0559302674504,1.29402767335515,-12.5156671175476));
#65337=CARTESIAN_POINT('Ctrl Pts',(40.1099375420237,1.29035002061777,-12.4996778081882));
#65338=CARTESIAN_POINT('Ctrl Pts',(40.1634181868812,1.2866723678804,-12.4822548165633));
#65339=CARTESIAN_POINT('Ctrl Pts',(40.2555075253338,1.28033974776062,-12.4522538362669));
#65340=CARTESIAN_POINT('Ctrl Pts',(40.3463541332558,1.27400712764084,-12.4178951367548));
#65341=CARTESIAN_POINT('Ctrl Pts',(40.4355161287737,1.26767450752106,-12.3793003605858));
#65342=CARTESIAN_POINT('Ctrl Pts',(40.524558126488,1.26135041009641,-12.3407575268205));
#65343=CARTESIAN_POINT('Ctrl Pts',(40.6119196200631,1.25502631267176,-12.297990119818));
#65344=CARTESIAN_POINT('Ctrl Pts',(40.697174425737,1.24870221524711,-12.2511693622772));
#65345=CARTESIAN_POINT('Ctrl Pts',(40.7823399950771,1.24238473726479,-12.2043976120941));
#65346=CARTESIAN_POINT('Ctrl Pts',(40.8654028790095,1.23606725928246,-12.1535811553654));
#65347=CARTESIAN_POINT('Ctrl Pts',(40.9459583408031,1.22974978130014,-12.0989386405041));
#65348=CARTESIAN_POINT('Ctrl Pts',(41.0264566216689,1.22343678767238,-12.0443349127049));
#65349=CARTESIAN_POINT('Ctrl Pts',(41.1044506579647,1.21712379404462,-11.9859107708638));
#65350=CARTESIAN_POINT('Ctrl Pts',(41.1795625661053,1.21081080041686,-11.9239294903716));
#65351=CARTESIAN_POINT('Ctrl Pts',(41.2546473310598,1.20450008811525,-11.8619706080512));
#65352=CARTESIAN_POINT('Ctrl Pts',(41.3268517004008,1.19818937581364,-11.7964574193223));
#65353=CARTESIAN_POINT('Ctrl Pts',(41.3958296707027,1.19187866351202,-11.7276944205136));
#65354=CARTESIAN_POINT('Ctrl Pts',(41.4648013972136,1.18556852244741,-11.658937646037));
#65355=CARTESIAN_POINT('Ctrl Pts',(41.5305469957859,1.1792583813828,-11.5869319552453));
#65356=CARTESIAN_POINT('Ctrl Pts',(41.5927570080808,1.17294824031818,-11.5120190117812));
#65357=CARTESIAN_POINT('Ctrl Pts',(41.654978238618,1.16663696135488,-11.4370925593736));
#65358=CARTESIAN_POINT('Ctrl Pts',(41.7136623372357,1.16032568239159,-11.3592581494967));
#65359=CARTESIAN_POINT('Ctrl Pts',(41.7685405279353,1.15401440342829,-11.278890021995));
#65360=CARTESIAN_POINT('Ctrl Pts',(41.8234774071826,1.14769637497505,-11.1984359461663));
#65361=CARTESIAN_POINT('Ctrl Pts',(41.8746000056417,1.14137834652181,-11.1154431048064));
#65362=CARTESIAN_POINT('Ctrl Pts',(41.9216833747809,1.13506031806857,-11.0303140072228));
#65363=CARTESIAN_POINT('Ctrl Pts',(41.9687943332519,1.12873858745496,-10.9451350267408));
#65364=CARTESIAN_POINT('Ctrl Pts',(42.0118611559856,1.12241685684135,-10.8578176894343));
#65365=CARTESIAN_POINT('Ctrl Pts',(42.0507062157808,1.11609512622774,-10.7687864463841));
#65366=CARTESIAN_POINT('Ctrl Pts',(42.0896135608007,1.10976325917944,-10.6796124482188));
#65367=CARTESIAN_POINT('Ctrl Pts',(42.1242854700353,1.10343139213113,-10.5887194651272));
#65368=CARTESIAN_POINT('Ctrl Pts',(42.1545935460052,1.09709952508282,-10.4965490882113));
#65369=CARTESIAN_POINT('Ctrl Pts',(42.1721969767555,1.09342187219535,-10.4430150120506));
#65370=CARTESIAN_POINT('Ctrl Pts',(42.1883292228158,1.08974421930789,-10.3890502585163));
#65371=CARTESIAN_POINT('Ctrl Pts',(42.2029730639892,1.08606656642042,-10.3347428171064));
#65372=CARTESIAN_POINT('Ctrl Pts',(42.2281885714969,1.07973394624948,-10.2412298050229));
#65373=CARTESIAN_POINT('Ctrl Pts',(42.2490757054682,1.07340132607854,-10.1463754208036));
#65374=CARTESIAN_POINT('Ctrl Pts',(42.2654947861516,1.0670687059076,-10.0506161802851));
#65375=CARTESIAN_POINT('Ctrl Pts',(42.2818917693775,1.06074460843094,-9.95498581639423));
#65376=CARTESIAN_POINT('Ctrl Pts',(42.2938325777206,1.05442051095429,-9.85845344400553));
#65377=CARTESIAN_POINT('Ctrl Pts',(42.3012276298065,1.04809641347763,-9.76146953508838));
#65378=CARTESIAN_POINT('Ctrl Pts',(42.3086149414812,1.04177893544254,-9.66458713936265));
#65379=CARTESIAN_POINT('Ctrl Pts',(42.3114659230558,1.03546145740745,-9.56725458046418));
#65380=CARTESIAN_POINT('Ctrl Pts',(42.309742429924,1.02914397937235,-9.46993029480624));
#65381=CARTESIAN_POINT('Ctrl Pts',(42.3080201601844,1.02283098569086,-9.37267509312588));
#65382=CARTESIAN_POINT('Ctrl Pts',(42.3017298789135,1.01651799200937,-9.27542858901532));
#65383=CARTESIAN_POINT('Ctrl Pts',(42.2908854897475,1.01020499832788,-9.17865112650952));
#65384=CARTESIAN_POINT('Ctrl Pts',(42.2800450194169,1.00389428597198,-9.08190863646093));
#65385=CARTESIAN_POINT('Ctrl Pts',(42.2646537598981,0.997583573616074,-8.98563528537614));
#65386=CARTESIAN_POINT('Ctrl Pts',(42.2447775587764,0.99127286126017,-8.89028725357704));
#65387=CARTESIAN_POINT('Ctrl Pts',(42.2249031568195,0.984962720140777,-8.7949478525432));
#65388=CARTESIAN_POINT('Ctrl Pts',(42.2005447098696,0.978652579021385,-8.70053403232942));
#65389=CARTESIAN_POINT('Ctrl Pts',(42.1718191649682,0.972342437901991,-8.60749168743394));
#65390=CARTESIAN_POINT('Ctrl Pts',(42.1430884400284,0.966031158883453,-8.51443256433925));
#65391=CARTESIAN_POINT('Ctrl Pts',(42.1099891820753,0.959719879864914,-8.42274582559994));
#65392=CARTESIAN_POINT('Ctrl Pts',(42.0726878545949,0.953408600846376,-8.33286110584249));
#65393=CARTESIAN_POINT('Ctrl Pts',(42.0353466358428,0.947090572337603,-8.24288026039698));
#65394=CARTESIAN_POINT('Ctrl Pts',(41.9937945437706,0.940772543828831,-8.15470568593885));
#65395=CARTESIAN_POINT('Ctrl Pts',(41.9482456711112,0.934454515320058,-8.06874576940746));
#65396=CARTESIAN_POINT('Ctrl Pts',(41.9026701082835,0.928132784650637,-7.98273548314129));
#65397=CARTESIAN_POINT('Ctrl Pts',(41.8530933239235,0.921811053981216,-7.89894281511702));
#65398=CARTESIAN_POINT('Ctrl Pts',(41.799773651133,0.915489323311794,-7.81774852005495));
#65399=CARTESIAN_POINT('Ctrl Pts',(41.7463684841319,0.909157456207825,-7.73642403585629));
#65400=CARTESIAN_POINT('Ctrl Pts',(41.6892087016501,0.902825589103855,-7.65770659763154));
#65401=CARTESIAN_POINT('Ctrl Pts',(41.6285938994227,0.896493721999885,-7.58194510510211));
#65402=CARTESIAN_POINT('Ctrl Pts',(41.5933878273459,0.8928160696534,-7.53794158667712));
#65403=CARTESIAN_POINT('Ctrl Pts',(41.5570169369935,0.889138417306913,-7.49493459441095));
#65404=CARTESIAN_POINT('Ctrl Pts',(41.5195454962285,0.885460764960428,-7.45298664487264));
#65405=CARTESIAN_POINT('Ctrl Pts',(41.4550227033396,0.879128144814911,-7.38075566562761));
#65406=CARTESIAN_POINT('Ctrl Pts',(41.3870106994681,0.872795524669392,-7.31141596690157));
#65407=CARTESIAN_POINT('Ctrl Pts',(41.3157986633026,0.866462904523875,-7.24532312174136));
#65408=CARTESIAN_POINT('Ctrl Pts',(41.2446824671559,0.860138807072926,-7.17931922698708));
#65409=CARTESIAN_POINT('Ctrl Pts',(41.1703751163723,0.853814709621979,-7.1165537957038));
#65410=CARTESIAN_POINT('Ctrl Pts',(41.0932048609678,0.847490612171031,-7.05734807817065));
#65411=CARTESIAN_POINT('Ctrl Pts',(41.0161153797798,0.841173134161922,-6.99820433134664));
#65412=CARTESIAN_POINT('Ctrl Pts',(40.9361692965096,0.834855656152813,-6.94261315568515));
#65413=CARTESIAN_POINT('Ctrl Pts',(40.8537296467609,0.828538178143704,-6.89085708278307));
#65414=CARTESIAN_POINT('Ctrl Pts',(40.7713485153901,0.822225184488502,-6.8391377480457));
#65415=CARTESIAN_POINT('Ctrl Pts',(40.6864777057602,0.8159121908333,-6.79124833587066));
#65416=CARTESIAN_POINT('Ctrl Pts',(40.5995103014359,0.809599197178097,-6.74742883636173));
#65417=CARTESIAN_POINT('Ctrl Pts',(40.5125743245118,0.803288484848641,-6.70362517189999));
#65418=CARTESIAN_POINT('Ctrl Pts',(40.4235436484879,0.796977772519183,-6.66388869429876));
#65419=CARTESIAN_POINT('Ctrl Pts',(40.3328362638571,0.790667060189726,-6.62841362079596));
#65420=CARTESIAN_POINT('Ctrl Pts',(40.2421370899287,0.784356919096905,-6.59294175844597));
#65421=CARTESIAN_POINT('Ctrl Pts',(40.1497619165014,0.778046778004085,-6.56173069234922));
#65422=CARTESIAN_POINT('Ctrl Pts',(40.0561480528386,0.771736636911264,-6.53492622757887));
#65423=CARTESIAN_POINT('Ctrl Pts',(39.9625173079169,0.765425357919411,-6.50811692919638));
#65424=CARTESIAN_POINT('Ctrl Pts',(39.8676478495388,0.759114078927558,-6.48571593073111));
#65425=CARTESIAN_POINT('Ctrl Pts',(39.7719904378764,0.752802799935705,-6.46781868514836));
#65426=CARTESIAN_POINT('Ctrl Pts',(39.6762307270179,0.746484771453607,-6.44990229965995));
#65427=CARTESIAN_POINT('Ctrl Pts',(39.5796818111064,0.740166742971509,-6.4364993634139));
#65428=CARTESIAN_POINT('Ctrl Pts',(39.4828026929409,0.733848714489411,-6.4276538311378));
#65429=CARTESIAN_POINT('Ctrl Pts',(39.3858668067417,0.727526983846716,-6.41880311566552));
#65430=CARTESIAN_POINT('Ctrl Pts',(39.2886007696971,0.721205253204021,-6.41451514109264));
#65431=CARTESIAN_POINT('Ctrl Pts',(39.1914646285191,0.714883522561326,-6.41478171178715));
#65432=CARTESIAN_POINT('Ctrl Pts',(39.0941727366117,0.708551655483863,-6.41504870990836));
#65433=CARTESIAN_POINT('Ctrl Pts',(38.9970115929632,0.702219788406399,-6.41988481414417));
#65434=CARTESIAN_POINT('Ctrl Pts',(38.9004371244342,0.695887921328936,-6.42922986375236));
#65435=CARTESIAN_POINT('Ctrl Pts',(38.8443450836742,0.692210268719442,-6.43465762236715));
#65436=CARTESIAN_POINT('Ctrl Pts',(38.7884508038198,0.688532616109947,-6.44160549850996));
#65437=CARTESIAN_POINT('Ctrl Pts',(38.7328417651375,0.684854963500453,-6.45005384819504));
#65438=CARTESIAN_POINT('Ctrl Pts',(38.6370875011892,0.678522343354097,-6.4646012225939));
#65439=CARTESIAN_POINT('Ctrl Pts',(38.5418470733761,0.672189723207741,-6.48365082630189));
#65440=CARTESIAN_POINT('Ctrl Pts',(38.4475763025267,0.665857103061384,-6.50715486938435));
#65441=CARTESIAN_POINT('Ctrl Pts',(38.3534324050684,0.659533005609661,-6.53062727978125));
#65442=CARTESIAN_POINT('Ctrl Pts',(38.2602559915588,0.653208908157937,-6.55854210938224));
#65443=CARTESIAN_POINT('Ctrl Pts',(38.1684954987019,0.646884810706214,-6.59080008917221));
#65444=CARTESIAN_POINT('Ctrl Pts',(38.0768310516849,0.640567332696389,-6.62302430448834));
#65445=CARTESIAN_POINT('Ctrl Pts',(37.9865799893365,0.634249854686566,-6.65958248809077));
#65446=CARTESIAN_POINT('Ctrl Pts',(37.8981773405126,0.627932376676741,-6.70032507779298));
#65447=CARTESIAN_POINT('Ctrl Pts',(37.8098374428005,0.621619383020876,-6.74103874706314));
#65448=CARTESIAN_POINT('Ctrl Pts',(37.7233437461858,0.615306389365011,-6.7859307349164));
#65449=CARTESIAN_POINT('Ctrl Pts',(37.6391120808485,0.608993395709147,-6.83480306357564));
#65450=CARTESIAN_POINT('Ctrl Pts',(37.5549108542985,0.602682683379081,-6.88365773124704));
#65451=CARTESIAN_POINT('Ctrl Pts',(37.4729704126545,0.596371971049014,-6.93648966241158));
#65452=CARTESIAN_POINT('Ctrl Pts',(37.3936818713432,0.590061258718948,-6.99305500237745));
#65453=CARTESIAN_POINT('Ctrl Pts',(37.3144005071177,0.583751117625572,-7.04961522212933));
#65454=CARTESIAN_POINT('Ctrl Pts',(37.2377709218384,0.577440976532196,-7.10990792462877));
#65455=CARTESIAN_POINT('Ctrl Pts',(37.164154251486,0.57113083543882,-7.17364661499862));
#65456=CARTESIAN_POINT('Ctrl Pts',(37.0905243059421,0.564819556446501,-7.23739679927759));
#65457=CARTESIAN_POINT('Ctrl Pts',(37.0199086850006,0.558508277454183,-7.30459391935354));
#65458=CARTESIAN_POINT('Ctrl Pts',(36.9526337132396,0.552196998461865,-7.37491269339294));
#65459=CARTESIAN_POINT('Ctrl Pts',(36.8852867954021,0.545878969979356,-7.44530666865163));
#65460=CARTESIAN_POINT('Ctrl Pts',(36.8212879620569,0.539560941496847,-7.51882864629538));
#65461=CARTESIAN_POINT('Ctrl Pts',(36.7609249196866,0.533242913014338,-7.59511829235724));
#65462=CARTESIAN_POINT('Ctrl Pts',(36.7005265065239,0.526921182371293,-7.67145264168656));
#65463=CARTESIAN_POINT('Ctrl Pts',(36.643768381483,0.520599451728249,-7.75055753365188));
#65464=CARTESIAN_POINT('Ctrl Pts',(36.5908951519223,0.514277721085204,-7.83204325376056));
#65465=CARTESIAN_POINT('Ctrl Pts',(36.5379371439888,0.507945854007472,-7.91365963028698));
#65466=CARTESIAN_POINT('Ctrl Pts',(36.4888766904532,0.501613986929741,-7.99766408041352));
#65467=CARTESIAN_POINT('Ctrl Pts',(36.4439126320639,0.49528211985201,-8.08364193442328));
#65468=CARTESIAN_POINT('Ctrl Pts',(36.4177967669668,0.491604467248162,-8.13357928699093));
#65469=CARTESIAN_POINT('Ctrl Pts',(36.3930619200093,0.487926814644315,-8.1841819632088));
#65470=CARTESIAN_POINT('Ctrl Pts',(36.3697394600482,0.484249162040468,-8.23536597094681));
#65471=CARTESIAN_POINT('Ctrl Pts',(36.3240692249413,0.47704755211852,-8.33559492068105));
#65472=CARTESIAN_POINT('Ctrl Pts',(36.2836741068734,0.469845942196575,-8.43836987688406));
#65473=CARTESIAN_POINT('Ctrl Pts',(36.2488179398193,0.462644332274628,-8.54313692371715));
#65474=CARTESIAN_POINT('Ctrl Pts',(36.2155628225379,0.455773514201086,-8.6430917014258));
#65475=CARTESIAN_POINT('Ctrl Pts',(36.1873493158459,0.448902696127545,-8.74485929566455));
#65476=CARTESIAN_POINT('Ctrl Pts',(36.1643595640711,0.442031878054002,-8.84793442219139));
#65477=CARTESIAN_POINT('Ctrl Pts',(36.1414261472589,0.435177896494522,-8.95075696950586));
#65478=CARTESIAN_POINT('Ctrl Pts',(36.123691054362,0.428323914935042,-9.0548803662193));
#65479=CARTESIAN_POINT('Ctrl Pts',(36.1112870594205,0.421469933375563,-9.15978359347306));
#65480=CARTESIAN_POINT('Ctrl Pts',(36.0989262652497,0.414639822938852,-9.26432146260688));
#65481=CARTESIAN_POINT('Ctrl Pts',(36.0918596059849,0.407809712502143,-9.36963344301793));
#65482=CARTESIAN_POINT('Ctrl Pts',(36.0901688933401,0.400979602065433,-9.47518894750603));
#65483=CARTESIAN_POINT('Ctrl Pts',(36.0899089982004,0.399929682369326,-9.49141486423484));
#65484=CARTESIAN_POINT('Ctrl Pts',(36.0897760372556,0.398879762673219,-9.50764651150324));
#65485=CARTESIAN_POINT('Ctrl Pts',(36.08977020096,0.397829842977112,-9.52388193753633));
#65486=CARTESIAN_POINT('',(36.0897712321793,-0.872170157086845,-9.5277685231493));
#65487=CARTESIAN_POINT('Ctrl Pts',(36.0897702009597,0.39782984291316,-9.52388193852522));
#65488=CARTESIAN_POINT('Ctrl Pts',(36.0897343557348,0.391381464763058,-9.62359638990521));
#65489=CARTESIAN_POINT('Ctrl Pts',(36.0944981487142,0.384933086612956,-9.7232801458052));
#65490=CARTESIAN_POINT('Ctrl Pts',(36.1040264597517,0.378484708462853,-9.82245334253061));
#65491=CARTESIAN_POINT('Ctrl Pts',(36.1135603149128,0.372032578272663,-9.92168424396891));
#65492=CARTESIAN_POINT('Ctrl Pts',(36.1278641678259,0.365580448082471,-10.0204035870194));
#65493=CARTESIAN_POINT('Ctrl Pts',(36.1468512464212,0.359128317892281,-10.1181385516219));
#65494=CARTESIAN_POINT('Ctrl Pts',(36.1658692662952,0.352665673332668,-10.2160327847905));
#65495=CARTESIAN_POINT('Ctrl Pts',(36.1895856790021,0.346203028773054,-10.3129390317701));
#65496=CARTESIAN_POINT('Ctrl Pts',(36.217862847812,0.339740384213441,-10.4083960937427));
#65497=CARTESIAN_POINT('Ctrl Pts',(36.2461635676093,0.333272357160923,-10.503932658302));
#65498=CARTESIAN_POINT('Ctrl Pts',(36.2790324788456,0.326804330108407,-10.5980172454756));
#65499=CARTESIAN_POINT('Ctrl Pts',(36.3162831849237,0.320336303055889,-10.6902072705516));
#65500=CARTESIAN_POINT('Ctrl Pts',(36.3536114327368,0.313854812042757,-10.7825892000301));
#65501=CARTESIAN_POINT('Ctrl Pts',(36.3953395343823,0.307373321029622,-10.8730683119811));
#65502=CARTESIAN_POINT('Ctrl Pts',(36.4412340768188,0.300891830016489,-10.9612246460753));
#65503=CARTESIAN_POINT('Ctrl Pts',(36.4819454198771,0.295142340204486,-11.0394248539767));
#65504=CARTESIAN_POINT('Ctrl Pts',(36.5259344897854,0.289392850392485,-11.1157975248511));
#65505=CARTESIAN_POINT('Ctrl Pts',(36.5730104120667,0.283643360580482,-11.1900694753642));
#65506=CARTESIAN_POINT('Ctrl Pts',(36.624860914235,0.277310740431624,-11.2718743077396));
#65507=CARTESIAN_POINT('Ctrl Pts',(36.6806262385994,0.270978120282766,-11.3513969780834));
#65508=CARTESIAN_POINT('Ctrl Pts',(36.7400792061342,0.264645500133907,-11.4282394333889));
#65509=CARTESIAN_POINT('Ctrl Pts',(36.7994521594771,0.258321402679619,-11.5049784710314));
#65510=CARTESIAN_POINT('Ctrl Pts',(36.8625026264951,0.251997305225331,-11.579044120041));
#65511=CARTESIAN_POINT('Ctrl Pts',(36.9289592727588,0.245673207771043,-11.6500658032427));
#65512=CARTESIAN_POINT('Ctrl Pts',(36.9953463587561,0.239355729758577,-11.7210131479474));
#65513=CARTESIAN_POINT('Ctrl Pts',(37.0651322388804,0.23303825174611,-11.7889225433691));
#65514=CARTESIAN_POINT('Ctrl Pts',(37.1380049329877,0.226720773733644,-11.8534559253971));
#65515=CARTESIAN_POINT('Ctrl Pts',(37.2108258996572,0.220407780075086,-11.9179434995057));
#65516=CARTESIAN_POINT('Ctrl Pts',(37.2867289977642,0.214094786416527,-11.9790595353139));
#65517=CARTESIAN_POINT('Ctrl Pts',(37.3653656506136,0.20778179275797,-12.0365030274621));
#65518=CARTESIAN_POINT('Ctrl Pts',(37.4439738865452,0.20147108042517,-12.0939257612625));
#65519=CARTESIAN_POINT('Ctrl Pts',(37.5253133616304,0.195160368092372,-12.1476783307608));
#65520=CARTESIAN_POINT('Ctrl Pts',(37.6090034464273,0.188849655759572,-12.1975008174779));
#65521=CARTESIAN_POINT('Ctrl Pts',(37.6926859557175,0.182539514663424,-12.2473187943347));
#65522=CARTESIAN_POINT('Ctrl Pts',(37.7787182758046,0.176229373567277,-12.2932071721927));
#65523=CARTESIAN_POINT('Ctrl Pts',(37.8666928061809,0.169919232471129,-12.3349506365433));
#65524=CARTESIAN_POINT('Ctrl Pts',(37.9546832008825,0.163607953475969,-12.3767016284351));
#65525=CARTESIAN_POINT('Ctrl Pts',(38.0446161063843,0.157296674480808,-12.4143060348617));
#65526=CARTESIAN_POINT('Ctrl Pts',(38.136062423033,0.150985395485647,-12.4475960181348));
#65527=CARTESIAN_POINT('Ctrl Pts',(38.2276065353931,0.144667367000273,-12.4809216028156));
#65528=CARTESIAN_POINT('Ctrl Pts',(38.3206668785228,0.138349338514899,-12.5099234029303));
#65529=CARTESIAN_POINT('Ctrl Pts',(38.4147978045665,0.132031310029525,-12.5344830395246));
#65530=CARTESIAN_POINT('Ctrl Pts',(38.5089838882917,0.125709579383574,-12.5590570672726));
#65531=CARTESIAN_POINT('Ctrl Pts',(38.6042413764323,0.119387848737622,-12.5791836579252));
#65532=CARTESIAN_POINT('Ctrl Pts',(38.7001150682789,0.113066118091671,-12.5947957111082));
#65533=CARTESIAN_POINT('Ctrl Pts',(38.7961424866082,0.106734251011021,-12.6104327970814));
#65534=CARTESIAN_POINT('Ctrl Pts',(38.8927876474032,0.10040238393037,-12.6215408412043));
#65535=CARTESIAN_POINT('Ctrl Pts',(38.9895909217126,0.0940705168497189,
-12.6281046828417));
#65536=CARTESIAN_POINT('Ctrl Pts',(39.0458158561015,0.090392864273315,-12.6319170700573));
#65537=CARTESIAN_POINT('Ctrl Pts',(39.1020941225829,0.086715211696911,-12.6341974578348));
#65538=CARTESIAN_POINT('Ctrl Pts',(39.1583362066502,0.0830375591205073,
-12.6349509290701));
#65539=CARTESIAN_POINT('Ctrl Pts',(39.2551805244327,0.0767049389712069,
-12.636248345568));
#65540=CARTESIAN_POINT('Ctrl Pts',(39.3522537177662,0.0703723188219073,
-12.6330200894804));
#65541=CARTESIAN_POINT('Ctrl Pts',(39.4490982840774,0.0640396986726079,
-12.6252388130223));
#65542=CARTESIAN_POINT('Ctrl Pts',(39.5458125130811,0.0577156012178801,
-12.6174680089186));
#65543=CARTESIAN_POINT('Ctrl Pts',(39.6422982943944,0.0513915037631515,
-12.6051563981387));
#65544=CARTESIAN_POINT('Ctrl Pts',(39.7380969970189,0.0450674063084238,
-12.5883286266249));
#65545=CARTESIAN_POINT('Ctrl Pts',(39.8337954270048,0.0387499282955115,
-12.5715184687635));
#65546=CARTESIAN_POINT('Ctrl Pts',(39.9288077795831,0.0324324502826007,
-12.5502016230762));
#65547=CARTESIAN_POINT('Ctrl Pts',(40.0226804318778,0.0261149722696885,
-12.5244545437305));
#65548=CARTESIAN_POINT('Ctrl Pts',(40.1164864502727,0.0198019786107041,
-12.4987257405095));
#65549=CARTESIAN_POINT('Ctrl Pts',(40.2091539561765,0.0134889849517186,
-12.4685730708776));
#65550=CARTESIAN_POINT('Ctrl Pts',(40.3002403546591,0.00717599129273427,
-12.4341238912909));
#65551=CARTESIAN_POINT('Ctrl Pts',(40.3912938372609,0.000865278959509648,
-12.3996871606001));
#65552=CARTESIAN_POINT('Ctrl Pts',(40.4807669391273,-0.0054454333737152,
-12.3609571595875));
#65553=CARTESIAN_POINT('Ctrl Pts',(40.5682339500845,-0.0117561457069399,
-12.3181105439521));
#65554=CARTESIAN_POINT('Ctrl Pts',(40.6556930436529,-0.0180662868035042,
-12.275267806731));
#65555=CARTESIAN_POINT('Ctrl Pts',(40.7411460147206,-0.0243764279000681,
-12.2283093883281));
#65556=CARTESIAN_POINT('Ctrl Pts',(40.8241897607595,-0.0306865689966322,
-12.177458910887));
#65557=CARTESIAN_POINT('Ctrl Pts',(40.9072484819621,-0.0369978479921994,
-12.1265992636498));
#65558=CARTESIAN_POINT('Ctrl Pts',(40.987896742334,-0.043309126987767,-12.0718463918084));
#65559=CARTESIAN_POINT('Ctrl Pts',(41.0657594437187,-0.0496204059833341,
-12.0134678722207));
#65560=CARTESIAN_POINT('Ctrl Pts',(41.143705414048,-0.0559384344691134,
-11.9550269207159));
#65561=CARTESIAN_POINT('Ctrl Pts',(41.2188595275753,-0.0622564629548936,
-11.8929528432398));
#65562=CARTESIAN_POINT('Ctrl Pts',(41.2908790564124,-0.068574491440673,
-11.8275541088878));
#65563=CARTESIAN_POINT('Ctrl Pts',(41.3629407863668,-0.0748962220870305,
-11.7621170529902));
#65564=CARTESIAN_POINT('Ctrl Pts',(41.431863964685,-0.0812179527333876,
-11.6933517696709));
#65565=CARTESIAN_POINT('Ctrl Pts',(41.4973435814427,-0.0875396833797453,
-11.621602757249));
#65566=CARTESIAN_POINT('Ctrl Pts',(41.562928189997,-0.0938715504607866,
-11.5497387005111));
#65567=CARTESIAN_POINT('Ctrl Pts',(41.6250579324058,-0.100203417541828,
-11.4748816977733));
#65568=CARTESIAN_POINT('Ctrl Pts',(41.6834688715607,-0.106535284622869,
-11.3974083467259));
#65569=CARTESIAN_POINT('Ctrl Pts',(41.7173949059955,-0.110212937195073,
-11.3524105498503));
#65570=CARTESIAN_POINT('Ctrl Pts',(41.750067224777,-0.113890589767275,-11.3065306738168));
#65571=CARTESIAN_POINT('Ctrl Pts',(41.781441153907,-0.117568242339479,-11.259846454824));
#65572=CARTESIAN_POINT('Ctrl Pts',(41.8354645212297,-0.12390086248949,-11.1794600071983));
#65573=CARTESIAN_POINT('Ctrl Pts',(41.8858232817599,-0.130233482639502,
-11.0964080852364));
#65574=CARTESIAN_POINT('Ctrl Pts',(41.9322444554138,-0.136566102789513,
-11.0110588443129));
#65575=CARTESIAN_POINT('Ctrl Pts',(41.9786031535875,-0.142890200244962,
-10.9258244698262));
#65576=CARTESIAN_POINT('Ctrl Pts',(42.0210345904329,-0.149214297700411,
-10.8382993024448));
#65577=CARTESIAN_POINT('Ctrl Pts',(42.0593087076327,-0.155538395155859,
-10.7488808632199));
#65578=CARTESIAN_POINT('Ctrl Pts',(42.0975427632596,-0.161855873169507,
-10.6595560184025));
#65579=CARTESIAN_POINT('Ctrl Pts',(42.1316279789981,-0.168173351183154,
-10.5683422413577));
#65580=CARTESIAN_POINT('Ctrl Pts',(42.1613804173148,-0.174490829196802,
-10.4756611787828));
#65581=CARTESIAN_POINT('Ctrl Pts',(42.1911117363711,-0.180803822856548,
-10.3830459042777));
#65582=CARTESIAN_POINT('Ctrl Pts',(42.2165162590907,-0.187116816516293,
-10.2889658300647));
#65583=CARTESIAN_POINT('Ctrl Pts',(42.2374587006585,-0.193429810176038,
-10.1938611923964));
#65584=CARTESIAN_POINT('Ctrl Pts',(42.2583935742588,-0.199740522510024,
-10.0987909226795));
#65585=CARTESIAN_POINT('Ctrl Pts',(42.2748694767364,-0.20605123484401,-10.0026972518387));
#65586=CARTESIAN_POINT('Ctrl Pts',(42.286801635077,-0.212361947177996,-9.90603322504187));
#65587=CARTESIAN_POINT('Ctrl Pts',(42.2987327133358,-0.218672088275344,
-9.80937794813424));
#65588=CARTESIAN_POINT('Ctrl Pts',(42.3061208118354,-0.224982229372693,
-9.71215285196113));
#65589=CARTESIAN_POINT('Ctrl Pts',(42.30893284416,-0.231292370470041,-9.61481772321296));
#65590=CARTESIAN_POINT('Ctrl Pts',(42.3117453835745,-0.237603649466402,
-9.51746504215571));
#65591=CARTESIAN_POINT('Ctrl Pts',(42.3099802052781,-0.243914928462761,
-9.42000272624048));
#65592=CARTESIAN_POINT('Ctrl Pts',(42.303656337438,-0.250226207459121,-9.3228911382925));
#65593=CARTESIAN_POINT('Ctrl Pts',(42.2973257066449,-0.256544235945681,
-9.22567569600509));
#65594=CARTESIAN_POINT('Ctrl Pts',(42.2864266816765,-0.26286226443224,-9.12881216761935));
#65595=CARTESIAN_POINT('Ctrl Pts',(42.271030227304,-0.2691802929188,-9.0327561621666));
#65596=CARTESIAN_POINT('Ctrl Pts',(42.2556247511067,-0.275502023565946,
-8.93664387099778));
#65597=CARTESIAN_POINT('Ctrl Pts',(42.2357166871887,-0.281823754213095,
-8.84134047288126));
#65598=CARTESIAN_POINT('Ctrl Pts',(42.2114277878788,-0.288145484860242,
-8.74728968677825));
#65599=CARTESIAN_POINT('Ctrl Pts',(42.1870999430878,-0.294477351942071,
-8.65308809708942));
#65600=CARTESIAN_POINT('Ctrl Pts',(42.1583773655456,-0.3008092190239,-8.56014354753402));
#65601=CARTESIAN_POINT('Ctrl Pts',(42.1254311381782,-0.307141086105729,
-8.46888290957993));
#65602=CARTESIAN_POINT('Ctrl Pts',(42.1062954273358,-0.310818738670307,
-8.41587722975762));
#65603=CARTESIAN_POINT('Ctrl Pts',(42.0857357750569,-0.314496391234885,
-8.36343922708463));
#65604=CARTESIAN_POINT('Ctrl Pts',(42.0637928565438,-0.318174043799464,
-8.3116488028156));
#65605=CARTESIAN_POINT('Ctrl Pts',(42.0260089263125,-0.324506663948962,
-8.2224698826979));
#65606=CARTESIAN_POINT('Ctrl Pts',(41.983989833842,-0.330839284098463,-8.13490263785141));
#65607=CARTESIAN_POINT('Ctrl Pts',(41.9378946495576,-0.337171904247962,
-8.0493768974349));
#65608=CARTESIAN_POINT('Ctrl Pts',(41.8918615020238,-0.343496001702896,
-7.96396626099521));
#65609=CARTESIAN_POINT('Ctrl Pts',(41.8417633716234,-0.34982009915783,-7.88059204983426));
#65610=CARTESIAN_POINT('Ctrl Pts',(41.7878073809052,-0.356144196612765,
-7.7996642030513));
#65611=CARTESIAN_POINT('Ctrl Pts',(41.7339078659995,-0.362461674625868,
-7.71882106356106));
#65612=CARTESIAN_POINT('Ctrl Pts',(41.6761587598858,-0.36877915263897,-7.64041955977328));
#65613=CARTESIAN_POINT('Ctrl Pts',(41.6148125979747,-0.375096630652074,
-7.56484419763051));
#65614=CARTESIAN_POINT('Ctrl Pts',(41.5535099815891,-0.381409624311284,
-7.48932248136806));
#65615=CARTESIAN_POINT('Ctrl Pts',(41.4886156603618,-0.387722617970494,
-7.41662325709803));
#65616=CARTESIAN_POINT('Ctrl Pts',(41.4204243307487,-0.394035611629704,
-7.34710045127899));
#65617=CARTESIAN_POINT('Ctrl Pts',(41.3522576434282,-0.400346323963149,
-7.277602768908));
#65618=CARTESIAN_POINT('Ctrl Pts',(41.2807966210374,-0.406657036296594,
-7.21127953605949));
#65619=CARTESIAN_POINT('Ctrl Pts',(41.206374296686,-0.412967748630038,-7.14844938313994));
#65620=CARTESIAN_POINT('Ctrl Pts',(41.1319587089367,-0.419277889726845,
-7.0856249175158));
#65621=CARTESIAN_POINT('Ctrl Pts',(41.0545826864648,-0.425588030823653,
-7.02629318510998));
#65622=CARTESIAN_POINT('Ctrl Pts',(40.974613160478,-0.43189817192046,-6.97073321997129));
#65623=CARTESIAN_POINT('Ctrl Pts',(40.8946292136973,-0.438209450916274,
-6.91516323578102));
#65624=CARTESIAN_POINT('Ctrl Pts',(40.8120511936819,-0.444520729912088,
-6.86336661922318));
#65625=CARTESIAN_POINT('Ctrl Pts',(40.7272750009004,-0.450832008907901,
-6.81557907948492));
#65626=CARTESIAN_POINT('Ctrl Pts',(40.6424081456583,-0.457150037393917,
-6.76774043417337));
#65627=CARTESIAN_POINT('Ctrl Pts',(40.5553388059945,-0.463468065879932,
-6.72391964041467));
#65628=CARTESIAN_POINT('Ctrl Pts',(40.466487291168,-0.469786094365948,-6.68430631813108));
#65629=CARTESIAN_POINT('Ctrl Pts',(40.3775837122242,-0.476107825012546,
-6.64466978372038));
#65630=CARTESIAN_POINT('Ctrl Pts',(40.2868962857968,-0.482429555659144,
-6.60924578919691));
#65631=CARTESIAN_POINT('Ctrl Pts',(40.194863126059,-0.488751286305741,-6.57817492658485));
#65632=CARTESIAN_POINT('Ctrl Pts',(40.1026823978522,-0.495083153387022,
-6.54705424410747));
#65633=CARTESIAN_POINT('Ctrl Pts',(40.0091520478015,-0.501415020468303,
-6.52030075142709));
#65634=CARTESIAN_POINT('Ctrl Pts',(39.9147230473378,-0.507746887549584,
-6.49800452288013));
#65635=CARTESIAN_POINT('Ctrl Pts',(39.8598771303633,-0.511424540119536,
-6.48505450653212));
#65636=CARTESIAN_POINT('Ctrl Pts',(39.8047282224243,-0.515102192689488,
-6.4736071754637));
#65637=CARTESIAN_POINT('Ctrl Pts',(39.7493654651879,-0.51877984525944,-6.46367214454922));
#65638=CARTESIAN_POINT('Ctrl Pts',(39.6540352768832,-0.525112465409043,
-6.44656482520372));
#65639=CARTESIAN_POINT('Ctrl Pts',(39.557739655896,-0.531445085558645,-6.43388492453164));
#65640=CARTESIAN_POINT('Ctrl Pts',(39.460925484113,-0.537777705708248,-6.42573419264491));
#65641=CARTESIAN_POINT('Ctrl Pts',(39.3642416087312,-0.544101803163289,
-6.41759443034054));
#65642=CARTESIAN_POINT('Ctrl Pts',(39.2670410017269,-0.550425900618329,
-6.41397175803448));
#65643=CARTESIAN_POINT('Ctrl Pts',(39.169780155618,-0.556749998073369,-6.41491681559713));
#65644=CARTESIAN_POINT('Ctrl Pts',(39.0726211125755,-0.56306747608658,-6.41586088396667));
#65645=CARTESIAN_POINT('Ctrl Pts',(38.9754023907747,-0.569384954099792,
-6.42136317302188));
#65646=CARTESIAN_POINT('Ctrl Pts',(38.8785840090073,-0.575702432113004,
-6.43142239249859));
#65647=CARTESIAN_POINT('Ctrl Pts',(38.781834352115,-0.582015425772317,-6.44147447161011));
#65648=CARTESIAN_POINT('Ctrl Pts',(38.6854849040381,-0.588328419431632,
-6.45607700538267));
#65649=CARTESIAN_POINT('Ctrl Pts',(38.5899931228984,-0.594641413090945,
-6.47517668334889));
#65650=CARTESIAN_POINT('Ctrl Pts',(38.4945358496122,-0.600952125424498,
-6.49426945926678));
#65651=CARTESIAN_POINT('Ctrl Pts',(38.3999360558037,-0.607262837758047,
-6.5178560645398));
#65652=CARTESIAN_POINT('Ctrl Pts',(38.3066425988733,-0.6135735500916,-6.54583179280656));
#65653=CARTESIAN_POINT('Ctrl Pts',(38.2133575867334,-0.619883691188486,
-6.57380498875036));
#65654=CARTESIAN_POINT('Ctrl Pts',(38.1213790951914,-0.626193832285376,
-6.60616639196017));
#65655=CARTESIAN_POINT('Ctrl Pts',(38.0311413537314,-0.632503973382262,
-6.6427612663169));
#65656=CARTESIAN_POINT('Ctrl Pts',(37.9408873398241,-0.638815252378183,
-6.67936273977682));
#65657=CARTESIAN_POINT('Ctrl Pts',(37.8523751046955,-0.645126531374105,
-6.7201990362465));
#65658=CARTESIAN_POINT('Ctrl Pts',(37.766018433538,-0.651437810370027,-6.76506747909534));
#65659=CARTESIAN_POINT('Ctrl Pts',(37.6795694097043,-0.657755838856146,
-6.8099839057388));
#65660=CARTESIAN_POINT('Ctrl Pts',(37.5952809408086,-0.664073867342263,
-6.85894088569714));
#65661=CARTESIAN_POINT('Ctrl Pts',(37.5135415600515,-0.670391895828382,
-6.91169010960686));
#65662=CARTESIAN_POINT('Ctrl Pts',(37.4317542826579,-0.676713626475093,
-6.96447024285776));
#65663=CARTESIAN_POINT('Ctrl Pts',(37.3525194234754,-0.683035357121804,
-7.02104679092049));
#65664=CARTESIAN_POINT('Ctrl Pts',(37.2761941931527,-0.689357087768515,
-7.08112973534995));
#65665=CARTESIAN_POINT('Ctrl Pts',(37.1997465808821,-0.695688954849898,
-7.14130901840487));
#65666=CARTESIAN_POINT('Ctrl Pts',(37.1262182437386,-0.702020821931283,
-7.20500563831858));
#65667=CARTESIAN_POINT('Ctrl Pts',(37.0559311178139,-0.708352689012665,
-7.27189119629315));
#65668=CARTESIAN_POINT('Ctrl Pts',(37.0151071987555,-0.712030341581586,
-7.31073942872559));
#65669=CARTESIAN_POINT('Ctrl Pts',(36.9753759799599,-0.715707994150504,
-7.35066277636454));
#65670=CARTESIAN_POINT('Ctrl Pts',(36.9367942392651,-0.719385646719425,
-7.39159184929921));
#65671=CARTESIAN_POINT('Ctrl Pts',(36.8700091971459,-0.725751667984734,
-7.46244012650557));
#65672=CARTESIAN_POINT('Ctrl Pts',(36.8064215504707,-0.732117689250043,
-7.53656840224095));
#65673=CARTESIAN_POINT('Ctrl Pts',(36.7463748568544,-0.738483710515352,
-7.61365118049482));
#65674=CARTESIAN_POINT('Ctrl Pts',(36.6874698523395,-0.744728692358501,
-7.68926835652253));
#65675=CARTESIAN_POINT('Ctrl Pts',(36.6319726606026,-0.750973674201652,
-7.76772832768793));
#65676=CARTESIAN_POINT('Ctrl Pts',(36.5801714436936,-0.757218656044802,
-7.84868589206516));
#65677=CARTESIAN_POINT('Ctrl Pts',(36.5284184462394,-0.76345782471139,-7.92956809663711));
#65678=CARTESIAN_POINT('Ctrl Pts',(36.4803548329806,-0.769696993377978,
-8.01294290208393));
#65679=CARTESIAN_POINT('Ctrl Pts',(36.4362275009105,-0.775936162044567,
-8.09843341333937));
#65680=CARTESIAN_POINT('Ctrl Pts',(36.3921285670166,-0.782171315489688,
-8.18386890711501));
#65681=CARTESIAN_POINT('Ctrl Pts',(36.3519610877662,-0.788406468934808,
-8.27141700411107));
#65682=CARTESIAN_POINT('Ctrl Pts',(36.3159271122552,-0.794641622379929,
-8.36067434492102));
#65683=CARTESIAN_POINT('Ctrl Pts',(36.2785896012964,-0.801102333605506,
-8.45316058584701));
#65684=CARTESIAN_POINT('Ctrl Pts',(36.2456905899654,-0.807563044831082,
-8.54748164869504));
#65685=CARTESIAN_POINT('Ctrl Pts',(36.2174009197196,-0.814023756056659,
-8.64316476640455));
#65686=CARTESIAN_POINT('Ctrl Pts',(36.1901025329634,-0.820258080890536,
-8.73549510219756));
#65687=CARTESIAN_POINT('Ctrl Pts',(36.1670959464817,-0.826492405724413,
-8.82909316493853));
#65688=CARTESIAN_POINT('Ctrl Pts',(36.1484837600194,-0.83272673055829,-8.92351908589345));
#65689=CARTESIAN_POINT('Ctrl Pts',(36.1298684664969,-0.838962096130854,
-9.01796077001624));
#65690=CARTESIAN_POINT('Ctrl Pts',(36.1156491071054,-0.845197461703417,
-9.1132301443313));
#65691=CARTESIAN_POINT('Ctrl Pts',(36.1058768389215,-0.851432827275981,
-9.20887895201744));
#65692=CARTESIAN_POINT('Ctrl Pts',(36.0960970467662,-0.857672993649282,
-9.30460140267786));
#65693=CARTESIAN_POINT('Ctrl Pts',(36.0907712056005,-0.863913160022584,
-9.40070342170071));
#65694=CARTESIAN_POINT('Ctrl Pts',(36.089898442095,-0.870153326395885,-9.49673425364528));
#65695=CARTESIAN_POINT('Ctrl Pts',(36.0898044159576,-0.870825603292871,
-9.50708002102593));
#65696=CARTESIAN_POINT('Ctrl Pts',(36.0897620250169,-0.871497880189858,
-9.51742496460401));
#65697=CARTESIAN_POINT('Ctrl Pts',(36.0897712321793,-0.872170157086845,
-9.5277685231493));
#65698=CARTESIAN_POINT('',(36.0897704137311,-2.14217015708684,-9.52339575640588));
#65699=CARTESIAN_POINT('Ctrl Pts',(36.0899125803325,-0.872170241694712,
-9.5277696990371));
#65700=CARTESIAN_POINT('Ctrl Pts',(36.0877068998987,-0.888110643856278,
-9.77301751196299));
#65701=CARTESIAN_POINT('Ctrl Pts',(36.2258738429507,-0.970919646504489,
-11.0446027236326));
#65702=CARTESIAN_POINT('Ctrl Pts',(37.9701641530118,-1.12059724963941,-12.9826522251454));
#65703=CARTESIAN_POINT('Ctrl Pts',(41.4231224819371,-1.32120305109937,-12.4448598512402));
#65704=CARTESIAN_POINT('Ctrl Pts',(42.8602373914268,-1.52180885255935,-9.25944895221449));
#65705=CARTESIAN_POINT('Ctrl Pts',(40.9783874130057,-1.72241465401934,-6.31482970391815));
#65706=CARTESIAN_POINT('Ctrl Pts',(37.483962962039,-1.92302045547933,-6.28107151667509));
#65707=CARTESIAN_POINT('Ctrl Pts',(36.1319771607599,-2.06293895650182,-8.30914305999039));
#65708=CARTESIAN_POINT('Ctrl Pts',(36.0852272677007,-2.13598885703766,-9.42861603492319));
#65709=CARTESIAN_POINT('Ctrl Pts',(36.0858265164569,-2.14217015708684,-9.52339372215993));
#65710=CARTESIAN_POINT('',(36.0897702438652,-3.41217015705251,-9.52376835315985));
#65711=CARTESIAN_POINT('Ctrl Pts',(36.0897704137311,-2.14217015708684,-9.52339575640588));
#65712=CARTESIAN_POINT('Ctrl Pts',(36.0897210100065,-2.14842487072775,-9.61917729887397));
#65713=CARTESIAN_POINT('Ctrl Pts',(36.0941003085369,-2.15467958436866,-9.7151342087082));
#65714=CARTESIAN_POINT('Ctrl Pts',(36.1029305733703,-2.16093429800956,-9.81081745841623));
#65715=CARTESIAN_POINT('Ctrl Pts',(36.1117498912511,-2.16718125763004,-9.90638208880517));
#65716=CARTESIAN_POINT('Ctrl Pts',(36.1250091728486,-2.17342821725052,-10.0016732896905));
#65717=CARTESIAN_POINT('Ctrl Pts',(36.1426786579585,-2.17967517687099,-10.0962415114449));
#65718=CARTESIAN_POINT('Ctrl Pts',(36.1603314513654,-2.18591623522185,-10.1907203981295));
#65719=CARTESIAN_POINT('Ctrl Pts',(36.1823860860398,-2.19215729357271,-10.2844772239474));
#65720=CARTESIAN_POINT('Ctrl Pts',(36.2087610630663,-2.19839835192357,-10.377068233812));
#65721=CARTESIAN_POINT('Ctrl Pts',(36.235122762356,-2.20463626838999,-10.4696126313497));
#65722=CARTESIAN_POINT('Ctrl Pts',(36.2658003628854,-2.21087418485642,-10.5609919475004));
#65723=CARTESIAN_POINT('Ctrl Pts',(36.3006616346398,-2.21711210132285,-10.6507742651395));
#65724=CARTESIAN_POINT('Ctrl Pts',(36.3355153493107,-2.22334866555934,-10.7405371201361));
#65725=CARTESIAN_POINT('Ctrl Pts',(36.374550771124,-2.22958522979582,-10.8287032461613));
#65726=CARTESIAN_POINT('Ctrl Pts',(36.4175867298321,-2.2358217940323,-10.9148586427739));
#65727=CARTESIAN_POINT('Ctrl Pts',(36.4606256955022,-2.24205879402327,-11.0010200591434));
#65728=CARTESIAN_POINT('Ctrl Pts',(36.5076655512623,-2.24829579401424,-11.0851700662614));
#65729=CARTESIAN_POINT('Ctrl Pts',(36.5584787228057,-2.2545327940052,-11.166918388663));
#65730=CARTESIAN_POINT('Ctrl Pts',(36.6093418550827,-2.26077592636473,-11.2487470879834));
#65731=CARTESIAN_POINT('Ctrl Pts',(36.6639854731947,-2.26701905872425,-11.3281690059682));
#65732=CARTESIAN_POINT('Ctrl Pts',(36.7221383179323,-2.27326219108377,-11.4048223685872));
#65733=CARTESIAN_POINT('Ctrl Pts',(36.7803211527836,-2.27950854310091,-11.481515262257));
#65734=CARTESIAN_POINT('Ctrl Pts',(36.8420165285394,-2.28575489511805,-11.5554364144923));
#65735=CARTESIAN_POINT('Ctrl Pts',(36.906913942458,-2.29200124713519,-11.6262584290388));
#65736=CARTESIAN_POINT('Ctrl Pts',(36.9719170676987,-2.29825777382787,-11.6971958054824));
#65737=CARTESIAN_POINT('Ctrl Pts',(37.0401323275585,-2.30451430052054,-11.7650236480001));
#65738=CARTESIAN_POINT('Ctrl Pts',(37.1112136356493,-2.31077082721321,-11.829452684913));
#65739=CARTESIAN_POINT('Ctrl Pts',(37.1621919695941,-2.31525790427523,-11.8756601204217));
#65740=CARTESIAN_POINT('Ctrl Pts',(37.2146437318066,-2.31974498133725,-11.9201201988837));
#65741=CARTESIAN_POINT('Ctrl Pts',(37.2684320627391,-2.32423205839928,-11.9627399280164));
#65742=CARTESIAN_POINT('Ctrl Pts',(37.3443436335834,-2.3305646785489,-12.0228892305014));
#65743=CARTESIAN_POINT('Ctrl Pts',(37.4231993222627,-2.33689729869852,-12.0795937882138));
#65744=CARTESIAN_POINT('Ctrl Pts',(37.5046534682714,-2.34322991884815,-12.132552643813));
#65745=CARTESIAN_POINT('Ctrl Pts',(37.5859979900185,-2.3495540163032,-12.1854402252569));
#65746=CARTESIAN_POINT('Ctrl Pts',(37.6699336548913,-2.35587811375825,-12.2345918876808));
#65747=CARTESIAN_POINT('Ctrl Pts',(37.7560821674047,-2.3622022112133,-12.2797471654606));
#65748=CARTESIAN_POINT('Ctrl Pts',(37.8421405081474,-2.36851968922653,-12.3248551791469));
#65749=CARTESIAN_POINT('Ctrl Pts',(37.9304067065361,-2.37483716723977,-12.3659749222822));
#65750=CARTESIAN_POINT('Ctrl Pts',(38.0204748056826,-2.38115464525301,-12.4028900202875));
#65751=CARTESIAN_POINT('Ctrl Pts',(38.110478971527,-2.38746763891236,-12.439778914741));
#65752=CARTESIAN_POINT('Ctrl Pts',(38.202282091807,-2.3937806325717,-12.4724689322425));
#65753=CARTESIAN_POINT('Ctrl Pts',(38.295455869171,-2.40009362623105,-12.5007907467231));
#65754=CARTESIAN_POINT('Ctrl Pts',(38.3885959763382,-2.40640433856464,-12.529102326553));
#65755=CARTESIAN_POINT('Ctrl Pts',(38.4831053384089,-2.41271505089823,-12.5530487128777));
#65756=CARTESIAN_POINT('Ctrl Pts',(38.5785389349689,-2.41902576323182,-12.5725099339544));
#65757=CARTESIAN_POINT('Ctrl Pts',(38.6739638930162,-2.42533590432875,-12.5919693934291));
#65758=CARTESIAN_POINT('Ctrl Pts',(38.7703124906826,-2.43164604542568,-12.6069444076832));
#65759=CARTESIAN_POINT('Ctrl Pts',(38.8671289413233,-2.43795618652261,-12.6173660053744));
#65760=CARTESIAN_POINT('Ctrl Pts',(38.9639628507405,-2.44426746551855,-12.627789482378));
#65761=CARTESIAN_POINT('Ctrl Pts',(39.0612643458969,-2.4505787445145,-12.6336578652206));
#65762=CARTESIAN_POINT('Ctrl Pts',(39.1585729868944,-2.45689002351044,-12.6349540921829));
#65763=CARTESIAN_POINT('Ctrl Pts',(39.2559856929666,-2.46320805199659,-12.6362517053732));
#65764=CARTESIAN_POINT('Ctrl Pts',(39.3534051221422,-2.46952608048274,-12.6329673950012));
#65765=CARTESIAN_POINT('Ctrl Pts',(39.4503715087784,-2.4758441089689,-12.6251362486981));
#65766=CARTESIAN_POINT('Ctrl Pts',(39.5473947145845,-2.48216583961563,-12.6173005135963));
#65767=CARTESIAN_POINT('Ctrl Pts',(39.6439639156643,-2.48848757026237,-12.6049126928345));
#65768=CARTESIAN_POINT('Ctrl Pts',(39.7396272249482,-2.4948093009091,-12.5880594364123));
#65769=CARTESIAN_POINT('Ctrl Pts',(39.8354439233815,-2.50114116799052,-12.5711791570209));
#65770=CARTESIAN_POINT('Ctrl Pts',(39.9303514031963,-2.50747303507194,-12.5498192406631));
#65771=CARTESIAN_POINT('Ctrl Pts',(40.0239107121449,-2.51380490215336,-12.5241168352221));
#65772=CARTESIAN_POINT('Ctrl Pts',(40.078251497959,-2.51748255472199,-12.5091884553028));
#65773=CARTESIAN_POINT('Ctrl Pts',(40.1321377965864,-2.52116020729063,-12.4927960712961));
#65774=CARTESIAN_POINT('Ctrl Pts',(40.1854867683263,-2.52483785985926,-12.4749739799452));
#65775=CARTESIAN_POINT('Ctrl Pts',(40.2773493809841,-2.53117048000889,-12.4442857806955));
#65776=CARTESIAN_POINT('Ctrl Pts',(40.3679367385615,-2.53750310015852,-12.4092492690312));
#65777=CARTESIAN_POINT('Ctrl Pts',(40.4568078803832,-2.54383572030815,-12.3699893856932));
#65778=CARTESIAN_POINT('Ctrl Pts',(40.5455594158526,-2.55015981776323,-12.3307823398831));
#65779=CARTESIAN_POINT('Ctrl Pts',(40.6325989296655,-2.5564839152183,-12.2873633948018));
#65780=CARTESIAN_POINT('Ctrl Pts',(40.7175015292641,-2.56280801267338,-12.2399069526562));
#65781=CARTESIAN_POINT('Ctrl Pts',(40.8023152611905,-2.56912549068661,-12.1925001832364));
#65782=CARTESIAN_POINT('Ctrl Pts',(40.8849961458686,-2.57544296869985,-12.141064530598));
#65783=CARTESIAN_POINT('Ctrl Pts',(40.9651410915204,-2.58176044671308,-12.0858216610936));
#65784=CARTESIAN_POINT('Ctrl Pts',(41.0452291476511,-2.58807344037242,-12.0306180047969));
#65785=CARTESIAN_POINT('Ctrl Pts',(41.1227844844056,-2.59438643403177,-11.971612751825));
#65786=CARTESIAN_POINT('Ctrl Pts',(41.197431195838,-2.60069942769111,-11.9090719936263));
#65787=CARTESIAN_POINT('Ctrl Pts',(41.2720509321971,-2.60701014002469,-11.8465538357739));
#65788=CARTESIAN_POINT('Ctrl Pts',(41.3437637968885,-2.61332085235827,-11.7805029919129));
#65789=CARTESIAN_POINT('Ctrl Pts',(41.4122260712237,-2.61963156469185,-11.7112265350824));
#65790=CARTESIAN_POINT('Ctrl Pts',(41.4806821484518,-2.62594170578879,-11.6419563490574));
#65791=CARTESIAN_POINT('Ctrl Pts',(41.5458879130941,-2.63225184688573,-11.5694614417768));
#65792=CARTESIAN_POINT('Ctrl Pts',(41.6075364682288,-2.63856198798267,-11.4940857795049));
#65793=CARTESIAN_POINT('Ctrl Pts',(41.6691961403618,-2.64487326697859,-11.4186965248445));
#65794=CARTESIAN_POINT('Ctrl Pts',(41.7272970521219,-2.65118454597451,-11.3404258219638));
#65795=CARTESIAN_POINT('Ctrl Pts',(41.781573231189,-2.65749582497043,-11.2596499084565));
#65796=CARTESIAN_POINT('Ctrl Pts',(41.8359074549949,-2.66381385345658,-11.1787876105192));
#65797=CARTESIAN_POINT('Ctrl Pts',(41.8864085357551,-2.67013188194273,-11.0954151167484));
#65798=CARTESIAN_POINT('Ctrl Pts',(41.9328545386116,-2.67644991042888,-11.0099366059498));
#65799=CARTESIAN_POINT('Ctrl Pts',(41.9793277573254,-2.68277164107561,-10.9244080075054));
#65800=CARTESIAN_POINT('Ctrl Pts',(42.0217409761598,-2.68909337172234,-10.8367713281497));
#65801=CARTESIAN_POINT('Ctrl Pts',(42.0599197442076,-2.69541510236907,-10.7474523342821));
#65802=CARTESIAN_POINT('Ctrl Pts',(42.0981597291293,-2.70174696945048,-10.6579901239129));
#65803=CARTESIAN_POINT('Ctrl Pts',(42.1321515528492,-2.70807883653189,-10.5668406221492));
#65804=CARTESIAN_POINT('Ctrl Pts',(42.1617701208713,-2.7144107036133,-10.4744463671076));
#65805=CARTESIAN_POINT('Ctrl Pts',(42.178973072444,-2.71808835618195,-10.4207822637692));
#65806=CARTESIAN_POINT('Ctrl Pts',(42.194701662792,-2.72176600875059,-10.3666984872842));
#65807=CARTESIAN_POINT('Ctrl Pts',(42.2089393296271,-2.72544366131924,-10.3122831533337));
#65808=CARTESIAN_POINT('Ctrl Pts',(42.2334554398906,-2.73177628146887,-10.2185843512333));
#65809=CARTESIAN_POINT('Ctrl Pts',(42.2536332752531,-2.7381089016185,-10.123576554382));
#65810=CARTESIAN_POINT('Ctrl Pts',(42.2693364213388,-2.74444152176813,-10.0276973100617));
#65811=CARTESIAN_POINT('Ctrl Pts',(42.2850184334997,-2.7507656192232,-9.93194710387979));
#65812=CARTESIAN_POINT('Ctrl Pts',(42.2962376557355,-2.75708971667826,-9.83532820920002));
#65813=CARTESIAN_POINT('Ctrl Pts',(42.3029078749237,-2.76341381413333,-9.73829175473226));
#65814=CARTESIAN_POINT('Ctrl Pts',(42.3095711123839,-2.76973129214659,-9.64135686845946));
#65815=CARTESIAN_POINT('Ctrl Pts',(42.3116947829521,-2.77604877015985,-9.54400572528747));
#65816=CARTESIAN_POINT('Ctrl Pts',(42.3092441683453,-2.78236624817311,-9.4466970338322));
#65817=CARTESIAN_POINT('Ctrl Pts',(42.3067952932655,-2.78867924183245,-9.34945741529036));
#65818=CARTESIAN_POINT('Ctrl Pts',(42.2997785991763,-2.79499223549179,-9.25226062449232));
#65819=CARTESIAN_POINT('Ctrl Pts',(42.2882114288376,-2.80130522915113,-9.15556688873823));
#65820=CARTESIAN_POINT('Ctrl Pts',(42.2766484385259,-2.80761594148472,-9.05890809518778));
#65821=CARTESIAN_POINT('Ctrl Pts',(42.2605382913067,-2.8139266538183,-8.96275242924147));
#65822=CARTESIAN_POINT('Ctrl Pts',(42.2399502413291,-2.82023736615188,-8.86755556649762));
#65823=CARTESIAN_POINT('Ctrl Pts',(42.2193640549523,-2.82654750724881,-8.7723673208376));
#65824=CARTESIAN_POINT('Ctrl Pts',(42.1943008643566,-2.83285764834574,-8.67813813320795));
#65825=CARTESIAN_POINT('Ctrl Pts',(42.1648809448693,-2.83916778944267,-8.58531301187511));
#65826=CARTESIAN_POINT('Ctrl Pts',(42.1354557201285,-2.84547906843863,-8.49247115151641));
#65827=CARTESIAN_POINT('Ctrl Pts',(42.1016723382666,-2.85179034743458,-8.40103427718842));
#65828=CARTESIAN_POINT('Ctrl Pts',(42.0637004681861,-2.85810162643054,-8.31143076777195));
#65829=CARTESIAN_POINT('Ctrl Pts',(42.0256879897337,-2.86441965491668,-8.22173143340328));
#65830=CARTESIAN_POINT('Ctrl Pts',(41.9834782512849,-2.87073768340283,-8.13386978161148));
#65831=CARTESIAN_POINT('Ctrl Pts',(41.9372883909053,-2.87705571188898,-8.04825258831602));
#65832=CARTESIAN_POINT('Ctrl Pts',(41.8910714647597,-2.8833774425357,-7.96258522611139));
#65833=CARTESIAN_POINT('Ctrl Pts',(41.8408699979806,-2.88969917318242,-7.87916531581658));
#65834=CARTESIAN_POINT('Ctrl Pts',(41.78694516131,-2.89602090382914,-7.79837167135629));
#65835=CARTESIAN_POINT('Ctrl Pts',(41.732933860091,-2.90235277091055,-7.71744848017113));
#65836=CARTESIAN_POINT('Ctrl Pts',(41.675187527059,-2.90868463799196,-7.63916031521021));
#65837=CARTESIAN_POINT('Ctrl Pts',(41.6140083564293,-2.91501650507338,-7.56385382798998));
#65838=CARTESIAN_POINT('Ctrl Pts',(41.5784744876479,-2.91869415764199,-7.52011458131945));
#65839=CARTESIAN_POINT('Ctrl Pts',(41.5417832786228,-2.92237181021061,-7.47738053618639));
#65840=CARTESIAN_POINT('Ctrl Pts',(41.5039994625352,-2.92604946277923,-7.43571372724143));
#65841=CARTESIAN_POINT('Ctrl Pts',(41.4389387884715,-2.93238208292886,-7.36396685366578));
#65842=CARTESIAN_POINT('Ctrl Pts',(41.3704106033539,-2.93871470307849,-7.2951372499552));
#65843=CARTESIAN_POINT('Ctrl Pts',(41.2987067345049,-2.94504732322812,-7.22957831859948));
#65844=CARTESIAN_POINT('Ctrl Pts',(41.2270993676031,-2.95137142068317,-7.16410761908714));
#65845=CARTESIAN_POINT('Ctrl Pts',(41.1523251316917,-2.95769551813822,-7.10189913573855));
#65846=CARTESIAN_POINT('Ctrl Pts',(41.0747146678837,-2.96401961559327,-7.04327165730782));
#65847=CARTESIAN_POINT('Ctrl Pts',(40.9971854390586,-2.97033709360651,-6.9847055443422));
#65848=CARTESIAN_POINT('Ctrl Pts',(40.9168262313329,-2.97665457161975,-6.92971324681606));
#65849=CARTESIAN_POINT('Ctrl Pts',(40.8340021811452,-2.98297204963299,-6.87857457597748));
#65850=CARTESIAN_POINT('Ctrl Pts',(40.7512369221952,-2.98928504329234,-6.82747220505116));
#65851=CARTESIAN_POINT('Ctrl Pts',(40.6660106701898,-2.99559803695169,-6.78021825170862));
#65852=CARTESIAN_POINT('Ctrl Pts',(40.5787182908357,-3.00191103061104,-6.73704976238542));
#65853=CARTESIAN_POINT('Ctrl Pts',(40.4914574563183,-3.00822174294462,-6.69389687285405));
#65854=CARTESIAN_POINT('Ctrl Pts',(40.4021323696278,-3.01453245527821,-6.65482670744933));
#65855=CARTESIAN_POINT('Ctrl Pts',(40.311162460707,-3.02084316761179,-6.62003035492356));
#65856=CARTESIAN_POINT('Ctrl Pts',(40.2202007862522,-3.02715330870873,-6.58523715211385));
#65857=CARTESIAN_POINT('Ctrl Pts',(40.1275949941139,-3.03346344980566,-6.55471714905668));
#65858=CARTESIAN_POINT('Ctrl Pts',(40.0337834707486,-3.03977359090259,-6.52861287934847));
#65859=CARTESIAN_POINT('Ctrl Pts',(39.9399550304815,-3.04608486989852,-6.50250390229351));
#65860=CARTESIAN_POINT('Ctrl Pts',(39.8449208484584,-3.05239614889445,-6.48081235730437));
#65861=CARTESIAN_POINT('Ctrl Pts',(39.749132385458,-3.05870742789038,-6.46363032677509));
#65862=CARTESIAN_POINT('Ctrl Pts',(39.6532414831113,-3.06502545637653,-6.44642992121483));
#65863=CARTESIAN_POINT('Ctrl Pts',(39.5565951205009,-3.07134348486269,-6.43374873555632));
#65864=CARTESIAN_POINT('Ctrl Pts',(39.4596526160273,-3.07766151334884,-6.42562729380763));
#65865=CARTESIAN_POINT('Ctrl Pts',(39.3626533063777,-3.08398324399558,-6.41750109315645));
#65866=CARTESIAN_POINT('Ctrl Pts',(39.2653579461476,-3.09030497464232,-6.41393997281143));
#65867=CARTESIAN_POINT('Ctrl Pts',(39.1682265079734,-3.09662670528906,-6.41493230007699));
#65868=CARTESIAN_POINT('Ctrl Pts',(39.0709393266122,-3.10295857237048,-6.41592621846704));
#65869=CARTESIAN_POINT('Ctrl Pts',(38.9738170284686,-3.10929043945189,-6.42148813853957));
#65870=CARTESIAN_POINT('Ctrl Pts',(38.8773150781794,-3.1156223065333,-6.43155449472119));
#65871=CARTESIAN_POINT('Ctrl Pts',(38.8212651578643,-3.11929995910194,-6.43740119999661));
#65872=CARTESIAN_POINT('Ctrl Pts',(38.7654243506651,-3.12297761167057,-6.44476650274189));
#65873=CARTESIAN_POINT('Ctrl Pts',(38.709879987631,-3.12665526423921,-6.45363010590137));
#65874=CARTESIAN_POINT('Ctrl Pts',(38.6142370888026,-3.13298788438884,-6.46889251335247));
#65875=CARTESIAN_POINT('Ctrl Pts',(38.5191416506987,-3.13932050453847,-6.4886531852611));
#65876=CARTESIAN_POINT('Ctrl Pts',(38.4250491243567,-3.1456531246881,-6.51286092730768));
#65877=CARTESIAN_POINT('Ctrl Pts',(38.3310832315159,-3.15197722214318,-6.53703608960273));
#65878=CARTESIAN_POINT('Ctrl Pts',(38.2381179876727,-3.15830131959827,-6.56564631843693));
#65879=CARTESIAN_POINT('Ctrl Pts',(38.1466010753143,-3.16462541705335,-6.59858899701855));
#65880=CARTESIAN_POINT('Ctrl Pts',(38.0551799538386,-3.17094289506661,-6.63149719445149));
#65881=CARTESIAN_POINT('Ctrl Pts',(37.9652045593308,-3.17726037307986,-6.66872867893345));
#65882=CARTESIAN_POINT('Ctrl Pts',(37.8771087910329,-3.18357785109312,-6.71013064208345));
#65883=CARTESIAN_POINT('Ctrl Pts',(37.7890755560121,-3.18989084475246,-6.75150321675674));
#65884=CARTESIAN_POINT('Ctrl Pts',(37.7029196893523,-3.1962038384118,-6.79704019928177));
#65885=CARTESIAN_POINT('Ctrl Pts',(37.6190555304126,-3.20251683207115,-6.8465405104835));
#65886=CARTESIAN_POINT('Ctrl Pts',(37.5352216774539,-3.20882754440473,-6.89602293376374));
#65887=CARTESIAN_POINT('Ctrl Pts',(37.4536782628863,-3.21513825673832,-6.94946561780621));
#65888=CARTESIAN_POINT('Ctrl Pts',(37.3748145692308,-3.2214489690719,-7.00662179246092));
#65889=CARTESIAN_POINT('Ctrl Pts',(37.295958014204,-3.22775911016883,-7.06377279342048));
#65890=CARTESIAN_POINT('Ctrl Pts',(37.2197810517871,-3.23406925126577,-7.12463635987137));
#65891=CARTESIAN_POINT('Ctrl Pts',(37.1466426673008,-3.2403793923627,-7.1889233066634));
#65892=CARTESIAN_POINT('Ctrl Pts',(37.073491093871,-3.24669067135863,-7.25322184623148));
#65893=CARTESIAN_POINT('Ctrl Pts',(37.0033795150905,-3.25300195035456,-7.32094470350832));
#65894=CARTESIAN_POINT('Ctrl Pts',(36.936631816048,-3.25931322935049,-7.39176416756751));
#65895=CARTESIAN_POINT('Ctrl Pts',(36.8698127348115,-3.26563125783664,-7.46265936830071));
#65896=CARTESIAN_POINT('Ctrl Pts',(36.8063650158503,-3.2719492863228,-7.53665746850689));
#65897=CARTESIAN_POINT('Ctrl Pts',(36.7465736653391,-3.27826731480895,-7.61339599464424));
#65898=CARTESIAN_POINT('Ctrl Pts',(36.6867472790282,-3.28458904545566,-7.69017948707857));
#65899=CARTESIAN_POINT('Ctrl Pts',(36.6305817796637,-3.29091077610238,-7.7697062459808));
#65900=CARTESIAN_POINT('Ctrl Pts',(36.5783188559795,-3.29723250674909,-7.85158474012361));
#65901=CARTESIAN_POINT('Ctrl Pts',(36.5259721325032,-3.30356437383051,-7.93359452046888));
#65902=CARTESIAN_POINT('Ctrl Pts',(36.477540697407,-3.30989624091193,-8.01796318672667));
#65903=CARTESIAN_POINT('Ctrl Pts',(36.4332202876357,-3.31622810799334,-8.10427459509259));
#65904=CARTESIAN_POINT('Ctrl Pts',(36.4074782645102,-3.31990576056196,-8.15440568101024));
#65905=CARTESIAN_POINT('Ctrl Pts',(36.3831221919925,-3.32358341313057,-8.2051917535564));
#65906=CARTESIAN_POINT('Ctrl Pts',(36.3601828105059,-3.32726106569919,-8.25654858857189));
#65907=CARTESIAN_POINT('Ctrl Pts',(36.3160477270097,-3.33433682331197,-8.35535849775967));
#65908=CARTESIAN_POINT('Ctrl Pts',(36.2770243650611,-3.34141258092474,-8.45658489155548));
#65909=CARTESIAN_POINT('Ctrl Pts',(36.243357954337,-3.34848833853752,-8.55970291271675));
#65910=CARTESIAN_POINT('Ctrl Pts',(36.2105182027539,-3.3553903550361,-8.66028893082336));
#65911=CARTESIAN_POINT('Ctrl Pts',(36.1827755450531,-3.36229237153469,-8.76267446198814));
#65912=CARTESIAN_POINT('Ctrl Pts',(36.1603110343668,-3.36919438803328,-8.86634861640778));
#65913=CARTESIAN_POINT('Ctrl Pts',(36.1369982913306,-3.37635701620315,-8.97393737964616));
#65914=CARTESIAN_POINT('Ctrl Pts',(36.1193703286723,-3.38351964437303,-9.08291374571453));
#65915=CARTESIAN_POINT('Ctrl Pts',(36.1075742388077,-3.3906822725429,-9.19268454081396));
#65916=CARTESIAN_POINT('Ctrl Pts',(36.0957781489431,-3.39784490071277,-9.30245533591338));
#65917=CARTESIAN_POINT('Ctrl Pts',(36.0898140999805,-3.40500752888264,-9.41302021472769));
#65918=CARTESIAN_POINT('Ctrl Pts',(36.0897702438652,-3.41217015705251,-9.52376835315984));
#65919=CARTESIAN_POINT('',(36.0897712316907,-4.68217015708684,-9.52776797424251));
#65920=CARTESIAN_POINT('Ctrl Pts',(36.089770243865,-3.41217015708684,-9.52376835369061));
#65921=CARTESIAN_POINT('Ctrl Pts',(36.0897308469584,-3.41860450524517,-9.6232558691197));
#65922=CARTESIAN_POINT('Ctrl Pts',(36.0944692869388,-3.4250388534035,-9.72271952248611));
#65923=CARTESIAN_POINT('Ctrl Pts',(36.1039523828961,-3.43147320156183,-9.82168131981128));
#65924=CARTESIAN_POINT('Ctrl Pts',(36.1134403070674,-3.43791082569778,-9.92069350244754));
#65925=CARTESIAN_POINT('Ctrl Pts',(36.1276776560797,-3.44434844983373,-10.0192029096662));
#65926=CARTESIAN_POINT('Ctrl Pts',(36.1465795645642,-3.45078607396968,-10.1167383690139));
#65927=CARTESIAN_POINT('Ctrl Pts',(36.165510976694,-3.45723374647609,-10.2144260696866));
#65928=CARTESIAN_POINT('Ctrl Pts',(36.1891214144015,-3.4636814189825,-10.3111363793427));
#65929=CARTESIAN_POINT('Ctrl Pts',(36.2172751014949,-3.4701290914889,-10.4064095715034));
#65930=CARTESIAN_POINT('Ctrl Pts',(36.2454507957173,-3.47658180400162,-10.5017572366603));
#65931=CARTESIAN_POINT('Ctrl Pts',(36.2781766812073,-3.48303451651434,-10.5956651556457));
#65932=CARTESIAN_POINT('Ctrl Pts',(36.3152681542323,-3.48948722902706,-10.6876920619465));
#65933=CARTESIAN_POINT('Ctrl Pts',(36.3524368379709,-3.49595337369811,-10.7799105341933));
#65934=CARTESIAN_POINT('Ctrl Pts',(36.393989101499,-3.50241951836916,-10.8702397909493));
#65935=CARTESIAN_POINT('Ctrl Pts',(36.4396932262027,-3.50888566304022,-10.9582610255738));
#65936=CARTESIAN_POINT('Ctrl Pts',(36.4844143268592,-3.51521273107987,-11.0443890614801));
#65937=CARTESIAN_POINT('Ctrl Pts',(36.5331102241574,-3.52153979911952,-11.1283070947645));
#65938=CARTESIAN_POINT('Ctrl Pts',(36.5855244989187,-3.52786686715917,-11.2096508561555));
#65939=CARTESIAN_POINT('Ctrl Pts',(36.6379847680988,-3.5341994873088,-11.2910659980827));
#65940=CARTESIAN_POINT('Ctrl Pts',(36.6943426987631,-3.54053210745842,-11.3701697916308));
#65941=CARTESIAN_POINT('Ctrl Pts',(36.7543681441278,-3.54686472760805,-11.4465658922981));
#65942=CARTESIAN_POINT('Ctrl Pts',(36.814312804837,-3.55318882506311,-11.5228591760244));
#65943=CARTESIAN_POINT('Ctrl Pts',(36.8779149020383,-3.55951292251816,-11.5964516687685));
#65944=CARTESIAN_POINT('Ctrl Pts',(36.9449003400655,-3.56583701997322,-11.666974831006));
#65945=CARTESIAN_POINT('Ctrl Pts',(37.0118156643394,-3.57215449798647,-11.7374241765492));
#65946=CARTESIAN_POINT('Ctrl Pts',(37.0821069894798,-3.57847197599972,-11.8048102631216));
#65947=CARTESIAN_POINT('Ctrl Pts',(37.1554598181657,-3.58478945401297,-11.8687973670445));
#65948=CARTESIAN_POINT('Ctrl Pts',(37.2287605785984,-3.59110244767231,-11.9327390508142));
#65949=CARTESIAN_POINT('Ctrl Pts',(37.305118193598,-3.59741544133165,-11.9932862618891));
#65950=CARTESIAN_POINT('Ctrl Pts',(37.3841818472024,-3.60372843499099,-12.0501406077426));
#65951=CARTESIAN_POINT('Ctrl Pts',(37.4632169295839,-3.61003914732457,-12.1069744081481));
#65952=CARTESIAN_POINT('Ctrl Pts',(37.5449557528238,-3.61634985965815,-12.1601177399249));
#65953=CARTESIAN_POINT('Ctrl Pts',(37.6290157560935,-3.62266057199173,-12.2093135357661));
#65954=CARTESIAN_POINT('Ctrl Pts',(37.7130681503719,-3.62897071308866,-12.2585048784743));
#65955=CARTESIAN_POINT('Ctrl Pts',(37.7994409294023,-3.63528085418559,-12.3037491749849));
#65956=CARTESIAN_POINT('Ctrl Pts',(37.8877248953068,-3.64159099528252,-12.3448341622341));
#65957=CARTESIAN_POINT('Ctrl Pts',(37.9760247813366,-3.64790227427845,-12.3859265582821));
#65958=CARTESIAN_POINT('Ctrl Pts',(38.0662361422508,-3.65421355327439,-12.4228579709121));
#65959=CARTESIAN_POINT('Ctrl Pts',(38.1579286363547,-3.66052483227032,-12.4554637731885));
#65960=CARTESIAN_POINT('Ctrl Pts',(38.2497191894404,-3.66684286075647,-12.4881044451869));
#65961=CARTESIAN_POINT('Ctrl Pts',(38.3429936253149,-3.67316088924262,-12.5164101246133));
#65962=CARTESIAN_POINT('Ctrl Pts',(38.4373054240797,-3.67947891772876,-12.5402657655275));
#65963=CARTESIAN_POINT('Ctrl Pts',(38.5316724865116,-3.68580064837548,-12.5641353850765));
#65964=CARTESIAN_POINT('Ctrl Pts',(38.6270776939102,-3.6921223790222,-12.5835496865475));
#65965=CARTESIAN_POINT('Ctrl Pts',(38.7230653569237,-3.69844410966892,-12.5984449725241));
#65966=CARTESIAN_POINT('Ctrl Pts',(38.8192069291644,-3.70477597675033,-12.613364142007));
#65967=CARTESIAN_POINT('Ctrl Pts',(38.9159323873655,-3.71110784383175,-12.6237497805225));
#65968=CARTESIAN_POINT('Ctrl Pts',(39.012782002131,-3.71743971091316,-12.6295901620301));
#65969=CARTESIAN_POINT('Ctrl Pts',(39.069033851694,-3.72111736348183,-12.6329823516918));
#65970=CARTESIAN_POINT('Ctrl Pts',(39.1253275853489,-3.72479501605049,-12.6348421862075));
#65971=CARTESIAN_POINT('Ctrl Pts',(39.1815737290658,-3.72847266861915,-12.6351754171492));
#65972=CARTESIAN_POINT('Ctrl Pts',(39.2784250374454,-3.73480528876879,-12.6357492138678));
#65973=CARTESIAN_POINT('Ctrl Pts',(39.375471400899,-3.74113790891842,-12.6317957542547));
#65974=CARTESIAN_POINT('Ctrl Pts',(39.4722551252913,-3.74747052906806,-12.623291109572));
#65975=CARTESIAN_POINT('Ctrl Pts',(39.5689085942595,-3.75379462652311,-12.6147979107817));
#65976=CARTESIAN_POINT('Ctrl Pts',(39.6652996947494,-3.76011872397817,-12.6017657389353));
#65977=CARTESIAN_POINT('Ctrl Pts',(39.7609699927092,-3.76644282143322,-12.5842226660019));
#65978=CARTESIAN_POINT('Ctrl Pts',(39.8565401524318,-3.77276029944646,-12.566697955428));
#65979=CARTESIAN_POINT('Ctrl Pts',(39.9513905816555,-3.77907777745969,-12.5446718089296));
#65980=CARTESIAN_POINT('Ctrl Pts',(40.0450682414024,-3.78539525547293,-12.5182240678361));
#65981=CARTESIAN_POINT('Ctrl Pts',(40.1386794056622,-3.79170824913227,-12.4917951002199));
#65982=CARTESIAN_POINT('Ctrl Pts',(40.2311190357782,-3.79802124279162,-12.4609508962037));
#65983=CARTESIAN_POINT('Ctrl Pts',(40.321945500733,-3.80433423645096,-12.4258221155881));
#65984=CARTESIAN_POINT('Ctrl Pts',(40.412739143739,-3.81064494878454,-12.3907060294557));
#65985=CARTESIAN_POINT('Ctrl Pts',(40.5019203724547,-3.81695566111812,-12.3513086008371));
#65986=CARTESIAN_POINT('Ctrl Pts',(40.5890648084925,-3.8232663734517,-12.307809661243));
#65987=CARTESIAN_POINT('Ctrl Pts',(40.6762013563408,-3.82957651454865,-12.2643146591107));
#65988=CARTESIAN_POINT('Ctrl Pts',(40.761301086895,-3.83588665564559,-12.216719079654));
#65989=CARTESIAN_POINT('Ctrl Pts',(40.8439625796973,-3.84219679674253,-12.1652495506022));
#65990=CARTESIAN_POINT('Ctrl Pts',(40.9266389787322,-3.84850807573848,-12.1137707401214));
#65991=CARTESIAN_POINT('Ctrl Pts',(41.0068758955392,-3.85481935473442,-12.0584168237454));
#65992=CARTESIAN_POINT('Ctrl Pts',(41.0843002416636,-3.86113063373037,-11.9994581734526));
#65993=CARTESIAN_POINT('Ctrl Pts',(41.1618073879408,-3.86744866221652,-11.9404364708319));
#65994=CARTESIAN_POINT('Ctrl Pts',(41.236495610022,-3.87376669070267,-11.8778026033331));
#65995=CARTESIAN_POINT('Ctrl Pts',(41.3080244943481,-3.88008471918883,-11.8118675921724));
#65996=CARTESIAN_POINT('Ctrl Pts',(41.3795952922897,-3.88640644983557,-11.7458939452252));
#65997=CARTESIAN_POINT('Ctrl Pts',(41.4480027589633,-3.89272818048231,-11.6766156138095));
#65998=CARTESIAN_POINT('Ctrl Pts',(41.5129444669172,-3.89904991112905,-11.6043793655457));
#65999=CARTESIAN_POINT('Ctrl Pts',(41.5779903041701,-3.90538177821047,-11.5320272917188));
#66000=CARTESIAN_POINT('Ctrl Pts',(41.6395590095688,-3.91171364529189,-11.4567081688672));
#66001=CARTESIAN_POINT('Ctrl Pts',(41.6973894671656,-3.91804551237331,-11.3788005562061));
#66002=CARTESIAN_POINT('Ctrl Pts',(41.7309783483266,-3.92172316494192,-11.3335505330877));
#66003=CARTESIAN_POINT('Ctrl Pts',(41.7633069582748,-3.92540081751053,-11.2874278227167));
#66004=CARTESIAN_POINT('Ctrl Pts',(41.794331205074,-3.92907847007914,-11.2405104929085));
#66005=CARTESIAN_POINT('Ctrl Pts',(41.8477524477669,-3.93541109022877,-11.1597226472469));
#66006=CARTESIAN_POINT('Ctrl Pts',(41.8974892705568,-3.9417437103784,-11.0762967821856));
#66007=CARTESIAN_POINT('Ctrl Pts',(41.9432714516952,-3.94807633052803,-10.9906030824252));
#66008=CARTESIAN_POINT('Ctrl Pts',(41.9889920173352,-3.95440042798309,-10.9050247126882));
#66009=CARTESIAN_POINT('Ctrl Pts',(42.0307683153435,-3.96072452543815,-10.8171849569883));
#66010=CARTESIAN_POINT('Ctrl Pts',(42.0683732639495,-3.96704862289321,-10.7274830441881));
#66011=CARTESIAN_POINT('Ctrl Pts',(42.1059388514021,-3.97336610090644,-10.6378750225079));
#66012=CARTESIAN_POINT('Ctrl Pts',(42.1393416013967,-3.97968357891967,-10.546409119865));
#66013=CARTESIAN_POINT('Ctrl Pts',(42.1684007319163,-3.98600105693291,-10.4535083454977));
#66014=CARTESIAN_POINT('Ctrl Pts',(42.1974392353083,-3.99231405059225,-10.3606735151586));
#66015=CARTESIAN_POINT('Ctrl Pts',(42.2221401187166,-3.99862704425159,-10.2664062541597));
#66016=CARTESIAN_POINT('Ctrl Pts',(42.2423713903786,-4.00494003791094,-10.1711477972613));
#66017=CARTESIAN_POINT('Ctrl Pts',(42.2625953510684,-4.01125075024452,-10.0759237639));
#66018=CARTESIAN_POINT('Ctrl Pts',(42.2783528186387,-4.0175614625781,-9.97970967370127));
#66019=CARTESIAN_POINT('Ctrl Pts',(42.2895624074209,-4.02387217491168,-9.88295919257854));
#66020=CARTESIAN_POINT('Ctrl Pts',(42.3007709815272,-4.03018231600861,-9.78621746917095));
#66021=CARTESIAN_POINT('Ctrl Pts',(42.3074324452119,-4.03649245710554,-9.68893988580377));
#66022=CARTESIAN_POINT('Ctrl Pts',(42.3095171483323,-4.04280259820247,-9.59158646354242));
#66023=CARTESIAN_POINT('Ctrl Pts',(42.3116022273844,-4.04911387719839,-9.49421548567346));
#66024=CARTESIAN_POINT('Ctrl Pts',(42.3091088973539,-4.05542515619432,-9.39676907895592));
#66025=CARTESIAN_POINT('Ctrl Pts',(42.3020596255315,-4.06173643519024,-9.29970745119377));
#66026=CARTESIAN_POINT('Ctrl Pts',(42.2950028149849,-4.06805446367639,-9.20254202252081));
#66027=CARTESIAN_POINT('Ctrl Pts',(42.2833803671463,-4.07437249216254,-9.10576263121383));
#66028=CARTESIAN_POINT('Ctrl Pts',(42.2672666489418,-4.08069052064869,-9.00982434336522));
#66029=CARTESIAN_POINT('Ctrl Pts',(42.2511434886192,-4.08701225129541,-8.9138298387795));
#66030=CARTESIAN_POINT('Ctrl Pts',(42.230523909995,-4.09333398194213,-8.81867784627415));
#66031=CARTESIAN_POINT('Ctrl Pts',(42.2055329772973,-4.09965571258885,-8.72481116273821));
#66032=CARTESIAN_POINT('Ctrl Pts',(42.1805019734591,-4.10598757967026,-8.63079397081134));
#66033=CARTESIAN_POINT('Ctrl Pts',(42.1510857516613,-4.11231944675168,-8.53806661968593));
#66034=CARTESIAN_POINT('Ctrl Pts',(42.1174585794742,-4.1186513138331,-8.44705469064864));
#66035=CARTESIAN_POINT('Ctrl Pts',(42.0979273646554,-4.12232896640177,-8.39419346499427));
#66036=CARTESIAN_POINT('Ctrl Pts',(42.076976489609,-4.12600661897045,-8.34191053978871));
#66037=CARTESIAN_POINT('Ctrl Pts',(42.0546472253936,-4.12968427153912,-8.2902855101471));
#66038=CARTESIAN_POINT('Ctrl Pts',(42.0161980391651,-4.13601689168875,-8.20139138629269));
#66039=CARTESIAN_POINT('Ctrl Pts',(41.9735258507318,-4.14234951183837,-8.11414053622946));
#66040=CARTESIAN_POINT('Ctrl Pts',(41.9267929375975,-4.14868213198799,-8.02896158860526));
#66041=CARTESIAN_POINT('Ctrl Pts',(41.8801229194947,-4.15500622944307,-7.94389727822993));
#66042=CARTESIAN_POINT('Ctrl Pts',(41.8294032473786,-4.16133032689815,-7.86089970828239));
#66043=CARTESIAN_POINT('Ctrl Pts',(41.7748441009242,-4.16765442435323,-7.78037725887913));
#66044=CARTESIAN_POINT('Ctrl Pts',(41.7203420616064,-4.17397190236645,-7.69993909243891));
#66045=CARTESIAN_POINT('Ctrl Pts',(41.6620087814985,-4.18028938037968,-7.6219712562158));
#66046=CARTESIAN_POINT('Ctrl Pts',(41.6000996618428,-4.1866068583929,-7.54685635857203));
#66047=CARTESIAN_POINT('Ctrl Pts',(41.5382344873185,-4.19291985205224,-7.47179477995561));
#66048=CARTESIAN_POINT('Ctrl Pts',(41.4727987967841,-4.19923284571157,-7.39958245038754));
#66049=CARTESIAN_POINT('Ctrl Pts',(41.404089922872,-4.20554583937091,-7.33057108458848));
#66050=CARTESIAN_POINT('Ctrl Pts',(41.3354058782774,-4.21185655170449,-7.26158465741842));
#66051=CARTESIAN_POINT('Ctrl Pts',(41.2634513088352,-4.21816726403806,-7.19579720516986));
#66052=CARTESIAN_POINT('Ctrl Pts',(41.188561619043,-4.22447797637164,-7.13352486105981));
#66053=CARTESIAN_POINT('Ctrl Pts',(41.1136787081582,-4.23078811746858,-7.07125815375307));
#66054=CARTESIAN_POINT('Ctrl Pts',(41.0358615415469,-4.23709825856552,-7.01250620140424));
#66055=CARTESIAN_POINT('Ctrl Pts',(40.9554791250099,-4.24340839966246,-6.95754528870432));
#66056=CARTESIAN_POINT('Ctrl Pts',(40.8750822132234,-4.24971967865839,-6.90257446497931));
#66057=CARTESIAN_POINT('Ctrl Pts',(40.7921194937645,-4.25603095765431,-6.85139628548057));
#66058=CARTESIAN_POINT('Ctrl Pts',(40.7069886171799,-4.26234223665024,-6.80424349479959));
#66059=CARTESIAN_POINT('Ctrl Pts',(40.6217666988239,-4.26866026513638,-6.75704027736681));
#66060=CARTESIAN_POINT('Ctrl Pts',(40.5343723773683,-4.27497829362253,-6.71387125545519));
#66061=CARTESIAN_POINT('Ctrl Pts',(40.4452273671073,-4.28129632210867,-6.67492290330472));
#66062=CARTESIAN_POINT('Ctrl Pts',(40.3560301207502,-4.2876180527554,-6.63595172867815));
#66063=CARTESIAN_POINT('Ctrl Pts',(40.2650805511827,-4.29393978340213,-6.60120630457832));
#66064=CARTESIAN_POINT('Ctrl Pts',(40.1728178107986,-4.30026151404886,-6.57082394568417));
#66065=CARTESIAN_POINT('Ctrl Pts',(40.0804071338296,-4.30659338113028,-6.54039287089023));
#66066=CARTESIAN_POINT('Ctrl Pts',(39.9866795026542,-4.3129252482117,-6.5143389478488));
#66067=CARTESIAN_POINT('Ctrl Pts',(39.8920865491162,-4.31925711529312,-6.49274887889666));
#66068=CARTESIAN_POINT('Ctrl Pts',(39.8371454055193,-4.32293476786178,-6.48020901166344));
#66069=CARTESIAN_POINT('Ctrl Pts',(39.7819125069031,-4.32661242043044,-6.46917405159658));
#66070=CARTESIAN_POINT('Ctrl Pts',(39.7264770642849,-4.3302900729991,-6.45965294726977));
#66071=CARTESIAN_POINT('Ctrl Pts',(39.6310217176002,-4.33662269314873,-6.44325837600969));
#66072=CARTESIAN_POINT('Ctrl Pts',(39.5346340451537,-4.34295531329836,-6.43129831318331));
#66073=CARTESIAN_POINT('Ctrl Pts',(39.4377616765962,-4.34928793344799,-6.4238711671325));
#66074=CARTESIAN_POINT('Ctrl Pts',(39.3410196827633,-4.35561203090306,-6.41645401683317));
#66075=CARTESIAN_POINT('Ctrl Pts',(39.2437947216939,-4.36193612835813,-6.41355769126737));
#66076=CARTESIAN_POINT('Ctrl Pts',(39.1465436515253,-4.3682602258132,-6.41522941815514));
#66077=CARTESIAN_POINT('Ctrl Pts',(39.0493943741911,-4.37457770382642,-6.41689939524398));
#66078=CARTESIAN_POINT('Ctrl Pts',(38.9522194770394,-4.38089518183964,-6.42312791168205));
#66079=CARTESIAN_POINT('Ctrl Pts',(38.8554789563812,-4.38721265985286,-6.43391024015739));
#66080=CARTESIAN_POINT('Ctrl Pts',(38.7588071053295,-4.3935256535122,-6.444684914981));
#66081=CARTESIAN_POINT('Ctrl Pts',(38.6625694511726,-4.39983864717155,-6.46000692724261));
#66082=CARTESIAN_POINT('Ctrl Pts',(38.5672230409478,-4.40615164083089,-6.47981955001142));
#66083=CARTESIAN_POINT('Ctrl Pts',(38.4719110860439,-4.41246235316447,-6.49962501309511));
#66084=CARTESIAN_POINT('Ctrl Pts',(38.3774901628507,-4.41877306549805,-6.52391777334063));
#66085=CARTESIAN_POINT('Ctrl Pts',(38.2844083339141,-4.42508377783163,-6.55258977361906));
#66086=CARTESIAN_POINT('Ctrl Pts',(38.1913349306115,-4.43139391892856,-6.58125917854902));
#66087=CARTESIAN_POINT('Ctrl Pts',(38.0996007984381,-4.43770406002549,-6.61430690643706));
#66088=CARTESIAN_POINT('Ctrl Pts',(38.0096389986286,-4.44401420112242,-6.65157498108719));
#66089=CARTESIAN_POINT('Ctrl Pts',(37.9196609761319,-4.45032548011838,-6.68884977623781));
#66090=CARTESIAN_POINT('Ctrl Pts',(37.8314563247676,-4.45663675911435,-6.73034626228963));
#66091=CARTESIAN_POINT('Ctrl Pts',(37.7454373038562,-4.46294803811032,-6.77585867662521));
#66092=CARTESIAN_POINT('Ctrl Pts',(37.6593262913632,-4.46926606659647,-6.82141976343968));
#66093=CARTESIAN_POINT('Ctrl Pts',(37.5754059629639,-4.47558409508262,-6.87100514794837));
#66094=CARTESIAN_POINT('Ctrl Pts',(37.494062985742,-4.48190212356877,-6.92436362474789));
#66095=CARTESIAN_POINT('Ctrl Pts',(37.4126723441633,-4.48822385421551,-6.97775336789099));
#66096=CARTESIAN_POINT('Ctrl Pts',(37.3338624149043,-4.49454558486224,-7.03492034918793));
#66097=CARTESIAN_POINT('Ctrl Pts',(37.2579882317365,-4.50086731550897,-7.09557188934801));
#66098=CARTESIAN_POINT('Ctrl Pts',(37.1819923898418,-4.5071991825904,-7.15632067983559));
#66099=CARTESIAN_POINT('Ctrl Pts',(37.1089420217795,-4.51353104967182,-7.22056489729979));
#66100=CARTESIAN_POINT('Ctrl Pts',(37.0391566009855,-4.51986291675324,-7.28797374672638));
#66101=CARTESIAN_POINT('Ctrl Pts',(36.9986240805244,-4.52354056932185,-7.32712591543949));
#66102=CARTESIAN_POINT('Ctrl Pts',(36.9591922626734,-4.52721822189046,-7.36734500511245));
#66103=CARTESIAN_POINT('Ctrl Pts',(36.9209174052313,-4.53089587445908,-7.40856120354915));
#66104=CARTESIAN_POINT('Ctrl Pts',(36.8553184770402,-4.53719896956857,-7.47920126917562));
#66105=CARTESIAN_POINT('Ctrl Pts',(36.7928785099401,-4.54350206467806,-7.55303258751636));
#66106=CARTESIAN_POINT('Ctrl Pts',(36.7339284141938,-4.54980515978755,-7.62973706663706));
#66107=CARTESIAN_POINT('Ctrl Pts',(36.6754872120085,-4.55605384269508,-7.70577938541652));
#66108=CARTESIAN_POINT('Ctrl Pts',(36.6204761746455,-4.56230252560262,-7.78464511883583));
#66109=CARTESIAN_POINT('Ctrl Pts',(36.569181482799,-4.56855120851016,-7.86598686489461));
#66110=CARTESIAN_POINT('Ctrl Pts',(36.5179349658241,-4.57479402278907,-7.94725221653455));
#66111=CARTESIAN_POINT('Ctrl Pts',(36.4703981015631,-4.58103683706799,-8.03098858612567));
#66112=CARTESIAN_POINT('Ctrl Pts',(36.4268156026728,-4.5872796513469,-8.11681714563738));
#66113=CARTESIAN_POINT('Ctrl Pts',(36.3832615433595,-4.59351839190352,-8.20258969808233));
#66114=CARTESIAN_POINT('Ctrl Pts',(36.3436569259494,-4.59975713246014,-8.29045132955641));
#66115=CARTESIAN_POINT('Ctrl Pts',(36.308201449891,-4.60599587301677,-8.37999703123199));
#66116=CARTESIAN_POINT('Ctrl Pts',(36.272125852573,-4.61234373002261,-8.4711088998159));
#66117=CARTESIAN_POINT('Ctrl Pts',(36.2403461461278,-4.61869158702844,-8.56396389225379));
#66118=CARTESIAN_POINT('Ctrl Pts',(36.2130219718117,-4.62503944403428,-8.65811309156248));
#66119=CARTESIAN_POINT('Ctrl Pts',(36.1861721018347,-4.63127711230808,-8.75062801006035));
#66120=CARTESIAN_POINT('Ctrl Pts',(36.1636244051878,-4.63751478058188,-8.84439210881212));
#66121=CARTESIAN_POINT('Ctrl Pts',(36.1454798590326,-4.64375244885568,-8.93896470983034));
#66122=CARTESIAN_POINT('Ctrl Pts',(36.1268545263607,-4.65015540022754,-9.03604325566669));
#66123=CARTESIAN_POINT('Ctrl Pts',(36.1128690938145,-4.6565583515994,-9.13397326884296));
#66124=CARTESIAN_POINT('Ctrl Pts',(36.1035763459161,-4.66296130297126,-9.23226939461385));
#66125=CARTESIAN_POINT('Ctrl Pts',(36.0942835980177,-4.66936425434312,-9.33056552038474));
#66126=CARTESIAN_POINT('Ctrl Pts',(36.0896835345435,-4.67576720571498,-9.42922724870747));
#66127=CARTESIAN_POINT('Ctrl Pts',(36.0897712316907,-4.68217015708684,-9.52776797424251));
#66128=CARTESIAN_POINT('',(36.0897047610518,-5.95217015708685,-9.52350960940354));
#66129=CARTESIAN_POINT('Ctrl Pts',(36.0901415350687,-4.68217037744286,-9.52777103554189));
#66130=CARTESIAN_POINT('Ctrl Pts',(36.0878821773097,-4.69861414360159,-9.78081088334408));
#66131=CARTESIAN_POINT('Ctrl Pts',(36.23139618657,-4.78192651024699,-11.0603082092272));
#66132=CARTESIAN_POINT('Ctrl Pts',(37.9960327313695,-4.93210747737905,-12.9917445733203));
#66133=CARTESIAN_POINT('Ctrl Pts',(41.4448765000052,-5.13271327883904,-12.4281680317038));
#66134=CARTESIAN_POINT('Ctrl Pts',(42.8581511280529,-5.33331908029901,-9.23210847586989));
#66135=CARTESIAN_POINT('Ctrl Pts',(40.9543526129433,-5.53392488175898,-6.30163188108486));
#66136=CARTESIAN_POINT('Ctrl Pts',(37.4597734733276,-5.73453068321898,-6.29398363414102));
#66137=CARTESIAN_POINT('Ctrl Pts',(36.1277880032688,-5.87394577499493,-8.32476719916938));
#66138=CARTESIAN_POINT('Ctrl Pts',(36.0851544239569,-5.94649226628422,-9.4364601111202));
#66139=CARTESIAN_POINT('Ctrl Pts',(36.0856727518626,-5.95217015708685,-9.52350767734625));
#66140=CARTESIAN_POINT('',(36.0897702898568,-7.22217015705017,-9.52365722578339));
#66141=CARTESIAN_POINT('Ctrl Pts',(36.089770357075,-5.95217015708685,-9.52350964083583));
#66142=CARTESIAN_POINT('Ctrl Pts',(36.089724436915,-5.95842920731442,-9.61934039494398));
#66143=CARTESIAN_POINT('Ctrl Pts',(36.0941117716707,-5.96468825754199,-9.71534736715066));
#66144=CARTESIAN_POINT('Ctrl Pts',(36.1029549177913,-5.97094730776956,-9.81108112777174));
#66145=CARTESIAN_POINT('Ctrl Pts',(36.1117869597681,-5.97719849864555,-9.90669467761718));
#66146=CARTESIAN_POINT('Ctrl Pts',(36.1250636570616,-5.98344968952154,-10.0020352547221));
#66147=CARTESIAN_POINT('Ctrl Pts',(36.142755544866,-5.98970088039753,-10.0966528618423));
#66148=CARTESIAN_POINT('Ctrl Pts',(36.1604303082252,-5.99594602058086,-10.1911788860831));
#66149=CARTESIAN_POINT('Ctrl Pts',(36.182511685981,-6.0021911607642,-10.2849828927258));
#66150=CARTESIAN_POINT('Ctrl Pts',(36.2089184721355,-6.00843630094753,-10.3776206346128));
#66151=CARTESIAN_POINT('Ctrl Pts',(36.235311544599,-6.01467819787661,-10.4702102674514));
#66152=CARTESIAN_POINT('Ctrl Pts',(36.2660254427374,-6.02092009480568,-10.5616344080258));
#66153=CARTESIAN_POINT('Ctrl Pts',(36.3009282168457,-6.02716199173475,-10.6514605847604));
#66154=CARTESIAN_POINT('Ctrl Pts',(36.335822844769,-6.03340243182698,-10.7412657963805));
#66155=CARTESIAN_POINT('Ctrl Pts',(36.3749042442181,-6.03964287191921,-10.8294733674587));
#66156=CARTESIAN_POINT('Ctrl Pts',(36.4179915011379,-6.04588331201144,-10.9156686755511));
#66157=CARTESIAN_POINT('Ctrl Pts',(36.4610810214978,-6.05212407992361,-11.001868511616));
#66158=CARTESIAN_POINT('Ctrl Pts',(36.5081766155351,-6.05836484783578,-11.0860554744702));
#66159=CARTESIAN_POINT('Ctrl Pts',(36.5590509280406,-6.06460561574796,-11.1678385959116));
#66160=CARTESIAN_POINT('Ctrl Pts',(36.6099747976654,-6.07085246284753,-11.2497013830173));
#66161=CARTESIAN_POINT('Ctrl Pts',(36.6646844987986,-6.07709930994711,-11.3291552714969));
#66162=CARTESIAN_POINT('Ctrl Pts',(36.7229089329688,-6.08334615704669,-11.4058377119077));
#66163=CARTESIAN_POINT('Ctrl Pts',(36.781162413407,-6.0895961204942,-11.4825584066829));
#66164=CARTESIAN_POINT('Ctrl Pts',(36.8429338296361,-6.09584608394171,-11.5565045573239));
#66165=CARTESIAN_POINT('Ctrl Pts',(36.9079127702298,-6.10209604738921,-11.6273479217352));
#66166=CARTESIAN_POINT('Ctrl Pts',(36.972999067908,-6.10835633691849,-11.6983083323309));
#66167=CARTESIAN_POINT('Ctrl Pts',(37.041303155336,-6.11461662644778,-11.766155402873));
#66168=CARTESIAN_POINT('Ctrl Pts',(37.1124789097127,-6.12087691597706,-11.8305989136244));
#66169=CARTESIAN_POINT('Ctrl Pts',(37.1688157042764,-6.12583203936435,-11.8816070252764));
#66170=CARTESIAN_POINT('Ctrl Pts',(37.226950855291,-6.13078716275165,-11.9304835512479));
#66171=CARTESIAN_POINT('Ctrl Pts',(37.2866998353367,-6.13574228613894,-11.9771038177042));
#66172=CARTESIAN_POINT('Ctrl Pts',(37.3630586997653,-6.14207490628857,-12.0366842591316));
#66173=CARTESIAN_POINT('Ctrl Pts',(37.4423358620394,-6.1484075264382,-12.092798054621));
#66174=CARTESIAN_POINT('Ctrl Pts',(37.5241834226642,-6.15474014658783,-12.145146837875));
#66175=CARTESIAN_POINT('Ctrl Pts',(37.6059208295544,-6.1610642440429,-12.1974251680338));
#66176=CARTESIAN_POINT('Ctrl Pts',(37.6902213938912,-6.16738834149797,-12.2459483234262));
#66177=CARTESIAN_POINT('Ctrl Pts',(37.7767048846497,-6.17371243895304,-12.2904586721772));
#66178=CARTESIAN_POINT('Ctrl Pts',(37.8630978530149,-6.18002991696628,-12.3349224318826));
#66179=CARTESIAN_POINT('Ctrl Pts',(37.951668818572,-6.18634739497951,-12.3753815360964));
#66180=CARTESIAN_POINT('Ctrl Pts',(38.0420102190963,-6.19266487299274,-12.4116226494335));
#66181=CARTESIAN_POINT('Ctrl Pts',(38.1322874923201,-6.19897786665208,-12.4478380376352));
#66182=CARTESIAN_POINT('Ctrl Pts',(38.2243322973688,-6.20529086031143,-12.479841224991));
#66183=CARTESIAN_POINT('Ctrl Pts',(38.3177150837064,-6.21160385397077,-12.5074660902315));
#66184=CARTESIAN_POINT('Ctrl Pts',(38.4110641243177,-6.21791456630435,-12.5350809726778));
#66185=CARTESIAN_POINT('Ctrl Pts',(38.5057497665624,-6.22422527863793,-12.5583205529172));
#66186=CARTESIAN_POINT('Ctrl Pts',(38.6013261060655,-6.23053599097151,-12.5770681875773));
#66187=CARTESIAN_POINT('Ctrl Pts',(38.6968937941349,-6.23684613206844,-12.5958141252283));
#66188=CARTESIAN_POINT('Ctrl Pts',(38.7933515899888,-6.24315627316536,-12.6100688417519));
#66189=CARTESIAN_POINT('Ctrl Pts',(38.8902432043774,-6.24946641426229,-12.619766773194));
#66190=CARTESIAN_POINT('Ctrl Pts',(38.9871522910966,-6.25577769325822,-12.6294664534506));
#66191=CARTESIAN_POINT('Ctrl Pts',(39.0844949165885,-6.26208897225415,-12.6346076730712));
#66192=CARTESIAN_POINT('Ctrl Pts',(39.1818105263284,-6.26840025125008,-12.6351768110427));
#66193=CARTESIAN_POINT('Ctrl Pts',(39.2792302085957,-6.27471827973623,-12.6357465576691));
#66194=CARTESIAN_POINT('Ctrl Pts',(39.3766223794049,-6.28103630822238,-12.6317344583957));
#66195=CARTESIAN_POINT('Ctrl Pts',(39.4735275481078,-6.28735433670852,-12.6231790350666));
#66196=CARTESIAN_POINT('Ctrl Pts',(39.570489500109,-6.29367606735526,-12.6146185985358));
#66197=CARTESIAN_POINT('Ctrl Pts',(39.6669634486199,-6.29999779800199,-12.601509595556));
#66198=CARTESIAN_POINT('Ctrl Pts',(39.7624981666,-6.30631952864872,-12.5839420500349));
#66199=CARTESIAN_POINT('Ctrl Pts',(39.8581860675425,-6.31265139573014,-12.566346336234));
#66200=CARTESIAN_POINT('Ctrl Pts',(39.9529313051179,-6.31898326281155,-12.5442779038389));
#66201=CARTESIAN_POINT('Ctrl Pts',(40.0462959640472,-6.32531512989297,-12.5178771765873));
#66202=CARTESIAN_POINT('Ctrl Pts',(40.100523693928,-6.32899278246162,-12.502543199872));
#66203=CARTESIAN_POINT('Ctrl Pts',(40.1542860108318,-6.33267043503027,-12.4857486556877));
#66204=CARTESIAN_POINT('Ctrl Pts',(40.2075003336219,-6.33634808759892,-12.4675284587667));
#66205=CARTESIAN_POINT('Ctrl Pts',(40.2991310916823,-6.34268070774852,-12.4361547539378));
#66206=CARTESIAN_POINT('Ctrl Pts',(40.3894541413373,-6.34901332789811,-12.4004423862849));
#66207=CARTESIAN_POINT('Ctrl Pts',(40.4780294677295,-6.35534594804771,-12.3605195877502));
#66208=CARTESIAN_POINT('Ctrl Pts',(40.5664855858895,-6.36167004550275,-12.3206505189214));
#66209=CARTESIAN_POINT('Ctrl Pts',(40.6531982604861,-6.36799414295779,-12.2765824599564));
#66210=CARTESIAN_POINT('Ctrl Pts',(40.7377439138879,-6.37431824041282,-12.2284929828281));
#66211=CARTESIAN_POINT('Ctrl Pts',(40.8222010732339,-6.38063571842606,-12.1804538410239));
#66212=CARTESIAN_POINT('Ctrl Pts',(40.904495342597,-6.38695319643929,-12.1284018642748));
#66213=CARTESIAN_POINT('Ctrl Pts',(40.9842252976564,-6.39327067445252,-12.0725617244932));
#66214=CARTESIAN_POINT('Ctrl Pts',(41.0638986577684,-6.39958366811184,-12.0167612218815));
#66215=CARTESIAN_POINT('Ctrl Pts',(41.1410109651289,-6.40589666177116,-11.9571781522152));
#66216=CARTESIAN_POINT('Ctrl Pts',(41.2151883124176,-6.41220965543048,-11.8940814081402));
#66217=CARTESIAN_POINT('Ctrl Pts',(41.2893388542473,-6.41852036776404,-11.8310074653279));
#66218=CARTESIAN_POINT('Ctrl Pts',(41.3605562106748,-6.4248310800976,-11.7644226541438));
#66219=CARTESIAN_POINT('Ctrl Pts',(41.4284989669377,-6.43114179243116,-11.6946366071897));
#66220=CARTESIAN_POINT('Ctrl Pts',(41.4964355731195,-6.43745193352806,-11.6248568771686));
#66221=CARTESIAN_POINT('Ctrl Pts',(41.5610978635619,-6.44376207462497,-11.5518768009912));
#66222=CARTESIAN_POINT('Ctrl Pts',(41.6221815198935,-6.45007221572188,-11.4760426283366));
#66223=CARTESIAN_POINT('Ctrl Pts',(41.6832761913563,-6.45638349471781,-11.4001947806105));
#66224=CARTESIAN_POINT('Ctrl Pts',(41.7407906727067,-6.46269477371374,-11.3214921547849));
#66225=CARTESIAN_POINT('Ctrl Pts',(41.7944618101514,-6.46900605270968,-11.2403129651949));
#66226=CARTESIAN_POINT('Ctrl Pts',(41.8481903452831,-6.47532408119581,-11.1590469598985));
#66227=CARTESIAN_POINT('Ctrl Pts',(41.8980670891438,-6.48164210968194,-11.0752994686089));
#66228=CARTESIAN_POINT('Ctrl Pts',(41.9438731329391,-6.48796013816807,-10.9894763170619));
#66229=CARTESIAN_POINT('Ctrl Pts',(41.9897060175962,-6.49428186881478,-10.9036028759207));
#66230=CARTESIAN_POINT('Ctrl Pts',(42.0314632649294,-6.5006035994615,-10.8156517474713));
#66231=CARTESIAN_POINT('Ctrl Pts',(42.0689736100634,-6.50692533010821,-10.726049989659));
#66232=CARTESIAN_POINT('Ctrl Pts',(42.1065441003039,-6.5132571971896,-10.6363045619539));
#66233=CARTESIAN_POINT('Ctrl Pts',(42.1398539411277,-6.519589064271,-10.544903630581));
#66234=CARTESIAN_POINT('Ctrl Pts',(42.1687813480053,-6.52592093135239,-10.4522906559626));
#66235=CARTESIAN_POINT('Ctrl Pts',(42.1855828618157,-6.52959858392123,-10.3984995166929));
#66236=CARTESIAN_POINT('Ctrl Pts',(42.2009069199183,-6.53327623649006,-10.3442997318519));
#66237=CARTESIAN_POINT('Ctrl Pts',(42.2147376188538,-6.5369538890589,-10.2897795384083));
#66238=CARTESIAN_POINT('Ctrl Pts',(42.2385529633224,-6.54328650920859,-10.1959001767492));
#66239=CARTESIAN_POINT('Ctrl Pts',(42.2580203736777,-6.54961912935828,-10.1007442708017));
#66240=CARTESIAN_POINT('Ctrl Pts',(42.2730067085367,-6.55595174950798,-10.0047503748703));
#66241=CARTESIAN_POINT('Ctrl Pts',(42.2879728741844,-6.5622758469631,-9.90888567138002));
#66242=CARTESIAN_POINT('Ctrl Pts',(42.2984698839692,-6.56859994441823,-9.81218564789262));
#66243=CARTESIAN_POINT('Ctrl Pts',(42.3044148978359,-6.57492404187336,-9.71510206467697));
#66244=CARTESIAN_POINT('Ctrl Pts',(42.3103536890481,-6.58124151988664,-9.6181200989866));
#66245=CARTESIAN_POINT('Ctrl Pts',(42.3117499299689,-6.58755899789992,-9.52075580591713));
#66246=CARTESIAN_POINT('Ctrl Pts',(42.3085723305793,-6.59387647591321,-9.42346814068221));
#66247=CARTESIAN_POINT('Ctrl Pts',(42.3053969867545,-6.6001894695726,-9.3262495334352));
#66248=CARTESIAN_POINT('Ctrl Pts',(42.2976542714137,-6.60650246323199,-9.22910788172664));
#66249=CARTESIAN_POINT('Ctrl Pts',(42.2853649654746,-6.61281545689138,-9.13250327043195));
#66250=CARTESIAN_POINT('Ctrl Pts',(42.2730801005206,-6.61912616922502,-9.03593356913402));
#66251=CARTESIAN_POINT('Ctrl Pts',(42.2562519647596,-6.62543688155865,-8.93990095600729));
#66252=CARTESIAN_POINT('Ctrl Pts',(42.2349532150411,-6.63174759389229,-8.84486057649043));
#66253=CARTESIAN_POINT('Ctrl Pts',(42.2136563932548,-6.63805773498928,-8.74982879989265));
#66254=CARTESIAN_POINT('Ctrl Pts',(42.1878898579292,-6.64436787608626,-8.65578950501199));
#66255=CARTESIAN_POINT('Ctrl Pts',(42.1577772059652,-6.65067801718325,-8.56318678904235));
#66256=CARTESIAN_POINT('Ctrl Pts',(42.1276591238284,-6.65698929617926,-8.47056737415298));
#66257=CARTESIAN_POINT('Ctrl Pts',(42.0931935037355,-6.66330057517527,-8.37938546855403));
#66258=CARTESIAN_POINT('Ctrl Pts',(42.0545532105356,-6.66961185417127,-8.29006817146812));
#66259=CARTESIAN_POINT('Ctrl Pts',(42.01587159413,-6.67592988265748,-8.20065535551486));
#66260=CARTESIAN_POINT('Ctrl Pts',(41.9730065653444,-6.68224791114369,-8.11311153115883));
#66261=CARTESIAN_POINT('Ctrl Pts',(41.926178295457,-6.6885659396299,-8.02784184059294));
#66262=CARTESIAN_POINT('Ctrl Pts',(41.8793225857162,-6.6948876702767,-7.94252218474294));
#66263=CARTESIAN_POINT('Ctrl Pts',(41.8284992386597,-6.70120940092349,-7.85947968902788));
#66264=CARTESIAN_POINT('Ctrl Pts',(41.7739722480919,-6.70753113157029,-7.77909120543114));
#66265=CARTESIAN_POINT('Ctrl Pts',(41.7193578274659,-6.71386299865176,-7.69857382475574));
#66266=CARTESIAN_POINT('Ctrl Pts',(41.6610281671869,-6.72019486573324,-7.62071930347723));
#66267=CARTESIAN_POINT('Ctrl Pts',(41.5992880430821,-6.72652673281471,-7.54587202555684));
#66268=CARTESIAN_POINT('Ctrl Pts',(41.5634283632996,-6.73020438538277,-7.50239949520928));
#66269=CARTESIAN_POINT('Ctrl Pts',(41.5264188860586,-6.73388203795083,-7.45994078554279));
#66270=CARTESIAN_POINT('Ctrl Pts',(41.4883248062323,-6.73755969051889,-7.41855744581492));
#66271=CARTESIAN_POINT('Ctrl Pts',(41.4227298831058,-6.74389231066848,-7.34729868328411));
#66272=CARTESIAN_POINT('Ctrl Pts',(41.3536893424341,-6.75022493081807,-7.27898301710029));
#66273=CARTESIAN_POINT('Ctrl Pts',(41.281497643882,-6.75655755096766,-7.213961659467));
#66274=CARTESIAN_POINT('Ctrl Pts',(41.2094031038176,-6.76288164842269,-7.14902781018855));
#66275=CARTESIAN_POINT('Ctrl Pts',(41.134166157167,-6.76920574587772,-7.08737974764538));
#66276=CARTESIAN_POINT('Ctrl Pts',(41.0561198176812,-6.77552984333275,-7.0293337812698));
#66277=CARTESIAN_POINT('Ctrl Pts',(40.9781551694107,-6.78184732134592,-6.97134857169034));
#66278=CARTESIAN_POINT('Ctrl Pts',(40.8973873234095,-6.78816479935909,-6.91695822231062));
#66279=CARTESIAN_POINT('Ctrl Pts',(40.8141834965666,-6.79448227737226,-6.86643980840906));
#66280=CARTESIAN_POINT('Ctrl Pts',(40.7310387305391,-6.80079527103157,-6.81595725414076));
#66281=CARTESIAN_POINT('Ctrl Pts',(40.6454617940483,-6.80710826469087,-6.76934139763099));
#66282=CARTESIAN_POINT('Ctrl Pts',(40.5578493128993,-6.81342125835017,-6.72682632841368));
#66283=CARTESIAN_POINT('Ctrl Pts',(40.470268492262,-6.81973197068373,-6.68432662286175));
#66284=CARTESIAN_POINT('Ctrl Pts',(40.3806539816182,-6.82604268301728,-6.64592495077549));
#66285=CARTESIAN_POINT('Ctrl Pts',(40.2894266269451,-6.83235339535084,-6.61180926175386));
#66286=CARTESIAN_POINT('Ctrl Pts',(40.1982075300416,-6.83866353644774,-6.57769666083561));
#66287=CARTESIAN_POINT('Ctrl Pts',(40.1053762890547,-6.84497367754465,-6.54786942460858));
#66288=CARTESIAN_POINT('Ctrl Pts',(40.0113723431609,-6.85128381864155,-6.52246680723534));
#66289=CARTESIAN_POINT('Ctrl Pts',(39.9173514456657,-6.85759509763746,-6.49705960904328));
#66290=CARTESIAN_POINT('Ctrl Pts',(39.8221578454268,-6.86390637663337,-6.47607872845315));
#66291=CARTESIAN_POINT('Ctrl Pts',(39.7262436786258,-6.87021765562928,-6.45961287214707));
#66292=CARTESIAN_POINT('Ctrl Pts',(39.6302269380468,-6.8765356841154,-6.44312940671043));
#66293=CARTESIAN_POINT('Ctrl Pts',(39.5334885241675,-6.88285371260151,-6.43117067953997));
#66294=CARTESIAN_POINT('Ctrl Pts',(39.4364880453472,-6.88917174108763,-6.42377378166186));
#66295=CARTESIAN_POINT('Ctrl Pts',(39.3394307273799,-6.89549347173433,-6.41637254944056));
#66296=CARTESIAN_POINT('Ctrl Pts',(39.2421114756232,-6.90181520238103,-6.41353848207697));
#66297=CARTESIAN_POINT('Ctrl Pts',(39.1449901629594,-6.90813693302774,-6.41525651046123));
#66298=CARTESIAN_POINT('Ctrl Pts',(39.047713123344,-6.91446880010912,-6.41697729357889));
#66299=CARTESIAN_POINT('Ctrl Pts',(38.9506350926986,-6.92080066719052,-6.42326471892864));
#66300=CARTESIAN_POINT('Ctrl Pts',(38.8542110480094,-6.9271325342719,-6.43405181965449));
#66301=CARTESIAN_POINT('Ctrl Pts',(38.7982063765427,-6.93081018684089,-6.44031714521905));
#66302=CARTESIAN_POINT('Ctrl Pts',(38.7424221587324,-6.93448783940988,-6.44809946345234));
#66303=CARTESIAN_POINT('Ctrl Pts',(38.6869455715382,-6.93816549197887,-6.4573778253612));
#66304=CARTESIAN_POINT('Ctrl Pts',(38.5914193772331,-6.94449811212838,-6.47335441381708));
#66305=CARTESIAN_POINT('Ctrl Pts',(38.4964742376763,-6.95083073227788,-6.49382505075428));
#66306=CARTESIAN_POINT('Ctrl Pts',(38.402565208688,-6.95716335242738,-6.51873514032692));
#66307=CARTESIAN_POINT('Ctrl Pts',(38.3087825662435,-6.9634874498823,-6.54361170490033));
#66308=CARTESIAN_POINT('Ctrl Pts',(38.21603368198,-6.96981154733722,-6.57291573575188));
#66309=CARTESIAN_POINT('Ctrl Pts',(38.1247654591753,-6.97613564479213,-6.6065412740425));
#66310=CARTESIAN_POINT('Ctrl Pts',(38.0335927669488,-6.98245312280528,-6.64013161643452));
#66311=CARTESIAN_POINT('Ctrl Pts',(37.9438980632769,-6.98877060081842,-6.67803432328299));
#66312=CARTESIAN_POINT('Ctrl Pts',(37.8561140935644,-6.99508807883156,-6.72009334854371));
#66313=CARTESIAN_POINT('Ctrl Pts',(37.7683924358044,-7.00140107249077,-6.76212251892326));
#66314=CARTESIAN_POINT('Ctrl Pts',(37.6825792088593,-7.00771406614998,-6.80830195393796));
#66315=CARTESIAN_POINT('Ctrl Pts',(37.5990872381363,-7.01402705980919,-6.85842748424088));
#66316=CARTESIAN_POINT('Ctrl Pts',(37.5156254388967,-7.02033777214265,-6.90853490068697));
#66317=CARTESIAN_POINT('Ctrl Pts',(37.4344836036633,-7.0266484844761,-6.96258535407638));
#66318=CARTESIAN_POINT('Ctrl Pts',(37.3560491603192,-7.03295919680955,-7.02032917257765));
#66319=CARTESIAN_POINT('Ctrl Pts',(37.2776218167489,-7.03926933790634,-7.07806776419099));
#66320=CARTESIAN_POINT('Ctrl Pts',(37.2019017298573,-7.04557947900313,-7.13949879677973));
#66321=CARTESIAN_POINT('Ctrl Pts',(37.1292457142642,-7.05188962009993,-7.20433041106518));
#66322=CARTESIAN_POINT('Ctrl Pts',(37.0565765967122,-7.05820089909575,-7.26917371634608));
#66323=CARTESIAN_POINT('Ctrl Pts',(36.9869729741417,-7.06451217809156,-7.33741853007999));
#66324=CARTESIAN_POINT('Ctrl Pts',(36.9207562740704,-7.07082345708738,-7.40873473054285));
#66325=CARTESIAN_POINT('Ctrl Pts',(36.8544687596731,-7.0771414855734,-7.48012719890586));
#66326=CARTESIAN_POINT('Ctrl Pts',(36.7915756971201,-7.08345951405943,-7.55459729060612));
#66327=CARTESIAN_POINT('Ctrl Pts',(36.7323593763675,-7.08977754254545,-7.6317804127628));
#66328=CARTESIAN_POINT('Ctrl Pts',(36.6731083567639,-7.09609927319207,-7.70900876173575));
#66329=CARTESIAN_POINT('Ctrl Pts',(36.6175386185544,-7.10242100383869,-7.78895294786212));
#66330=CARTESIAN_POINT('Ctrl Pts',(36.5658889183557,-7.1087427344853,-7.87121964503795));
#66331=CARTESIAN_POINT('Ctrl Pts',(36.5141564016244,-7.11507460156659,-7.95361825087106));
#66332=CARTESIAN_POINT('Ctrl Pts',(36.4663566886759,-7.12140646864787,-8.03834642324154));
#66333=CARTESIAN_POINT('Ctrl Pts',(36.4226824017246,-7.12773833572916,-8.12498656748948));
#66334=CARTESIAN_POINT('Ctrl Pts',(36.3973156573532,-7.13141598829906,-8.17530858863417));
#66335=CARTESIAN_POINT('Ctrl Pts',(36.3733397187133,-7.13509364086896,-8.22627522283438));
#66336=CARTESIAN_POINT('Ctrl Pts',(36.3507846960796,-7.13877129343886,-8.27780201860111));
#66337=CARTESIAN_POINT('Ctrl Pts',(36.3081456435135,-7.14572369706949,-8.37521064411829));
#66338=CARTESIAN_POINT('Ctrl Pts',(36.2704600196826,-7.15267610070013,-8.47491220946225));
#66339=CARTESIAN_POINT('Ctrl Pts',(36.2379556849738,-7.15962850433076,-8.57640939878109));
#66340=CARTESIAN_POINT('Ctrl Pts',(36.205535236877,-7.16656296532109,-8.67764464594909));
#66341=CARTESIAN_POINT('Ctrl Pts',(36.1782695210843,-7.17349742631141,-8.78066600847023));
#66342=CARTESIAN_POINT('Ctrl Pts',(36.1563385086826,-7.18043188730174,-8.8849567364844));
#66343=CARTESIAN_POINT('Ctrl Pts',(36.1343381803525,-7.18738826559314,-8.98957708943827));
#66344=CARTESIAN_POINT('Ctrl Pts',(36.1177065160083,-7.19434464388455,-9.09547459308052));
#66345=CARTESIAN_POINT('Ctrl Pts',(36.1065761150675,-7.20130102217595,-9.20210788020016));
#66346=CARTESIAN_POINT('Ctrl Pts',(36.0954457141266,-7.20825740046736,-9.30874116731979));
#66347=CARTESIAN_POINT('Ctrl Pts',(36.0898167210575,-7.21521377875877,-9.41610995679598));
#66348=CARTESIAN_POINT('Ctrl Pts',(36.0897702898568,-7.22217015705017,-9.52365722578337));
#66349=CARTESIAN_POINT('',(36.0897712258121,-8.49217015713119,-9.52776136080223));
#66350=CARTESIAN_POINT('Ctrl Pts',(36.0897702898566,-7.22217015708685,-9.52365722635048));
#66351=CARTESIAN_POINT('Ctrl Pts',(36.0897274329479,-7.228591033366,-9.62292550639579));
#66352=CARTESIAN_POINT('Ctrl Pts',(36.0944413978688,-7.23501190964515,-9.7221767087338));
#66353=CARTESIAN_POINT('Ctrl Pts',(36.1038809221781,-7.2414327859243,-9.82093463610625));
#66354=CARTESIAN_POINT('Ctrl Pts',(36.113324596391,-7.24785648501707,-9.91973598048454));
#66355=CARTESIAN_POINT('Ctrl Pts',(36.1274979248913,-7.25428018410984,-10.0180432047192));
#66356=CARTESIAN_POINT('Ctrl Pts',(36.1463179296204,-7.26070388320261,-10.1153867088123));
#66357=CARTESIAN_POINT('Ctrl Pts',(36.1655258423147,-7.26725998417729,-10.2147366056314));
#66358=CARTESIAN_POINT('Ctrl Pts',(36.1895740108885,-7.27381608515198,-10.3130821696095));
#66359=CARTESIAN_POINT('Ctrl Pts',(36.2183201842394,-7.28037218612667,-10.4099384889276));
#66360=CARTESIAN_POINT('Ctrl Pts',(36.2465490334199,-7.28681030167575,-10.5050517548516));
#66361=CARTESIAN_POINT('Ctrl Pts',(36.2793079921364,-7.29324841722484,-10.5987285623426));
#66362=CARTESIAN_POINT('Ctrl Pts',(36.3164133193158,-7.29968653277392,-10.6905292822921));
#66363=CARTESIAN_POINT('Ctrl Pts',(36.3545386393298,-7.30630162646141,-10.7848535233554));
#66364=CARTESIAN_POINT('Ctrl Pts',(36.3972525535177,-7.31291672014889,-10.8771966020305));
#66365=CARTESIAN_POINT('Ctrl Pts',(36.4443055470847,-7.31953181383638,-10.9671091273103));
#66366=CARTESIAN_POINT('Ctrl Pts',(36.4913585406517,-7.32614690752387,-11.0570216525902));
#66367=CARTESIAN_POINT('Ctrl Pts',(36.542750316339,-7.33276200121135,-11.1445032562025));
#66368=CARTESIAN_POINT('Ctrl Pts',(36.5981845410128,-7.33937709489884,-11.2291381898999));
#66369=CARTESIAN_POINT('Ctrl Pts',(36.6512516485568,-7.34570971504808,-11.310159096297));
#66370=CARTESIAN_POINT('Ctrl Pts',(36.7081990392816,-7.35204233519732,-11.3888395970014));
#66371=CARTESIAN_POINT('Ctrl Pts',(36.7687936114938,-7.35837495534656,-11.4647850781431));
#66372=CARTESIAN_POINT('Ctrl Pts',(36.8293066330968,-7.36469905280125,-11.5406283488058));
#66373=CARTESIAN_POINT('Ctrl Pts',(36.8934568098284,-7.37102315025593,-11.6137435769121));
#66374=CARTESIAN_POINT('Ctrl Pts',(36.9609673000875,-7.37734724771062,-11.6837642811624));
#66375=CARTESIAN_POINT('Ctrl Pts',(37.0284071270201,-7.38366472572347,-11.7537116946416));
#66376=CARTESIAN_POINT('Ctrl Pts',(37.09919997309,-7.38998220373633,-11.8205707104724));
#66377=CARTESIAN_POINT('Ctrl Pts',(37.1730288413559,-7.39629968174919,-11.8840079641504));
#66378=CARTESIAN_POINT('Ctrl Pts',(37.2468053034605,-7.40261267540816,-11.9474001879773));
#66379=CARTESIAN_POINT('Ctrl Pts',(37.3236131726091,-7.40892566906713,-12.0073751942156));
#66380=CARTESIAN_POINT('Ctrl Pts',(37.4030994131577,-7.4152386627261,-12.0636372198299));
#66381=CARTESIAN_POINT('Ctrl Pts',(37.4825569297732,-7.42154937505932,-12.1198789140429));
#66382=CARTESIAN_POINT('Ctrl Pts',(37.5646905380128,-7.42786008739254,-12.1724100413258));
#66383=CARTESIAN_POINT('Ctrl Pts',(37.649115767018,-7.43417079972576,-12.2209763998945));
#66384=CARTESIAN_POINT('Ctrl Pts',(37.7335333539723,-7.44048094082234,-12.2695383623059));
#66385=CARTESIAN_POINT('Ctrl Pts',(37.8202417700958,-7.44679108191891,-12.3141360516697));
#66386=CARTESIAN_POINT('Ctrl Pts',(37.9088302429844,-7.45310122301548,-12.3545602682163));
#66387=CARTESIAN_POINT('Ctrl Pts',(37.9974346909096,-7.45941250201106,-12.3949917744059));
#66388=CARTESIAN_POINT('Ctrl Pts',(38.0879194710936,-7.46572378100665,-12.4312481315165));
#66389=CARTESIAN_POINT('Ctrl Pts',(38.1798530238244,-7.47203506000223,-12.4631679325559));
#66390=CARTESIAN_POINT('Ctrl Pts',(38.2718848933332,-7.47835308848803,-12.4951218696848));
#66391=CARTESIAN_POINT('Ctrl Pts',(38.3653682148109,-7.48467111697383,-12.5227298482419));
#66392=CARTESIAN_POINT('Ctrl Pts',(38.4598556212435,-7.49098914545963,-12.5458801617236));
#66393=CARTESIAN_POINT('Ctrl Pts',(38.5543983942439,-7.49731087610601,-12.5690440405411));
#66394=CARTESIAN_POINT('Ctrl Pts',(38.6499459948069,-7.50363260675241,-12.5877449690213));
#66395=CARTESIAN_POINT('Ctrl Pts',(38.746042270378,-7.50995433739879,-12.6019226562617));
#66396=CARTESIAN_POINT('Ctrl Pts',(38.8422926293284,-7.51628620447987,-12.616123076391));
#66397=CARTESIAN_POINT('Ctrl Pts',(38.9390929851383,-7.52261807156095,-12.6257857295259));
#66398=CARTESIAN_POINT('Ctrl Pts',(39.0359835336316,-7.52894993864204,-12.6309023248744));
#66399=CARTESIAN_POINT('Ctrl Pts',(39.092259158235,-7.53262759121429,-12.6338741276308));
#66400=CARTESIAN_POINT('Ctrl Pts',(39.148565216592,-7.53630524378655,-12.6353133050688));
#66401=CARTESIAN_POINT('Ctrl Pts',(39.2048122801432,-7.53998289635881,-12.6352262771155));
#66402=CARTESIAN_POINT('Ctrl Pts',(39.3016651722967,-7.54631551650768,-12.635076422022));
#66403=CARTESIAN_POINT('Ctrl Pts',(39.3986792881586,-7.55264813665654,-12.6303979795902));
#66404=CARTESIAN_POINT('Ctrl Pts',(39.495396767583,-7.5589807568054,-12.621170441465));
#66405=CARTESIAN_POINT('Ctrl Pts',(39.5919840807385,-7.5653048542597,-12.6119553221313));
#66406=CARTESIAN_POINT('Ctrl Pts',(39.6882751192754,-7.57162895171399,-12.598203316755));
#66407=CARTESIAN_POINT('Ctrl Pts',(39.7838116716812,-7.57795304916828,-12.579945921765));
#66408=CARTESIAN_POINT('Ctrl Pts',(39.8792482258414,-7.58427052718075,-12.5617076368164));
#66409=CARTESIAN_POINT('Ctrl Pts',(39.9739314365919,-7.59058800519322,-12.5389734191424));
#66410=CARTESIAN_POINT('Ctrl Pts',(40.0674088741442,-7.5969054832057,-12.5118264927772));
#66411=CARTESIAN_POINT('Ctrl Pts',(40.1608199583334,-7.60321847686426,-12.4846988361942));
#66412=CARTESIAN_POINT('Ctrl Pts',(40.253026552129,-7.60953147052282,-12.4531648197075));
#66413=CARTESIAN_POINT('Ctrl Pts',(40.3435880130806,-7.61584446418138,-12.4173583991681));
#66414=CARTESIAN_POINT('Ctrl Pts',(40.4341167478479,-7.62215517651418,-12.3815649179906));
#66415=CARTESIAN_POINT('Ctrl Pts',(40.5230011247852,-7.62846588884698,-12.3415022611731));
#66416=CARTESIAN_POINT('Ctrl Pts',(40.6098181209827,-7.63477660117978,-12.2973534259991));
#66417=CARTESIAN_POINT('Ctrl Pts',(40.6966272586301,-7.64108674227594,-12.2532085871144));
#66418=CARTESIAN_POINT('Ctrl Pts',(40.781368997898,-7.64739688337209,-12.2049785036821));
#66419=CARTESIAN_POINT('Ctrl Pts',(40.863643622809,-7.65370702446825,-12.152892796365));
#66420=CARTESIAN_POINT('Ctrl Pts',(40.9459330841891,-7.66001830346341,-12.1007976965044));
#66421=CARTESIAN_POINT('Ctrl Pts',(41.0257541781318,-7.66632958245858,-12.0448458257896));
#66422=CARTESIAN_POINT('Ctrl Pts',(41.1027358467116,-7.67264086145374,-11.9853103362256));
#66423=CARTESIAN_POINT('Ctrl Pts',(41.1797998420304,-7.67895888993911,-11.9257111774428));
#66424=CARTESIAN_POINT('Ctrl Pts',(41.254018003129,-7.68527691842448,-11.8625210165279));
#66425=CARTESIAN_POINT('Ctrl Pts',(41.3250522497817,-7.69159494690984,-11.7960534094552));
#66426=CARTESIAN_POINT('Ctrl Pts',(41.3961281202081,-7.6979166775558,-11.729546854512));
#66427=CARTESIAN_POINT('Ctrl Pts',(41.4640160563314,-7.70423840820175,-11.6597593425411));
#66428=CARTESIAN_POINT('Ctrl Pts',(41.5284162300564,-7.7105601388477,-11.5870398911054));
#66429=CARTESIAN_POINT('Ctrl Pts',(41.5929196647699,-7.71689200592834,-11.5142038393253));
#66430=CARTESIAN_POINT('Ctrl Pts',(41.6539238960357,-7.72322387300899,-11.4384268011343));
#66431=CARTESIAN_POINT('Ctrl Pts',(41.7111706436439,-7.72955574008963,-11.3600892761391));
#66432=CARTESIAN_POINT('Ctrl Pts',(41.7444204965151,-7.73323339266602,-11.3145895527626));
#66433=CARTESIAN_POINT('Ctrl Pts',(41.7764035929619,-7.7369110452424,-11.2682265827518));
#66434=CARTESIAN_POINT('Ctrl Pts',(41.8070764255713,-7.74058869781879,-11.2210787611814));
#66435=CARTESIAN_POINT('Ctrl Pts',(41.8598925613776,-7.74692131797149,-11.1398940274875));
#66436=CARTESIAN_POINT('Ctrl Pts',(41.9090046698514,-7.7532539381242,-11.0560988765982));
#66437=CARTESIAN_POINT('Ctrl Pts',(41.9541453026649,-7.7595865582769,-10.9700655018749));
#66438=CARTESIAN_POINT('Ctrl Pts',(41.9992251834015,-7.76591065573503,-10.8841479143231));
#66439=CARTESIAN_POINT('Ctrl Pts',(42.0403440103906,-7.77223475319315,-10.7959984739827));
#66440=CARTESIAN_POINT('Ctrl Pts',(42.0772776910847,-7.77855885065128,-10.7060180952409));
#66441=CARTESIAN_POINT('Ctrl Pts',(42.1141727132427,-7.78487632866761,-10.6161318990894));
#66442=CARTESIAN_POINT('Ctrl Pts',(42.1468911327621,-7.79119380668394,-10.5244189769566));
#66443=CARTESIAN_POINT('Ctrl Pts',(42.1752553332348,-7.79751128470027,-10.4313036770077));
#66444=CARTESIAN_POINT('Ctrl Pts',(42.2035993998641,-7.80382427836268,-10.3382544733648));
#66445=CARTESIAN_POINT('Ctrl Pts',(42.2275952650091,-7.8101372720251,-10.2438052880763));
#66446=CARTESIAN_POINT('Ctrl Pts',(42.2471142373284,-7.81645026568751,-10.1483983297787));
#66447=CARTESIAN_POINT('Ctrl Pts',(42.2666261560789,-7.82276097802417,-10.053025848682));
#66448=CARTESIAN_POINT('Ctrl Pts',(42.2816643090541,-7.82907169036082,-9.9566967103053));
#66449=CARTESIAN_POINT('Ctrl Pts',(42.2921507024747,-7.83538240269748,-9.85986517598162));
#66450=CARTESIAN_POINT('Ctrl Pts',(42.3026361466819,-7.84169254379746,-9.76304240671011));
#66451=CARTESIAN_POINT('Ctrl Pts',(42.3085706036467,-7.84800268489745,-9.66571776670031));
#66452=CARTESIAN_POINT('Ctrl Pts',(42.3099278611548,-7.85431282599744,-9.56835148571194));
#66453=CARTESIAN_POINT('Ctrl Pts',(42.3112853634152,-7.86062410499642,-9.47096764679713));
#66454=CARTESIAN_POINT('Ctrl Pts',(42.3080640208104,-7.86693538399541,-9.37354258925499));
#66455=CARTESIAN_POINT('Ctrl Pts',(42.3002897384998,-7.87324666299439,-9.27653634017716));
#66456=CARTESIAN_POINT('Ctrl Pts',(42.2925071421151,-7.87956469148354,-9.17942634941327));
#66457=CARTESIAN_POINT('Ctrl Pts',(42.2801619201976,-7.8858827199727,-9.08273649793021));
#66458=CARTESIAN_POINT('Ctrl Pts',(42.263331837677,-7.89220074846185,-8.98692128347737));
#66459=CARTESIAN_POINT('Ctrl Pts',(42.2464918932718,-7.89852247911156,-8.89104992440469));
#66460=CARTESIAN_POINT('Ctrl Pts',(42.2251619509961,-7.90484420976127,-8.79605464940832));
#66461=CARTESIAN_POINT('Ctrl Pts',(42.1994703799956,-7.91116594041098,-8.70237730858601));
#66462=CARTESIAN_POINT('Ctrl Pts',(42.1737376144323,-7.91749780749531,-8.6085497629711));
#66463=CARTESIAN_POINT('Ctrl Pts',(42.1436293905051,-7.92382967457964,-8.51604478682144));
#66464=CARTESIAN_POINT('Ctrl Pts',(42.1093231507,-7.93016154166398,-8.42528664748446));
#66465=CARTESIAN_POINT('Ctrl Pts',(42.0893975224111,-7.93383919420225,-8.37257282752336));
#66466=CARTESIAN_POINT('Ctrl Pts',(42.0680565943838,-7.93751684674051,-8.32044789901571));
#66467=CARTESIAN_POINT('Ctrl Pts',(42.0453422312277,-7.94119449927878,-8.26899114649144));
#66468=CARTESIAN_POINT('Ctrl Pts',(42.0062299354827,-7.94752711942473,-8.18038678153596));
#66469=CARTESIAN_POINT('Ctrl Pts',(41.9629070333242,-7.95385973957068,-8.09345719715179));
#66470=CARTESIAN_POINT('Ctrl Pts',(41.9155390002746,-7.96019235971662,-8.00862979754696));
#66471=CARTESIAN_POINT('Ctrl Pts',(41.8682347170265,-7.96651645716803,-7.92391656206355));
#66472=CARTESIAN_POINT('Ctrl Pts',(41.8168963346975,-7.97284055461945,-7.84130026677639));
#66473=CARTESIAN_POINT('Ctrl Pts',(41.7617370783549,-7.97916465207086,-7.76118771002079));
#66474=CARTESIAN_POINT('Ctrl Pts',(41.7066355572845,-7.98548213008046,-7.68115900719233));
#66475=CARTESIAN_POINT('Ctrl Pts',(41.6477213597273,-7.99179960809007,-7.6036291911841));
#66476=CARTESIAN_POINT('Ctrl Pts',(41.5852527384994,-7.99811708609968,-7.52897895141828));
#66477=CARTESIAN_POINT('Ctrl Pts',(41.5228284595552,-8.00443007975542,-7.45438170085015));
#66478=CARTESIAN_POINT('Ctrl Pts',(41.4568550527625,-8.01074307341117,-7.38266029732104));
#66479=CARTESIAN_POINT('Ctrl Pts',(41.3876324703314,-8.01705606706692,-7.31416422417865));
#66480=CARTESIAN_POINT('Ctrl Pts',(41.3184349028563,-8.02336677939693,-7.24569290345364));
#66481=CARTESIAN_POINT('Ctrl Pts',(41.2459908033385,-8.02967749172695,-7.18044490445988));
#66482=CARTESIAN_POINT('Ctrl Pts',(41.1706379289395,-8.03598820405697,-7.11873384557626));
#66483=CARTESIAN_POINT('Ctrl Pts',(41.0952918753744,-8.04229834515037,-7.05702837268908));
#66484=CARTESIAN_POINT('Ctrl Pts',(41.0170379088886,-8.04860848624376,-6.99885948028117));
#66485=CARTESIAN_POINT('Ctrl Pts',(40.9362470892756,-8.05491862733716,-6.94450068826169));
#66486=CARTESIAN_POINT('Ctrl Pts',(40.855441700766,-8.06122990632957,-6.89013209379651));
#66487=CARTESIAN_POINT('Ctrl Pts',(40.772098913387,-8.06754118532197,-6.83957520841959));
#66488=CARTESIAN_POINT('Ctrl Pts',(40.6866181055634,-8.07385246431438,-6.79305979913337));
#66489=CARTESIAN_POINT('Ctrl Pts',(40.601045881739,-8.08017049279711,-6.74649464473128));
#66490=CARTESIAN_POINT('Ctrl Pts',(40.5133314574149,-8.08648852127983,-6.70397980460187));
#66491=CARTESIAN_POINT('Ctrl Pts',(40.4238979283777,-8.09280654976256,-6.66569859689246));
#66492=CARTESIAN_POINT('Ctrl Pts',(40.3344119941812,-8.0991282804059,-6.62739495763183));
#66493=CARTESIAN_POINT('Ctrl Pts',(40.2432053588737,-8.10545001104925,-6.59333004362667));
#66494=CARTESIAN_POINT('Ctrl Pts',(40.1507181885533,-8.11177174169259,-6.56363788454469));
#66495=CARTESIAN_POINT('Ctrl Pts',(40.0580827217895,-8.11810360877071,-6.5338981162476));
#66496=CARTESIAN_POINT('Ctrl Pts',(39.9641630419777,-8.12443547584883,-6.50854521729546));
#66497=CARTESIAN_POINT('Ctrl Pts',(39.8694114161616,-8.13076734292696,-6.48766251318487));
#66498=CARTESIAN_POINT('Ctrl Pts',(39.8143781125389,-8.13444499553089,-6.47553349496609));
#66499=CARTESIAN_POINT('Ctrl Pts',(39.7590643061235,-8.13812264813482,-6.46491152181761));
#66500=CARTESIAN_POINT('Ctrl Pts',(39.7035592723059,-8.14180030073875,-6.45580487551301));
#66501=CARTESIAN_POINT('Ctrl Pts',(39.6079840961829,-8.14813292088444,-6.44012396759189));
#66502=CARTESIAN_POINT('Ctrl Pts',(39.5115097532658,-8.15446554103013,-6.42888441029796));
#66503=CARTESIAN_POINT('Ctrl Pts',(39.4145845959796,-8.16079816117581,-6.42218126470974));
#66504=CARTESIAN_POINT('Ctrl Pts',(39.3177898844641,-8.16712225862689,-6.41548714048415));
#66505=CARTESIAN_POINT('Ctrl Pts',(39.2205459970585,-8.17344635607797,-6.41331732334219));
#66506=CARTESIAN_POINT('Ctrl Pts',(39.1233101320149,-8.17977045352904,-6.41571562621744));
#66507=CARTESIAN_POINT('Ctrl Pts',(39.0261760438908,-8.18608793153824,-6.41811141878562));
#66508=CARTESIAN_POINT('Ctrl Pts',(38.9290503963186,-8.19240540954744,-6.42506581487646));
#66509=CARTESIAN_POINT('Ctrl Pts',(38.8323931374479,-8.19872288755664,-6.43657065039451));
#66510=CARTESIAN_POINT('Ctrl Pts',(38.7358044890827,-8.2050358812119,-6.44806731940143));
#66511=CARTESIAN_POINT('Ctrl Pts',(38.6396840014497,-8.21134887486717,-6.46410795475885));
#66512=CARTESIAN_POINT('Ctrl Pts',(38.5444882849865,-8.21766186852243,-6.48463241623977));
#66513=CARTESIAN_POINT('Ctrl Pts',(38.4493269693882,-8.22397258085192,-6.50514946079845));
#66514=CARTESIAN_POINT('Ctrl Pts',(38.3550901879882,-8.23028329318141,-6.53014701981337));
#66515=CARTESIAN_POINT('Ctrl Pts',(38.2622251834637,-8.23659400551089,-6.55951369142086));
#66516=CARTESIAN_POINT('Ctrl Pts',(38.169368584947,-8.24290414660371,-6.58887770479914));
#66517=CARTESIAN_POINT('Ctrl Pts',(38.0778839333214,-8.24921428769652,-6.62260991239922));
#66518=CARTESIAN_POINT('Ctrl Pts',(37.9882030973958,-8.25552442878933,-6.66054910676779));
#66519=CARTESIAN_POINT('Ctrl Pts',(37.8985060894496,-8.26183570778113,-6.6984951426586));
#66520=CARTESIAN_POINT('Ctrl Pts',(37.8106139459859,-8.26814698677292,-6.74064950165813));
#66521=CARTESIAN_POINT('Ctrl Pts',(37.724937377438,-8.27445826576472,-6.78680334664938));
#66522=CARTESIAN_POINT('Ctrl Pts',(37.639169183538,-8.28077629424672,-6.83300655008687));
#66523=CARTESIAN_POINT('Ctrl Pts',(37.5556216805866,-8.28709432272872,-6.88321757093409));
#66524=CARTESIAN_POINT('Ctrl Pts',(37.4746796479639,-8.29341235121072,-6.9371823217719));
#66525=CARTESIAN_POINT('Ctrl Pts',(37.3936901859248,-8.29973408185332,-6.99117869421039));
#66526=CARTESIAN_POINT('Ctrl Pts',(37.3153095862391,-8.30605581249591,-7.0489329172736));
#66527=CARTESIAN_POINT('Ctrl Pts',(37.2398906859807,-8.3123775431385,-7.11014966716469));
#66528=CARTESIAN_POINT('Ctrl Pts',(37.1643508570083,-8.31870941021578,-7.17146457365599));
#66529=CARTESIAN_POINT('Ctrl Pts',(37.0917825361352,-8.32504127729307,-7.23625280210336));
#66530=CARTESIAN_POINT('Ctrl Pts',(37.0225027163061,-8.33137314437035,-7.3041811797435));
#66531=CARTESIAN_POINT('Ctrl Pts',(36.9822638567299,-8.33505079697982,-7.34363509945403));
#66532=CARTESIAN_POINT('Ctrl Pts',(36.9431336406883,-8.33872844958928,-7.38414768634009));
#66533=CARTESIAN_POINT('Ctrl Pts',(36.9051678028014,-8.34240610219874,-7.42564870981517));
#66534=CARTESIAN_POINT('Ctrl Pts',(36.840538557626,-8.34866657017196,-7.49629590135606));
#66535=CARTESIAN_POINT('Ctrl Pts',(36.7790497127769,-8.35492703814518,-7.57006721002526));
#66536=CARTESIAN_POINT('Ctrl Pts',(36.7210228966364,-8.3611875061184,-7.64664881507776));
#66537=CARTESIAN_POINT('Ctrl Pts',(36.663067628609,-8.36744025482145,-7.72313599362693));
#66538=CARTESIAN_POINT('Ctrl Pts',(36.6085661827415,-8.3736930035245,-7.80242623624781));
#66539=CARTESIAN_POINT('Ctrl Pts',(36.5578026363479,-8.37994575222754,-7.8841698002506));
#66540=CARTESIAN_POINT('Ctrl Pts',(36.5070871640247,-8.38619257945537,-7.96583595150082));
#66541=CARTESIAN_POINT('Ctrl Pts',(36.4601027966921,-8.3924394066832,-8.04995043222001));
#66542=CARTESIAN_POINT('Ctrl Pts',(36.4170919295187,-8.39868623391103,-8.13613235902414));
#66543=CARTESIAN_POINT('Ctrl Pts',(36.3741094987145,-8.40492893108761,-8.22225730717951));
#66544=CARTESIAN_POINT('Ctrl Pts',(36.335095548604,-8.41117162826419,-8.3104465863091));
#66545=CARTESIAN_POINT('Ctrl Pts',(36.3002472873748,-8.41741432544077,-8.40029343448054));
#66546=CARTESIAN_POINT('Ctrl Pts',(36.2654023210465,-8.42365643237072,-8.49013178763803));
#66547=CARTESIAN_POINT('Ctrl Pts',(36.2347224379543,-8.42989853930067,-8.58162698684104));
#66548=CARTESIAN_POINT('Ctrl Pts',(36.2083569558186,-8.43614064623061,-8.67435168894478));
#66549=CARTESIAN_POINT('Ctrl Pts',(36.1819945151201,-8.44238203309121,-8.76706569462549));
#66550=CARTESIAN_POINT('Ctrl Pts',(36.1599456030518,-8.4486234199518,-8.86100848840364));
#66551=CARTESIAN_POINT('Ctrl Pts',(36.1423093694155,-8.45486480681239,-8.9557384954734));
#66552=CARTESIAN_POINT('Ctrl Pts',(36.1246594966111,-8.46111102051567,-9.05054176299818));
#66553=CARTESIAN_POINT('Ctrl Pts',(36.1114291994719,-8.46735723421894,-9.14613301810445));
#66554=CARTESIAN_POINT('Ctrl Pts',(36.102666203883,-8.47360344792221,-9.24206182949071));
#66555=CARTESIAN_POINT('Ctrl Pts',(36.0939836110761,-8.47979235097709,-9.33711046888127));
#66556=CARTESIAN_POINT('Ctrl Pts',(36.0896866409204,-8.48598125403197,-9.4324900624374));
#66557=CARTESIAN_POINT('Ctrl Pts',(36.0897712258115,-8.49217015708684,-9.52776136011945));
#66558=CARTESIAN_POINT('',(36.089632242379,-9.76217020937298,-9.52362827152999));
#66559=CARTESIAN_POINT('Ctrl Pts',(36.0897712258121,-8.4921701571312,-9.52776136080225));
#66560=CARTESIAN_POINT('Ctrl Pts',(36.0898810476013,-8.50020559029366,-9.65145794128347));
#66561=CARTESIAN_POINT('Ctrl Pts',(36.0973737509533,-8.50824102345612,-9.77483167154566));
#66562=CARTESIAN_POINT('Ctrl Pts',(36.112112747417,-8.51627645661858,-9.89713299804683));
#66563=CARTESIAN_POINT('Ctrl Pts',(36.1271629019818,-8.52448152752612,-10.0220162539634));
#66564=CARTESIAN_POINT('Ctrl Pts',(36.1497685385396,-8.53268659843367,-10.1457816117599));
#66565=CARTESIAN_POINT('Ctrl Pts',(36.1797360223109,-8.54089166934121,-10.2676548040467));
#66566=CARTESIAN_POINT('Ctrl Pts',(36.1823172751409,-8.54159841411371,-10.2781523661675));
#66567=CARTESIAN_POINT('Ctrl Pts',(36.1849531182365,-8.54230515888621,-10.2886359026316));
#66568=CARTESIAN_POINT('Ctrl Pts',(36.1876434113821,-8.54301190365871,-10.2991049256466));
#66569=CARTESIAN_POINT('Ctrl Pts',(36.2117491496296,-8.54934452377532,-10.3929101412286));
#66570=CARTESIAN_POINT('Ctrl Pts',(36.2402825925639,-8.55567714389193,-10.4857512369077));
#66571=CARTESIAN_POINT('Ctrl Pts',(36.2731503405401,-8.56200976400854,-10.5771795112145));
#66572=CARTESIAN_POINT('Ctrl Pts',(36.3059738537809,-8.56833386143066,-10.6684847376775));
#66573=CARTESIAN_POINT('Ctrl Pts',(36.3431199314519,-8.57465795885278,-10.7583805138988));
#66574=CARTESIAN_POINT('Ctrl Pts',(36.3844446987308,-8.58098205627489,-10.8464306634837));
#66575=CARTESIAN_POINT('Ctrl Pts',(36.4257262113175,-8.58729953425532,-10.9343886508527));
#66576=CARTESIAN_POINT('Ctrl Pts',(36.4711775332836,-8.59361701223574,-11.0205044583357));
#66577=CARTESIAN_POINT('Ctrl Pts',(36.5206061004642,-8.59993449021616,-11.1043603084889));
#66578=CARTESIAN_POINT('Ctrl Pts',(36.5699995816227,-8.60624748384301,-11.1881566350026));
#66579=CARTESIAN_POINT('Ctrl Pts',(36.6233644739105,-8.61256047746985,-11.2696958177493));
#66580=CARTESIAN_POINT('Ctrl Pts',(36.6804619743907,-8.61887347109669,-11.3485840508211));
#66581=CARTESIAN_POINT('Ctrl Pts',(36.7375388415559,-8.62518418339798,-11.427443776064));
#66582=CARTESIAN_POINT('Ctrl Pts',(36.7983453805853,-8.63149489569927,-11.5036541012356));
#66583=CARTESIAN_POINT('Ctrl Pts',(36.8625996304447,-8.63780560800057,-11.5768504246906));
#66584=CARTESIAN_POINT('Ctrl Pts',(36.9268480641038,-8.64411574906545,-11.6500401225219));
#66585=CARTESIAN_POINT('Ctrl Pts',(36.9945432994472,-8.65042589013034,-11.720216032561));
#66586=CARTESIAN_POINT('Ctrl Pts',(37.0653639672428,-8.65673603119522,-11.7870476698236));
#66587=CARTESIAN_POINT('Ctrl Pts',(37.1361974060345,-8.66304731015939,-11.8538913587459));
#66588=CARTESIAN_POINT('Ctrl Pts',(37.2101570785947,-8.66935858912356,-11.9173892770119));
#66589=CARTESIAN_POINT('Ctrl Pts',(37.2868865272362,-8.67566986808774,-11.9772494761402));
#66590=CARTESIAN_POINT('Ctrl Pts',(37.3636980328925,-8.68198789654275,-12.0371736917487));
#66591=CARTESIAN_POINT('Ctrl Pts',(37.4432848829153,-8.68830592499776,-12.093452152018));
#66592=CARTESIAN_POINT('Ctrl Pts',(37.5252596299661,-8.69462395345278,-12.145834856659));
#66593=CARTESIAN_POINT('Ctrl Pts',(37.6072824115746,-8.70094568406868,-12.1982482558754));
#66594=CARTESIAN_POINT('Ctrl Pts',(37.6916954974715,-8.70726741468458,-12.2467611360026));
#66595=CARTESIAN_POINT('Ctrl Pts',(37.7780865442638,-8.71358914530048,-12.2911693327228));
#66596=CARTESIAN_POINT('Ctrl Pts',(37.8646161128191,-8.71992101235185,-12.3356487347581));
#66597=CARTESIAN_POINT('Ctrl Pts',(37.9531295775849,-8.72625287940321,-12.3760101298394));
#66598=CARTESIAN_POINT('Ctrl Pts',(38.0431943702978,-8.73258474645458,-12.4120973984245));
#66599=CARTESIAN_POINT('Ctrl Pts',(38.0955054883842,-8.73626239934262,-12.4330574796227));
#66600=CARTESIAN_POINT('Ctrl Pts',(38.1483396355488,-8.73994005223066,-12.4525766208612));
#66601=CARTESIAN_POINT('Ctrl Pts',(38.2016100902036,-8.7436177051187,-12.4706320613608));
#66602=CARTESIAN_POINT('Ctrl Pts',(38.293337494604,-8.74995032525292,-12.5017220661874));
#66603=CARTESIAN_POINT('Ctrl Pts',(38.3866778299206,-8.75628294538714,-12.5285773868489));
#66604=CARTESIAN_POINT('Ctrl Pts',(38.4812043078318,-8.76261556552136,-12.5510309657735));
#66605=CARTESIAN_POINT('Ctrl Pts',(38.575603568206,-8.76893966296063,-12.5734543257683));
#66606=CARTESIAN_POINT('Ctrl Pts',(38.6711853764568,-8.7752637603999,-12.5914876181216));
#66607=CARTESIAN_POINT('Ctrl Pts',(38.7675058418423,-8.78158785783918,-12.6050128986839));
#66608=CARTESIAN_POINT('Ctrl Pts',(38.8637254884537,-8.78790533583628,-12.618524022315));
#66609=CARTESIAN_POINT('Ctrl Pts',(38.9606818243439,-8.79422281383338,-12.6275364543537));
#66610=CARTESIAN_POINT('Ctrl Pts',(39.057919751197,-8.80054029183049,-12.6319830794197));
#66611=CARTESIAN_POINT('Ctrl Pts',(39.1550886553608,-8.80685328547324,-12.6364265481244));
#66612=CARTESIAN_POINT('Ctrl Pts',(39.2525383174916,-8.81316627911599,-12.636310633159));
#66613=CARTESIAN_POINT('Ctrl Pts',(39.3498084376071,-8.81947927275875,-12.6316200419301));
#66614=CARTESIAN_POINT('Ctrl Pts',(39.4470434072268,-8.82578998507547,-12.6269311457397));
#66615=CARTESIAN_POINT('Ctrl Pts',(39.544098527388,-8.8321006973922,-12.6176708791558));
#66616=CARTESIAN_POINT('Ctrl Pts',(39.6405143621856,-8.83841140970892,-12.6038760529791));
#66617=CARTESIAN_POINT('Ctrl Pts',(39.736921469556,-8.84472155078874,-12.5900824754909));
#66618=CARTESIAN_POINT('Ctrl Pts',(39.832688973743,-8.85103169186857,-12.5717552166475));
#66619=CARTESIAN_POINT('Ctrl Pts',(39.9273644662361,-8.85734183294839,-12.5489827357571));
#66620=CARTESIAN_POINT('Ctrl Pts',(40.0220570314264,-8.863653111927,-12.5262061483376));
#66621=CARTESIAN_POINT('Ctrl Pts',(40.1156567686407,-8.86996439090561,-12.4989828490951));
#66622=CARTESIAN_POINT('Ctrl Pts',(40.2077243591099,-8.87627566988422,-12.4674517445417));
#66623=CARTESIAN_POINT('Ctrl Pts',(40.2998904096979,-8.88259369835279,-12.4358869195848));
#66624=CARTESIAN_POINT('Ctrl Pts',(40.3905206279047,-8.88891172682137,-12.4000052337996));
#66625=CARTESIAN_POINT('Ctrl Pts',(40.479193882072,-8.89522975528994,-12.3599944735342));
#66626=CARTESIAN_POINT('Ctrl Pts',(40.5679190958995,-8.90155148591894,-12.3199602682569));
#66627=CARTESIAN_POINT('Ctrl Pts',(40.6546846727078,-8.90787321654794,-12.2757923689068));
#66628=CARTESIAN_POINT('Ctrl Pts',(40.7390942543784,-8.91419494717694,-12.2277244641361));
#66629=CARTESIAN_POINT('Ctrl Pts',(40.8236391806651,-8.92052681424055,-12.1795794859811));
#66630=CARTESIAN_POINT('Ctrl Pts',(40.9058201992784,-8.92685868130416,-12.1275222493807));
#66631=CARTESIAN_POINT('Ctrl Pts',(40.9852701286095,-8.93319054836777,-12.0718296411018));
#66632=CARTESIAN_POINT('Ctrl Pts',(41.0314159568653,-8.93686820110474,-12.0394824564234));
#66633=CARTESIAN_POINT('Ctrl Pts',(41.0766410663143,-8.94054585384171,-12.00590965195));
#66634=CARTESIAN_POINT('Ctrl Pts',(41.1208789938497,-8.94422350657868,-11.971171405255));
#66635=CARTESIAN_POINT('Ctrl Pts',(41.197053124029,-8.95055612688772,-11.9113549564886));
#66636=CARTESIAN_POINT('Ctrl Pts',(41.270562866356,-8.95688874719677,-11.8478731106357));
#66637=CARTESIAN_POINT('Ctrl Pts',(41.3410350393383,-8.96322136750582,-11.7809919355409));
#66638=CARTESIAN_POINT('Ctrl Pts',(41.4114123680475,-8.9695454651208,-11.7142007718104));
#66639=CARTESIAN_POINT('Ctrl Pts',(41.4787599381421,-8.97586956273577,-11.6440196702687));
#66640=CARTESIAN_POINT('Ctrl Pts',(41.5427363462967,-8.98219366035075,-11.5707558663341));
#66641=CARTESIAN_POINT('Ctrl Pts',(41.6066457902582,-8.98851113852419,-11.4975687477223));
#66642=CARTESIAN_POINT('Ctrl Pts',(41.6671908011738,-8.99482861669763,-11.4213056691599));
#66643=CARTESIAN_POINT('Ctrl Pts',(41.7240664125183,-9.00114609487107,-11.3423110350451));
#66644=CARTESIAN_POINT('Ctrl Pts',(41.7809016516801,-9.00745908869036,-11.2633724739242));
#66645=CARTESIAN_POINT('Ctrl Pts',(41.8340724146941,-9.01377208250966,-11.1817065658849));
#66646=CARTESIAN_POINT('Ctrl Pts',(41.8833142871499,-9.02008507632895,-11.0976903984184));
#66647=CARTESIAN_POINT('Ctrl Pts',(41.9325383650749,-9.02639578882227,-11.0137045918662));
#66648=CARTESIAN_POINT('Ctrl Pts',(41.9778361526619,-9.0327065013156,-10.927370590385));
#66649=CARTESIAN_POINT('Ctrl Pts',(42.01898733824,-9.03901721380892,-10.8390932386032));
#66650=CARTESIAN_POINT('Ctrl Pts',(42.0601347988691,-9.04532735506519,-10.7508238775664));
#66651=CARTESIAN_POINT('Ctrl Pts',(42.0971362191833,-9.05163749632146,-10.6606119124268));
#66652=CARTESIAN_POINT('Ctrl Pts',(42.1298183783233,-9.05794763757773,-10.5688845352523));
#66653=CARTESIAN_POINT('Ctrl Pts',(42.1625064309886,-9.0642589167324,-10.477140617016));
#66654=CARTESIAN_POINT('Ctrl Pts',(42.1908735287742,-9.07057019588707,-10.3838811559448));
#66655=CARTESIAN_POINT('Ctrl Pts',(42.2147958494762,-9.07688147504175,-10.2895499583944));
#66656=CARTESIAN_POINT('Ctrl Pts',(42.2387437534904,-9.08319950368475,-10.1951178799764));
#66657=CARTESIAN_POINT('Ctrl Pts',(42.2582372828619,-9.08951753232775,-10.0996122014463));
#66658=CARTESIAN_POINT('Ctrl Pts',(42.2732034878762,-9.09583556097075,-10.0034882182518));
#66659=CARTESIAN_POINT('Ctrl Pts',(42.2881784626009,-9.10215729177351,-9.90730790952249));
#66660=CARTESIAN_POINT('Ctrl Pts',(42.2986207835065,-9.10847902257626,-9.81050900927613));
#66661=CARTESIAN_POINT('Ctrl Pts',(42.3045094803033,-9.11480075337901,-9.71355115912394));
#66662=CARTESIAN_POINT('Ctrl Pts',(42.3104076191937,-9.1211326206136,-9.61643784416791));
#66663=CARTESIAN_POINT('Ctrl Pts',(42.3117375483811,-9.12746448784819,-9.51916550738235));
#66664=CARTESIAN_POINT('Ctrl Pts',(42.3085304193097,-9.13379635508278,-9.42219297141593));
#66665=CARTESIAN_POINT('Ctrl Pts',(42.3066676668305,-9.13747400606808,-9.36586975280906));
#66666=CARTESIAN_POINT('Ctrl Pts',(42.3032753221632,-9.14115165705338,-9.30964758006777));
#66667=CARTESIAN_POINT('Ctrl Pts',(42.2983674468807,-9.14482930803867,-9.25361500223825));
#66668=CARTESIAN_POINT('Ctrl Pts',(42.2899164794979,-9.15116192790624,-9.15713139979396));
#66669=CARTESIAN_POINT('Ctrl Pts',(42.2769397722392,-9.1574945477738,-9.06087533093716));
#66670=CARTESIAN_POINT('Ctrl Pts',(42.2594561373029,-9.16382716764137,-8.96530472860719));
#66671=CARTESIAN_POINT('Ctrl Pts',(42.2419960325448,-9.17015126481474,-8.86986274903271));
#66672=CARTESIAN_POINT('Ctrl Pts',(42.2200411338116,-9.17647536198812,-8.77510482895813));
#66673=CARTESIAN_POINT('Ctrl Pts',(42.1936620968134,-9.1827994591615,-8.68148479385209));
#66674=CARTESIAN_POINT('Ctrl Pts',(42.1673106707889,-9.18911693689381,-8.58796275096358));
#66675=CARTESIAN_POINT('Ctrl Pts',(42.1365444306355,-9.19543441462612,-8.49557664393902));
#66676=CARTESIAN_POINT('Ctrl Pts',(42.1014850737235,-9.20175189235842,-8.40477010401458));
#66677=CARTESIAN_POINT('Ctrl Pts',(42.0664506030861,-9.20806488573908,-8.31402802153248));
#66678=CARTESIAN_POINT('Ctrl Pts',(42.027129231155,-9.21437787911974,-8.22486368388727));
#66679=CARTESIAN_POINT('Ctrl Pts',(41.9836921900713,-9.2206908725004,-8.13770462992338));
#66680=CARTESIAN_POINT('Ctrl Pts',(41.9402708458164,-9.2270015845568,-8.05057707259705));
#66681=CARTESIAN_POINT('Ctrl Pts',(41.8927369825086,-9.23331229661319,-7.96545375007072));
#66682=CARTESIAN_POINT('Ctrl Pts',(41.8413091829943,-9.23962300866959,-7.88274044294757));
#66683=CARTESIAN_POINT('Ctrl Pts',(41.7898860386361,-9.24593314949116,-7.80003462289102));
#66684=CARTESIAN_POINT('Ctrl Pts',(41.7345698899532,-9.25224329031274,-7.71973875577314));
#66685=CARTESIAN_POINT('Ctrl Pts',(41.6756237738523,-9.25855343113431,-7.64223140475594));
#66686=CARTESIAN_POINT('Ctrl Pts',(41.6166670280592,-9.26486470985705,-7.56471007691832));
#66687=CARTESIAN_POINT('Ctrl Pts',(41.554079279504,-9.27117598857979,-7.4899786119637));
#66688=CARTESIAN_POINT('Ctrl Pts',(41.488164479829,-9.27748726730253,-7.41838328921731));
#66689=CARTESIAN_POINT('Ctrl Pts',(41.4221791886356,-9.2838052955204,-7.34671140000888));
#66690=CARTESIAN_POINT('Ctrl Pts',(41.3528600395366,-9.29012332373827,-7.27818267113638));
#66691=CARTESIAN_POINT('Ctrl Pts',(41.2805484127911,-9.29644135195615,-7.21310706239831));
#66692=CARTESIAN_POINT('Ctrl Pts',(41.2081944137392,-9.302763082337,-7.14799332142959));
#66693=CARTESIAN_POINT('Ctrl Pts',(41.1328447836484,-9.30908481271785,-7.08633700659209));
#66694=CARTESIAN_POINT('Ctrl Pts',(41.0548729551091,-9.3154065430987,-7.02840692676906));
#66695=CARTESIAN_POINT('Ctrl Pts',(40.9767761043376,-9.3217384099206,-6.97038396021979));
#66696=CARTESIAN_POINT('Ctrl Pts',(40.8960490221214,-9.3280702767425,-6.91609940308681));
#66697=CARTESIAN_POINT('Ctrl Pts',(40.81309294599,-9.3344021435644,-6.86577797081605));
#66698=CARTESIAN_POINT('Ctrl Pts',(40.7649106543247,-9.33807979887582,-6.83655043210212));
#66699=CARTESIAN_POINT('Ctrl Pts',(40.7159768708064,-9.34175745418723,-6.80865898229115));
#66700=CARTESIAN_POINT('Ctrl Pts',(40.6663734313878,-9.34543510949864,-6.78214024918883));
#66701=CARTESIAN_POINT('Ctrl Pts',(40.5809603861182,-9.35176772964116,-6.73647717062995));
#66702=CARTESIAN_POINT('Ctrl Pts',(40.4932640181722,-9.35810034978367,-6.69472823736366));
#66703=CARTESIAN_POINT('Ctrl Pts',(40.4036780752508,-9.36443296992618,-6.65712801121451));
#66704=CARTESIAN_POINT('Ctrl Pts',(40.3142127007285,-9.37075706737141,-6.61957838897624));
#66705=CARTESIAN_POINT('Ctrl Pts',(40.2228632055255,-9.37708116481664,-6.58616654420512));
#66706=CARTESIAN_POINT('Ctrl Pts',(40.130048236466,-9.38340526226186,-6.55708138070693));
#66707=CARTESIAN_POINT('Ctrl Pts',(40.0373304170062,-9.3897227402626,-6.52802666070316));
#66708=CARTESIAN_POINT('Ctrl Pts',(39.9431505882964,-9.39604021826333,-6.50328974869088));
#66709=CARTESIAN_POINT('Ctrl Pts',(39.8479467610354,-9.40235769626406,-6.48301123477358));
#66710=CARTESIAN_POINT('Ctrl Pts',(39.7528105126443,-9.40867068990701,-6.46274711522564));
#66711=CARTESIAN_POINT('Ctrl Pts',(39.6566521372651,-9.41498368354997,-6.44693519296503));
#66712=CARTESIAN_POINT('Ctrl Pts',(39.5599232467678,-9.42129667719292,-6.43566578218929));
#66713=CARTESIAN_POINT('Ctrl Pts',(39.4632293112145,-9.42760738950773,-6.42440044384343));
#66714=CARTESIAN_POINT('Ctrl Pts',(39.365965704134,-9.43391810182253,-6.41767440580317));
#66715=CARTESIAN_POINT('Ctrl Pts',(39.268591700239,-9.44022881413734,-6.41552643819596));
#66716=CARTESIAN_POINT('Ctrl Pts',(39.1712265105358,-9.44653895521315,-6.4133786650205));
#66717=CARTESIAN_POINT('Ctrl Pts',(39.0737513810958,-9.45284909628896,-6.41580814778705));
#66718=CARTESIAN_POINT('Ctrl Pts',(38.9766270946817,-9.45915923736477,-6.42280155404758));
#66719=CARTESIAN_POINT('Ctrl Pts',(38.879485294015,-9.46547051633727,-6.4297962214168));
#66720=CARTESIAN_POINT('Ctrl Pts',(38.7826948982055,-9.47178179530978,-6.44135641542825));
#66721=CARTESIAN_POINT('Ctrl Pts',(38.6867120208982,-9.47809307428228,-6.4574168954355));
#66722=CARTESIAN_POINT('Ctrl Pts',(38.5906264963822,-9.48441110274165,-6.47349455104208));
#66723=CARTESIAN_POINT('Ctrl Pts',(38.4953506464988,-9.49072913120102,-6.49408202875086));
#66724=CARTESIAN_POINT('Ctrl Pts',(38.4013306307846,-9.49704715966039,-6.51906289294385));
#66725=CARTESIAN_POINT('Ctrl Pts',(38.307255522407,-9.50336889027841,-6.54405839510869));
#66726=CARTESIAN_POINT('Ctrl Pts',(38.2144381302551,-9.50969062089644,-6.5734522780838));
#66727=CARTESIAN_POINT('Ctrl Pts',(38.1233076752637,-9.51601235151446,-6.60707877235282));
#66728=CARTESIAN_POINT('Ctrl Pts',(38.0320310992633,-9.52234421856445,-6.64075918424217));
#66729=CARTESIAN_POINT('Ctrl Pts',(37.9424472640501,-9.52867608561444,-6.67868558885452));
#66730=CARTESIAN_POINT('Ctrl Pts',(37.8549636662382,-9.53500795266442,-6.72064483102433));
#66731=CARTESIAN_POINT('Ctrl Pts',(37.8041517504443,-9.53868560542916,-6.74501545058311));
#66732=CARTESIAN_POINT('Ctrl Pts',(37.7540478701526,-9.54236325819389,-6.77074568509546));
#66733=CARTESIAN_POINT('Ctrl Pts',(37.7047274297335,-9.54604091095863,-6.79778702820835));
#66734=CARTESIAN_POINT('Ctrl Pts',(37.6198016118814,-9.55237353220384,-6.84435003859853));
#66735=CARTESIAN_POINT('Ctrl Pts',(37.5369053206938,-9.55870615344906,-6.89496460821624));
#66736=CARTESIAN_POINT('Ctrl Pts',(37.456450203917,-9.56503877469427,-6.94942923578501));
#66737=CARTESIAN_POINT('Ctrl Pts',(37.3761033667938,-9.57136287324929,-7.00382056272055));
#66738=CARTESIAN_POINT('Ctrl Pts',(37.2981915332185,-9.57768697180431,-7.06205140593578));
#66739=CARTESIAN_POINT('Ctrl Pts',(37.2231017280754,-9.58401107035933,-7.12387445655967));
#66740=CARTESIAN_POINT('Ctrl Pts',(37.1480905194909,-9.59032854947539,-7.18563279694752));
#66741=CARTESIAN_POINT('Ctrl Pts',(37.0758958028394,-9.59664602859145,-7.25097559324891));
#66742=CARTESIAN_POINT('Ctrl Pts',(37.0068747306551,-9.6029635077075,-7.31961291246618));
#66743=CARTESIAN_POINT('Ctrl Pts',(36.9379026518954,-9.60927650246933,-7.38820151065927));
#66744=CARTESIAN_POINT('Ctrl Pts',(36.8721000481953,-9.61558949723116,-7.46007967508075));
#66745=CARTESIAN_POINT('Ctrl Pts',(36.809789406625,-9.62190249199298,-7.53491860161005));
#66746=CARTESIAN_POINT('Ctrl Pts',(36.7475012822458,-9.62821320542843,-7.60973048360285));
#66747=CARTESIAN_POINT('Ctrl Pts',(36.6887028921384,-9.63452391886388,-7.68750066600639));
#66748=CARTESIAN_POINT('Ctrl Pts',(36.6336777499718,-9.64083463229933,-7.76786575301988));
#66749=CARTESIAN_POINT('Ctrl Pts',(36.5786575886188,-9.64714477449615,-7.84822356547685));
#66750=CARTESIAN_POINT('Ctrl Pts',(36.5274102430144,-9.65345491669297,-7.93117545457953));
#66751=CARTESIAN_POINT('Ctrl Pts',(36.4801764214208,-9.6597650588898,-8.01632828146589));
#66752=CARTESIAN_POINT('Ctrl Pts',(36.4329340822439,-9.66607633898231,-8.10149646379606));
#66753=CARTESIAN_POINT('Ctrl Pts',(36.3897069166311,-9.67238761907482,-8.18886598975324));
#66754=CARTESIAN_POINT('Ctrl Pts',(36.3506896136501,-9.67869889916732,-8.27801925630812));
#66755=CARTESIAN_POINT('Ctrl Pts',(36.3116305843562,-9.68501692873832,-8.36726786612877));
#66756=CARTESIAN_POINT('Ctrl Pts',(36.2767905816254,-9.69133495830932,-8.45830362365475));
#66757=CARTESIAN_POINT('Ctrl Pts',(36.2463159836989,-9.69765298788032,-8.55068927710535));
#66758=CARTESIAN_POINT('Ctrl Pts',(36.21582352867,-9.70397471960686,-8.64312906548131));
#66759=CARTESIAN_POINT('Ctrl Pts',(36.1897016893659,-9.71029645133341,-8.73691990377445));
#66760=CARTESIAN_POINT('Ctrl Pts',(36.1680462737751,-9.71661818305996,-8.83161175743245));
#66761=CARTESIAN_POINT('Ctrl Pts',(36.1463561353721,-9.72295005120263,-8.92645544227755));
#66762=CARTESIAN_POINT('Ctrl Pts',(36.1291467983957,-9.7292819193453,-9.02220259717521));
#66763=CARTESIAN_POINT('Ctrl Pts',(36.1164625160446,-9.73561378748798,-9.11839547722381));
#66764=CARTESIAN_POINT('Ctrl Pts',(36.109095299302,-9.73929142913152,-9.17426570912192));
#66765=CARTESIAN_POINT('Ctrl Pts',(36.103253615341,-9.74296907077507,-9.23028623541386));
#66766=CARTESIAN_POINT('Ctrl Pts',(36.0989380633046,-9.74664671241861,-9.28636740021731));
#66767=CARTESIAN_POINT('Ctrl Pts',(36.0928660349285,-9.75182119397469,-9.36527420545974));
#66768=CARTESIAN_POINT('Ctrl Pts',(36.089805257095,-9.75699567553077,-9.4444156691509));
#66769=CARTESIAN_POINT('Ctrl Pts',(36.0897703028187,-9.76217015708685,-9.52362753095574));
#66770=CARTESIAN_POINT('',(36.0899227214263,-11.0321701121905,-9.5235494817152));
#66771=CARTESIAN_POINT('Ctrl Pts',(36.0855288150644,-9.76217176341955,-9.52365028285052));
#66772=CARTESIAN_POINT('Ctrl Pts',(36.0907961189434,-9.8238653469059,-10.4693569116554));
#66773=CARTESIAN_POINT('Ctrl Pts',(37.0531323133709,-9.95242753087891,-12.44936419088));
#66774=CARTESIAN_POINT('Ctrl Pts',(40.4146891398233,-10.1478583153386,-12.9880019777843));
#66775=CARTESIAN_POINT('Ctrl Pts',(42.7638264718393,-10.3484641167986,-10.4007848696135));
#66776=CARTESIAN_POINT('Ctrl Pts',(41.8814197118133,-10.5490699182586,-7.01943676244128));
#66777=CARTESIAN_POINT('Ctrl Pts',(38.5676048507788,-10.7496757197186,-5.9100433496554));
#66778=CARTESIAN_POINT('Ctrl Pts',(36.3678047754139,-10.9107087127355,-7.65077367760187));
#66779=CARTESIAN_POINT('Ctrl Pts',(36.092255627385,-11.0048731052659,-9.10216184953282));
#66780=CARTESIAN_POINT('Ctrl Pts',(36.0940461619714,-11.0321688973096,-9.5235326496095));
#66781=CARTESIAN_POINT('',(36.0897713719083,-12.3021701571198,-9.52792128380894));
#66782=CARTESIAN_POINT('Ctrl Pts',(36.0897703379492,-11.0321701570869,-9.52355010375274));
#66783=CARTESIAN_POINT('Ctrl Pts',(36.0897241617295,-11.0385779524537,-9.62260453497503));
#66784=CARTESIAN_POINT('Ctrl Pts',(36.0944143525894,-11.0449857478205,-9.72164861444106));
#66785=CARTESIAN_POINT('Ctrl Pts',(36.1038115441062,-11.0513935431873,-9.82020789029057));
#66786=CARTESIAN_POINT('Ctrl Pts',(36.1132122425988,-11.0578037299051,-9.91880394787363));
#66787=CARTESIAN_POINT('Ctrl Pts',(36.1273233973644,-11.0642139166229,-10.0169144255494));
#66788=CARTESIAN_POINT('Ctrl Pts',(36.1460638966692,-11.0706241033407,-10.1140712432912));
#66789=CARTESIAN_POINT('Ctrl Pts',(36.1656183557366,-11.0773127049489,-10.2154478920533));
#66790=CARTESIAN_POINT('Ctrl Pts',(36.1902132986866,-11.084001306557,-10.3157856690931));
#66791=CARTESIAN_POINT('Ctrl Pts',(36.2196981073553,-11.0906899081652,-10.4145680308993));
#66792=CARTESIAN_POINT('Ctrl Pts',(36.2480163797545,-11.0971138820983,-10.5094421696908));
#66793=CARTESIAN_POINT('Ctrl Pts',(36.2808447273581,-11.1035378560314,-10.6028812604354));
#66794=CARTESIAN_POINT('Ctrl Pts',(36.3180000700141,-11.1099618299644,-10.6944473294942));
#66795=CARTESIAN_POINT('Ctrl Pts',(36.3551891151171,-11.116391630883,-10.7860964552649));
#66796=CARTESIAN_POINT('Ctrl Pts',(36.3967127984438,-11.1228214318015,-10.8758687966678));
#66797=CARTESIAN_POINT('Ctrl Pts',(36.442341679746,-11.12925123272,-10.9633501804617));
#66798=CARTESIAN_POINT('Ctrl Pts',(36.4880483250545,-11.1356919917656,-11.050980656293));
#66799=CARTESIAN_POINT('Ctrl Pts',(36.5378739228314,-11.1421327508112,-11.1363120218029));
#66800=CARTESIAN_POINT('Ctrl Pts',(36.5915453137922,-11.1485735098568,-11.2189583238382));
#66801=CARTESIAN_POINT('Ctrl Pts',(36.5979723797916,-11.1493447807841,-11.2288550905937));
#66802=CARTESIAN_POINT('Ctrl Pts',(36.6044545459733,-11.1501160517113,-11.2387133935015));
#66803=CARTESIAN_POINT('Ctrl Pts',(36.6109913052643,-11.1508873226385,-11.2485326023847));
#66804=CARTESIAN_POINT('Ctrl Pts',(36.6646633149648,-11.1572200723766,-11.3291561424247));
#66805=CARTESIAN_POINT('Ctrl Pts',(36.7221981354031,-11.1635528221147,-11.407410242574));
#66806=CARTESIAN_POINT('Ctrl Pts',(36.7833597112063,-11.1698855718528,-11.4829020321454));
#66807=CARTESIAN_POINT('Ctrl Pts',(36.8444389669447,-11.1762097980635,-11.5582922139847));
#66808=CARTESIAN_POINT('Ctrl Pts',(36.9091350030548,-11.1825340242742,-11.6309271378762));
#66809=CARTESIAN_POINT('Ctrl Pts',(36.9771682360055,-11.1888582504848,-11.7004423922221));
#66810=CARTESIAN_POINT('Ctrl Pts',(37.0451302492573,-11.1951758562621,-11.7698848754344));
#66811=CARTESIAN_POINT('Ctrl Pts',(37.1164222098382,-11.2014934620394,-11.8362138707592));
#66812=CARTESIAN_POINT('Ctrl Pts',(37.1907246276679,-11.2078110678167,-11.8990983827634));
#66813=CARTESIAN_POINT('Ctrl Pts',(37.2649742809055,-11.2141241872542,-11.9619382384061));
#66814=CARTESIAN_POINT('Ctrl Pts',(37.3422298084112,-11.2204373066918,-12.0213381919138));
#66815=CARTESIAN_POINT('Ctrl Pts',(37.4221359635795,-11.2267504261293,-12.0770051177265));
#66816=CARTESIAN_POINT('Ctrl Pts',(37.5020132275409,-11.2330612629687,-12.1326519163706));
#66817=CARTESIAN_POINT('Ctrl Pts',(37.5845388564222,-11.2393720998081,-12.1845681195381));
#66818=CARTESIAN_POINT('Ctrl Pts',(37.669326479712,-11.2456829366476,-12.2325023965251));
#66819=CARTESIAN_POINT('Ctrl Pts',(37.7541064092692,-11.2519932008339,-12.2804323238971));
#66820=CARTESIAN_POINT('Ctrl Pts',(37.8411475443659,-11.2583034650203,-12.3243808284582));
#66821=CARTESIAN_POINT('Ctrl Pts',(37.9300375495852,-11.2646137292066,-12.364141776565));
#66822=CARTESIAN_POINT('Ctrl Pts',(38.018943561905,-11.2709251297303,-12.4039098847286));
#66823=CARTESIAN_POINT('Ctrl Pts',(38.1096987064192,-11.277236530254,-12.4394887602099));
#66824=CARTESIAN_POINT('Ctrl Pts',(38.2018702174821,-11.2835479307777,-12.4707202158642));
#66825=CARTESIAN_POINT('Ctrl Pts',(38.294140252596,-11.2898660776891,-12.5019850554729));
#66826=CARTESIAN_POINT('Ctrl Pts',(38.3878292619987,-11.2961842246005,-12.528893057107));
#66827=CARTESIAN_POINT('Ctrl Pts',(38.4824890439523,-11.3025023715119,-12.5513358506371));
#66828=CARTESIAN_POINT('Ctrl Pts',(38.5772042688076,-11.3088242190065,-12.5737917890697));
#66829=CARTESIAN_POINT('Ctrl Pts',(38.6728909688513,-11.3151460665011,-12.5917772308581));
#66830=CARTESIAN_POINT('Ctrl Pts',(38.7690925400138,-11.3214679139956,-12.6052352854657));
#66831=CARTESIAN_POINT('Ctrl Pts',(38.8654483054211,-11.3277998943029,-12.6187149109744));
#66832=CARTESIAN_POINT('Ctrl Pts',(38.9623201546527,-11.3341318746102,-12.6276526189722));
#66833=CARTESIAN_POINT('Ctrl Pts',(39.0592482195775,-11.3404638549174,-12.6320435447879));
#66834=CARTESIAN_POINT('Ctrl Pts',(39.11552580665,-11.3441402779778,-12.6345929685292));
#66835=CARTESIAN_POINT('Ctrl Pts',(39.1718223593645,-11.3478167010381,-12.6356106023868));
#66836=CARTESIAN_POINT('Ctrl Pts',(39.2280485906473,-11.3514931240985,-12.6351035239141));
#66837=CARTESIAN_POINT('Ctrl Pts',(39.3249020817444,-11.357826011792,-12.6342300469048));
#66838=CARTESIAN_POINT('Ctrl Pts',(39.4218828453814,-11.3641588994855,-12.6288264923168));
#66839=CARTESIAN_POINT('Ctrl Pts',(39.5185328446035,-11.370491787179,-12.6188758022598));
#66840=CARTESIAN_POINT('Ctrl Pts',(39.615052809339,-11.376816154502,-12.6089385000236));
#66841=CARTESIAN_POINT('Ctrl Pts',(39.7112424628503,-11.3831405218251,-12.5944662661471));
#66842=CARTESIAN_POINT('Ctrl Pts',(39.8066438092959,-11.3894648891481,-12.5754940487637));
#66843=CARTESIAN_POINT('Ctrl Pts',(39.9019453324034,-11.3957826389602,-12.5565416829878));
#66844=CARTESIAN_POINT('Ctrl Pts',(39.9964597616624,-11.4021003887722,-12.5330987794212));
#66845=CARTESIAN_POINT('Ctrl Pts',(40.0897352726025,-11.4084181385842,-12.5052519688085));
#66846=CARTESIAN_POINT('Ctrl Pts',(40.1829446018916,-11.4147314057715,-12.4774249163069));
#66847=CARTESIAN_POINT('Ctrl Pts',(40.2749163426568,-11.4210446729589,-12.4452002935937));
#66848=CARTESIAN_POINT('Ctrl Pts',(40.3652108391374,-11.4273579401462,-12.4087153731353));
#66849=CARTESIAN_POINT('Ctrl Pts',(40.4554727210744,-11.4336689269694,-12.3722436310994));
#66850=CARTESIAN_POINT('Ctrl Pts',(40.5440581574955,-11.4399799137926,-12.3315148126457));
#66851=CARTESIAN_POINT('Ctrl Pts',(40.6305454802007,-11.4462909006158,-12.2867150979016));
#66852=CARTESIAN_POINT('Ctrl Pts',(40.7170249830089,-11.4526013168205,-12.2419194337991));
#66853=CARTESIAN_POINT('Ctrl Pts',(40.8014063611047,-11.4589117330252,-12.1930538065363));
#66854=CARTESIAN_POINT('Ctrl Pts',(40.8832916023835,-11.4652221492299,-12.1403508434329));
#66855=CARTESIAN_POINT('Ctrl Pts',(40.9651916128401,-11.4715337036087,-12.0876383745942));
#66856=CARTESIAN_POINT('Ctrl Pts',(41.0445942246253,-11.4778452579875,-12.0310874319583));
#66857=CARTESIAN_POINT('Ctrl Pts',(41.1211304090095,-11.4841568123663,-11.9709739582585));
#66858=CARTESIAN_POINT('Ctrl Pts',(41.1977484247345,-11.4904751149644,-11.910796212134));
#66859=CARTESIAN_POINT('Ctrl Pts',(41.2714935500206,-11.4967934175625,-11.8470486010112));
#66860=CARTESIAN_POINT('Ctrl Pts',(41.342030035329,-11.5031117201606,-11.7800472235961));
#66861=CARTESIAN_POINT('Ctrl Pts',(41.4126078473937,-11.5094337246011,-11.7130065906158));
#66862=CARTESIAN_POINT('Ctrl Pts',(41.4799729736348,-11.5157557290416,-11.6427087108299));
#66863=CARTESIAN_POINT('Ctrl Pts',(41.5438281804137,-11.5220777334821,-11.5695048578076));
#66864=CARTESIAN_POINT('Ctrl Pts',(41.6077857375214,-11.5284098711484,-11.4961836699772));
#66865=CARTESIAN_POINT('Ctrl Pts',(41.6682218698025,-11.5347420088148,-11.4199475504585));
#66866=CARTESIAN_POINT('Ctrl Pts',(41.7248811254073,-11.5410741464812,-11.3411789436787));
#66867=CARTESIAN_POINT('Ctrl Pts',(41.7577639531156,-11.5447490728403,-11.2954647086802));
#66868=CARTESIAN_POINT('Ctrl Pts',(41.7893754825444,-11.5484239991994,-11.2488980050405));
#66869=CARTESIAN_POINT('Ctrl Pts',(41.8196728876223,-11.5520989255585,-11.2015573699568));
#66870=CARTESIAN_POINT('Ctrl Pts',(41.8718724618999,-11.5584304774175,-11.1199939162207));
#66871=CARTESIAN_POINT('Ctrl Pts',(41.9203500411026,-11.5647620292766,-11.035848339955));
#66872=CARTESIAN_POINT('Ctrl Pts',(41.9648409709928,-11.5710935811357,-10.9494946675996));
#66873=CARTESIAN_POINT('Ctrl Pts',(42.0092720006465,-11.577416608528,-10.8632572572645));
#66874=CARTESIAN_POINT('Ctrl Pts',(42.0497268502101,-11.5837396359203,-10.7748180450956));
#66875=CARTESIAN_POINT('Ctrl Pts',(42.0859844286908,-11.5900626633125,-10.6845794626735));
#66876=CARTESIAN_POINT('Ctrl Pts',(42.1222040480089,-11.596379070935,-10.5944353537702));
#66877=CARTESIAN_POINT('Ctrl Pts',(42.1542349699074,-11.6026954785574,-10.5024960234953));
#66878=CARTESIAN_POINT('Ctrl Pts',(42.1819027494922,-11.6090118861799,-10.4091869968908));
#66879=CARTESIAN_POINT('Ctrl Pts',(42.2095509033465,-11.6153238133519,-10.3159441576651));
#66880=CARTESIAN_POINT('Ctrl Pts',(42.2328419437029,-11.621635740524,-10.2213339718679));
#66881=CARTESIAN_POINT('Ctrl Pts',(42.2516504805008,-11.627947667696,-10.125799465512));
#66882=CARTESIAN_POINT('Ctrl Pts',(42.2704522276816,-11.6342573163513,-10.0302994457677));
#66883=CARTESIAN_POINT('Ctrl Pts',(42.2847746020702,-11.6405669650065,-9.93387619725917));
#66884=CARTESIAN_POINT('Ctrl Pts',(42.2945429989377,-11.6468766136617,-9.83698442369069));
#66885=CARTESIAN_POINT('Ctrl Pts',(42.3043105177682,-11.6531856951712,-9.74010135928578));
#66886=CARTESIAN_POINT('Ctrl Pts',(42.3095248292482,-11.6594947766806,-9.64275028884194));
#66887=CARTESIAN_POINT('Ctrl Pts',(42.3101631532206,-11.66580385819,-9.54539149943055));
#66888=CARTESIAN_POINT('Ctrl Pts',(42.3108015928644,-11.672114082975,-9.44801506752728));
#66889=CARTESIAN_POINT('Ctrl Pts',(42.3068623952391,-11.6784243077599,-9.35063135134026));
#66890=CARTESIAN_POINT('Ctrl Pts',(42.2983748946307,-11.6847345325449,-9.25370004566518));
#66891=CARTESIAN_POINT('Ctrl Pts',(42.289878296095,-11.6910515213902,-9.15666483731997));
#66892=CARTESIAN_POINT('Ctrl Pts',(42.2768236993154,-11.6973685102355,-9.06008344418471));
#66893=CARTESIAN_POINT('Ctrl Pts',(42.2592922556029,-11.7036854990808,-8.96440964358261));
#66894=CARTESIAN_POINT('Ctrl Pts',(42.2417505187476,-11.710006196786,-8.86867967053394));
#66895=CARTESIAN_POINT('Ctrl Pts',(42.2197267999755,-11.7163268944912,-8.77385877703149));
#66896=CARTESIAN_POINT('Ctrl Pts',(42.1933527578327,-11.7226475921964,-8.68038771020335));
#66897=CARTESIAN_POINT('Ctrl Pts',(42.1669363335332,-11.7289784470401,-8.58676643866337));
#66898=CARTESIAN_POINT('Ctrl Pts',(42.1361557648325,-11.7353093018838,-8.49449973986808));
#66899=CARTESIAN_POINT('Ctrl Pts',(42.1011916494707,-11.7416401567276,-8.40401040774618));
#66900=CARTESIAN_POINT('Ctrl Pts',(42.0808224722886,-11.7453283468245,-8.35129369462442));
#66901=CARTESIAN_POINT('Ctrl Pts',(42.0590343231343,-11.7490165369215,-8.29917979824462));
#66902=CARTESIAN_POINT('Ctrl Pts',(42.0358700493032,-11.7527047270185,-8.2477483739039));
#66903=CARTESIAN_POINT('Ctrl Pts',(41.9960890758525,-11.7590386096775,-8.15942304408162));
#66904=CARTESIAN_POINT('Ctrl Pts',(41.9521087431886,-11.7653724923366,-8.07280481370756));
#66905=CARTESIAN_POINT('Ctrl Pts',(41.9040978289802,-11.7717063749956,-7.9883199473526));
#66906=CARTESIAN_POINT('Ctrl Pts',(41.8561515555157,-11.7780317298669,-7.90394882939622));
#66907=CARTESIAN_POINT('Ctrl Pts',(41.804185700536,-11.7843570847382,-7.82170574339922));
#66908=CARTESIAN_POINT('Ctrl Pts',(41.7484166328061,-11.7906824396095,-7.74199598471091));
#66909=CARTESIAN_POINT('Ctrl Pts',(41.6927059860422,-11.7970011683463,-7.66236972609333));
#66910=CARTESIAN_POINT('Ctrl Pts',(41.6332002963815,-11.8033198970831,-7.58527187516194));
#66911=CARTESIAN_POINT('Ctrl Pts',(41.5701607612321,-11.8096386258199,-7.51108127800159));
#66912=CARTESIAN_POINT('Ctrl Pts',(41.5071661144676,-11.8159528551973,-7.43694350953161));
#66913=CARTESIAN_POINT('Ctrl Pts',(41.440642907176,-11.8222670845747,-7.36570921132328));
#66914=CARTESIAN_POINT('Ctrl Pts',(41.3708937990263,-11.8285813139521,-7.29772570924704));
#66915=CARTESIAN_POINT('Ctrl Pts',(41.3011699986349,-11.8348932522752,-7.22976687429672));
#66916=CARTESIAN_POINT('Ctrl Pts',(41.2282229358957,-11.8412051905983,-7.16505679652928));
#66917=CARTESIAN_POINT('Ctrl Pts',(41.1523928059093,-11.8475171289215,-7.10390665517963));
#66918=CARTESIAN_POINT('Ctrl Pts',(41.0765696728215,-11.8538284848377,-7.04276215619577));
#66919=CARTESIAN_POINT('Ctrl Pts',(40.9978643418071,-11.8601398407539,-6.98517721476751));
#66920=CARTESIAN_POINT('Ctrl Pts',(40.9166500115214,-11.8664511966701,-6.93142266534353));
#66921=CARTESIAN_POINT('Ctrl Pts',(40.835421201202,-11.8727636778637,-6.87765853180205));
#66922=CARTESIAN_POINT('Ctrl Pts',(40.7516828676701,-11.8790761590573,-6.82772638789288));
#66923=CARTESIAN_POINT('Ctrl Pts',(40.6658362042823,-11.8853886402508,-6.78185310726617));
#66924=CARTESIAN_POINT('Ctrl Pts',(40.579898110483,-11.89170784451,-6.73593096961045));
#66925=CARTESIAN_POINT('Ctrl Pts',(40.4918475900371,-11.8980270487692,-6.69407653199056));
#66926=CARTESIAN_POINT('Ctrl Pts',(40.4021092098581,-11.9043462530284,-6.65647004539357));
#66927=CARTESIAN_POINT('Ctrl Pts',(40.3123184430967,-11.9106691462501,-6.61884160525448));
#66928=CARTESIAN_POINT('Ctrl Pts',(40.2208382649942,-11.9169920394717,-6.58546620401095));
#66929=CARTESIAN_POINT('Ctrl Pts',(40.1281099534859,-11.9233149326934,-6.55647468140485));
#66930=CARTESIAN_POINT('Ctrl Pts',(40.0352334573929,-11.9296479302218,-6.52743682886276));
#66931=CARTESIAN_POINT('Ctrl Pts',(39.941105267667,-11.9359809277502,-6.50279695473534));
#66932=CARTESIAN_POINT('Ctrl Pts',(39.8461783926739,-11.9423139252787,-6.48263510772599));
#66933=CARTESIAN_POINT('Ctrl Pts',(39.7912347859215,-11.9459794596786,-6.47096544522459));
#66934=CARTESIAN_POINT('Ctrl Pts',(39.7360237571867,-11.9496449940785,-6.4607949974646));
#66935=CARTESIAN_POINT('Ctrl Pts',(39.6806337417642,-11.9533105284784,-6.45213133063294));
#66936=CARTESIAN_POINT('Ctrl Pts',(39.5849202251457,-11.9596445434634,-6.43716058160992));
#66937=CARTESIAN_POINT('Ctrl Pts',(39.4883410379946,-11.9659785584484,-6.42664011360705));
#66938=CARTESIAN_POINT('Ctrl Pts',(39.3913454556738,-11.9723125734334,-6.42066149244433));
#66939=CARTESIAN_POINT('Ctrl Pts',(39.294480113299,-11.9786380834767,-6.41469089902142));
#66940=CARTESIAN_POINT('Ctrl Pts',(39.1971999196214,-11.98496359352,-6.41325005783559));
#66941=CARTESIAN_POINT('Ctrl Pts',(39.0999625889811,-11.9912891035633,-6.41637921751517));
#66942=CARTESIAN_POINT('Ctrl Pts',(39.0028267741711,-11.9976080097704,-6.4195051103502));
#66943=CARTESIAN_POINT('Ctrl Pts',(38.9057341680089,-12.0039269159775,-6.42719150479397));
#66944=CARTESIAN_POINT('Ctrl Pts',(38.809144825332,-12.0102458221846,-6.43942665208957));
#66945=CARTESIAN_POINT('Ctrl Pts',(38.7126237677838,-12.0165602611563,-6.451653149584));
#66946=CARTESIAN_POINT('Ctrl Pts',(38.6166056987806,-12.0228747001281,-6.46842195190101));
#66947=CARTESIAN_POINT('Ctrl Pts',(38.521546930115,-12.0291891390999,-6.48966936152523));
#66948=CARTESIAN_POINT('Ctrl Pts',(38.4265223544631,-12.035501306743,-6.51090912837251));
#66949=CARTESIAN_POINT('Ctrl Pts',(38.3324568196193,-12.0418134743862,-6.536624206213));
#66950=CARTESIAN_POINT('Ctrl Pts',(38.2397968720151,-12.0481256420294,-6.56669970998413));
#66951=CARTESIAN_POINT('Ctrl Pts',(38.1471451904813,-12.0544372465726,-6.59677253075963));
#66952=CARTESIAN_POINT('Ctrl Pts',(38.0558992625411,-12.0607488511157,-6.63120486891768));
#66953=CARTESIAN_POINT('Ctrl Pts',(37.9664898776547,-12.0670604556588,-6.66983215362533));
#66954=CARTESIAN_POINT('Ctrl Pts',(37.8770642844406,-12.0733732043833,-6.70846644077115));
#66955=CARTESIAN_POINT('Ctrl Pts',(37.7894762967557,-12.0796859531078,-6.75129701150839));
#66956=CARTESIAN_POINT('Ctrl Pts',(37.7041351823981,-12.0859987018324,-6.79811182840939));
#66957=CARTESIAN_POINT('Ctrl Pts',(37.6187028162322,-12.0923182005243,-6.84497670250415));
#66958=CARTESIAN_POINT('Ctrl Pts',(37.5355225036806,-12.0986376992161,-6.89583411745703));
#66959=CARTESIAN_POINT('Ctrl Pts',(37.4549772386612,-12.104957197908,-6.95042698388459));
#66960=CARTESIAN_POINT('Ctrl Pts',(37.3743847570931,-12.1112804011618,-7.00505185327026));
#66961=CARTESIAN_POINT('Ctrl Pts',(37.2964307487401,-12.1176036044155,-7.06341627276901));
#66962=CARTESIAN_POINT('Ctrl Pts',(37.2214659560914,-12.1239268076693,-7.12522215819994));
#66963=CARTESIAN_POINT('Ctrl Pts',(37.1463811192866,-12.1302601365243,-7.18712701589631));
#66964=CARTESIAN_POINT('Ctrl Pts',(37.0742953801205,-12.1365934653793,-7.252484050578));
#66965=CARTESIAN_POINT('Ctrl Pts',(37.0055233541049,-12.1429267942343,-7.32095759942762));
#66966=CARTESIAN_POINT('Ctrl Pts',(36.9657458188551,-12.1465899728023,-7.36056249637255));
#66967=CARTESIAN_POINT('Ctrl Pts',(36.927076136464,-12.1502531513704,-7.40120935512828));
#66968=CARTESIAN_POINT('Ctrl Pts',(36.8895688620344,-12.1539163299384,-7.44282839092957));
#66969=CARTESIAN_POINT('Ctrl Pts',(36.8254868610798,-12.1601749508609,-7.51393542636495));
#66970=CARTESIAN_POINT('Ctrl Pts',(36.764565764203,-12.1664335717834,-7.58814229296622));
#66971=CARTESIAN_POINT('Ctrl Pts',(36.7071249514657,-12.1726921927059,-7.66513316463385));
#66972=CARTESIAN_POINT('Ctrl Pts',(36.649755496101,-12.1789430386907,-7.74202839234961));
#66973=CARTESIAN_POINT('Ctrl Pts',(36.5958580071872,-12.1851938846754,-7.82170040393273));
#66974=CARTESIAN_POINT('Ctrl Pts',(36.5457140776744,-12.1914447306601,-7.90379770064187));
#66975=CARTESIAN_POINT('Ctrl Pts',(36.4956180854176,-12.1976896008785,-7.98581651289304));
#66976=CARTESIAN_POINT('Ctrl Pts',(36.4492687590421,-12.203934471097,-8.07025562599238));
#66977=CARTESIAN_POINT('Ctrl Pts',(36.4069058032,-12.2101793413154,-8.1567326793706));
#66978=CARTESIAN_POINT('Ctrl Pts',(36.3645712237582,-12.2164200284703,-8.2431518069637));
#66979=CARTESIAN_POINT('Ctrl Pts',(36.3262179067279,-12.2226607156251,-8.3316057616338));
#66980=CARTESIAN_POINT('Ctrl Pts',(36.2920401973097,-12.22890140278,-8.42168660896501));
#66981=CARTESIAN_POINT('Ctrl Pts',(36.2578666116568,-12.235141336955,-8.51175658744959));
#66982=CARTESIAN_POINT('Ctrl Pts',(36.2278678053593,-12.2413812711299,-8.6034526550614));
#66983=CARTESIAN_POINT('Ctrl Pts',(36.2021900878147,-12.2476212053048,-8.69634664466751));
#66984=CARTESIAN_POINT('Ctrl Pts',(36.1765154905506,-12.2538603812214,-8.78922934607045));
#66985=CARTESIAN_POINT('Ctrl Pts',(36.155161052167,-12.2600995571379,-8.88330924623595));
#66986=CARTESIAN_POINT('Ctrl Pts',(36.1382228227054,-12.2663387330545,-8.97814428822788));
#66987=CARTESIAN_POINT('Ctrl Pts',(36.1212723595305,-12.2725824152443,-9.07304782526019));
#66988=CARTESIAN_POINT('Ctrl Pts',(36.1087445529449,-12.278826097434,-9.16870715093872));
#66989=CARTESIAN_POINT('Ctrl Pts',(36.1006839684518,-12.2850697796238,-9.26467176586364));
#66990=CARTESIAN_POINT('Ctrl Pts',(36.0933251144286,-12.2907699054448,-9.35228198733494));
#66991=CARTESIAN_POINT('Ctrl Pts',(36.0896889292421,-12.2964700312659,-9.44014631837954));
#66992=CARTESIAN_POINT('Ctrl Pts',(36.0897713719079,-12.3021701570869,-9.52792128330179));
#66993=CARTESIAN_POINT('',(41.0695067500478,-12.749987293334,-12.0106538705994));
#66994=CARTESIAN_POINT('Ctrl Pts',(36.0897713719083,-12.3021701571198,-9.52792128380894));
#66995=CARTESIAN_POINT('Ctrl Pts',(36.0898859550271,-12.3100924880381,-9.64991548889901));
#66996=CARTESIAN_POINT('Ctrl Pts',(36.0971817230537,-12.3180148189564,-9.77159152110514));
#66997=CARTESIAN_POINT('Ctrl Pts',(36.1115251314279,-12.3259371498747,-9.89222423544519));
#66998=CARTESIAN_POINT('Ctrl Pts',(36.1261440100273,-12.3340116319572,-10.015173743683));
#66999=CARTESIAN_POINT('Ctrl Pts',(36.1480838130826,-12.3420861140396,-10.1370396621098));
#67000=CARTESIAN_POINT('Ctrl Pts',(36.1771548843577,-12.3501605961221,-10.2570779055111));
#67001=CARTESIAN_POINT('Ctrl Pts',(36.1823892552886,-12.3516144412142,-10.2786913055096));
#67002=CARTESIAN_POINT('Ctrl Pts',(36.1878546946538,-12.3530682863063,-10.3002455094091));
#67003=CARTESIAN_POINT('Ctrl Pts',(36.1935499325926,-12.3545221313983,-10.3217362456208));
#67004=CARTESIAN_POINT('Ctrl Pts',(36.2184018099668,-12.3608661648413,-10.4155137395126));
#67005=CARTESIAN_POINT('Ctrl Pts',(36.2476880166877,-12.3672101982842,-10.508287686898));
#67006=CARTESIAN_POINT('Ctrl Pts',(36.2813108665629,-12.3735542317272,-10.5996089499237));
#67007=CARTESIAN_POINT('Ctrl Pts',(36.3148883928595,-12.3798897134174,-10.6908071119496));
#67008=CARTESIAN_POINT('Ctrl Pts',(36.3527907932599,-12.3862251951077,-10.7805560766052));
#67009=CARTESIAN_POINT('Ctrl Pts',(36.3948700214694,-12.3925606767979,-10.8684196873832));
#67010=CARTESIAN_POINT('Ctrl Pts',(36.436904991161,-12.3988894948909,-10.9561908840806));
#67011=CARTESIAN_POINT('Ctrl Pts',(36.4831078669681,-12.4052183129839,-11.0420802786785));
#67012=CARTESIAN_POINT('Ctrl Pts',(36.5332820736652,-12.4115471310769,-11.1256705327034));
#67013=CARTESIAN_POINT('Ctrl Pts',(36.5834198380218,-12.4178713524466,-11.2092000737703));
#67014=CARTESIAN_POINT('Ctrl Pts',(36.6375229743783,-12.4241955738163,-11.2904334222201));
#67015=CARTESIAN_POINT('Ctrl Pts',(36.6953488730092,-12.430519795186,-11.3689775988237));
#67016=CARTESIAN_POINT('Ctrl Pts',(36.7531532351144,-12.4368416611793,-11.4474925226406));
#67017=CARTESIAN_POINT('Ctrl Pts',(36.8146773462053,-12.4431635271727,-11.5233199145098));
#67018=CARTESIAN_POINT('Ctrl Pts',(36.8796356676765,-12.449485393166,-11.5960963324242));
#67019=CARTESIAN_POINT('Ctrl Pts',(36.9445872192859,-12.4558066003036,-11.6688651656861));
#67020=CARTESIAN_POINT('Ctrl Pts',(37.0129719793865,-12.4621278074413,-11.7385833324219));
#67021=CARTESIAN_POINT('Ctrl Pts',(37.0844652528387,-12.4684490145789,-11.8049217939336));
#67022=CARTESIAN_POINT('Ctrl Pts',(37.1559702507216,-12.4747712583533,-11.8712711345204));
#67023=CARTESIAN_POINT('Ctrl Pts',(37.2305844550788,-12.4810935021277,-11.9342393728276));
#67024=CARTESIAN_POINT('Ctrl Pts',(37.307948348546,-12.4874157459021,-11.9935362466713));
#67025=CARTESIAN_POINT('Ctrl Pts',(37.3853921374805,-12.4937445188027,-12.0528943577568));
#67026=CARTESIAN_POINT('Ctrl Pts',(37.4655909386642,-12.5000732917032,-12.1085732691621));
#67027=CARTESIAN_POINT('Ctrl Pts',(37.5481545341936,-12.5064020646038,-12.1603248775046));
#67028=CARTESIAN_POINT('Ctrl Pts',(37.6307650023221,-12.5127344304443,-12.2121058660162));
#67029=CARTESIAN_POINT('Ctrl Pts',(37.7157425591651,-12.5190667962847,-12.2599548972531));
#67030=CARTESIAN_POINT('Ctrl Pts',(37.802672363057,-12.5253991621252,-12.3036698486749));
#67031=CARTESIAN_POINT('Ctrl Pts',(37.8897375398657,-12.5317413891501,-12.347452875949));
#67032=CARTESIAN_POINT('Ctrl Pts',(37.9787606369115,-12.5380836161751,-12.387088790452));
#67033=CARTESIAN_POINT('Ctrl Pts',(38.0693068804957,-12.5444258432,-12.4224236353018));
#67034=CARTESIAN_POINT('Ctrl Pts',(38.1202371511642,-12.5479932064195,-12.4422987084246));
#67035=CARTESIAN_POINT('Ctrl Pts',(38.171649027407,-12.5515605696389,-12.4608139017796));
#67036=CARTESIAN_POINT('Ctrl Pts',(38.2234634008129,-12.5551279328584,-12.4779488521388));
#67037=CARTESIAN_POINT('Ctrl Pts',(38.3150843011274,-12.5614359321341,-12.5082477726036));
#67038=CARTESIAN_POINT('Ctrl Pts',(38.4082797221892,-12.5677439314098,-12.534332451525));
#67039=CARTESIAN_POINT('Ctrl Pts',(38.5026246672537,-12.5740519306855,-12.556039144943));
#67040=CARTESIAN_POINT('Ctrl Pts',(38.5968442865265,-12.5803515505509,-12.5777170036573));
#67041=CARTESIAN_POINT('Ctrl Pts',(38.6922099691279,-12.5866511704163,-12.5950283357082));
#67042=CARTESIAN_POINT('Ctrl Pts',(38.7882798848438,-12.5929507902817,-12.607858608447));
#67043=CARTESIAN_POINT('Ctrl Pts',(38.8880642364851,-12.5994939779089,-12.6211849493424));
#67044=CARTESIAN_POINT('Ctrl Pts',(38.9886079299138,-12.6060371655361,-12.6296765276222));
#67045=CARTESIAN_POINT('Ctrl Pts',(39.0894019424228,-12.6125803531633,-12.6332629751294));
#67046=CARTESIAN_POINT('Ctrl Pts',(39.1862778293985,-12.6188691900619,-12.63671000809));
#67047=CARTESIAN_POINT('Ctrl Pts',(39.2833844506666,-12.6251580269606,-12.6356261437977));
#67048=CARTESIAN_POINT('Ctrl Pts',(39.3802641991579,-12.6314468638593,-12.6300016862156));
#67049=CARTESIAN_POINT('Ctrl Pts',(39.4771131819549,-12.6377337036385,-12.6243790147689));
#67050=CARTESIAN_POINT('Ctrl Pts',(39.5737349951434,-12.6440205434176,-12.6142186404297));
#67051=CARTESIAN_POINT('Ctrl Pts',(39.6696735849597,-12.6503073831968,-12.5995629569893));
#67052=CARTESIAN_POINT('Ctrl Pts',(39.7656082253187,-12.6565939641687,-12.5849078768724));
#67053=CARTESIAN_POINT('Ctrl Pts',(39.860859262293,-12.6628805451406,-12.565757922853));
#67054=CARTESIAN_POINT('Ctrl Pts',(39.9549784023291,-12.6691671261125,-12.542207030503));
#67055=CARTESIAN_POINT('Ctrl Pts',(40.0491196823481,-12.6754551858994,-12.5186505981921));
#67056=CARTESIAN_POINT('Ctrl Pts',(40.1421281089206,-12.6817432456863,-12.4906912788937));
#67057=CARTESIAN_POINT('Ctrl Pts',(40.2335692412759,-12.6880313054732,-12.4584732445325));
#67058=CARTESIAN_POINT('Ctrl Pts',(40.3251097880169,-12.6943262016102,-12.4262201828701));
#67059=CARTESIAN_POINT('Ctrl Pts',(40.415079223903,-12.7006210977473,-12.389699313691));
#67060=CARTESIAN_POINT('Ctrl Pts',(40.5030621364958,-12.7069159938843,-12.3491033482029));
#67061=CARTESIAN_POINT('Ctrl Pts',(40.5911018509854,-12.7132149540155,-12.3084811739003));
#67062=CARTESIAN_POINT('Ctrl Pts',(40.6771520989339,-12.7195139141467,-12.2637788700992));
#67063=CARTESIAN_POINT('Ctrl Pts',(40.7608230186359,-12.7258128742779,-12.2152345915173));
#67064=CARTESIAN_POINT('Ctrl Pts',(40.8446201610862,-12.7321213367794,-12.166617080894));
#67065=CARTESIAN_POINT('Ctrl Pts',(40.9260304439932,-12.7384297992808,-12.1141462693586));
#67066=CARTESIAN_POINT('Ctrl Pts',(41.0046941210115,-12.7447382617822,-12.0581027974574));
#67067=CARTESIAN_POINT('Ctrl Pts',(41.0265118049324,-12.7464879389662,-12.0425589174595));
#67068=CARTESIAN_POINT('Ctrl Pts',(41.0481184108033,-12.7482376161501,-12.0267404404404));
#67069=CARTESIAN_POINT('Ctrl Pts',(41.0695067500478,-12.749987293334,-12.0106538705994));
#67070=CARTESIAN_POINT('',(38.2853957334119,-12.75,-12.4977141955524));
#67071=CARTESIAN_POINT('Origin',(39.2,-12.75,-9.525));
#67072=CARTESIAN_POINT('',(36.0919483849455,-12.4928298429131,-9.52879526530289));
#67073=CARTESIAN_POINT('Ctrl Pts',(38.2853957334118,-12.75,-12.4977141955524));
#67074=CARTESIAN_POINT('Ctrl Pts',(37.3019474236971,-12.6831313995133,-12.1951401972246));
#67075=CARTESIAN_POINT('Ctrl Pts',(36.2593719387647,-12.5974080138178,-11.1359917255917));
#67076=CARTESIAN_POINT('Ctrl Pts',(36.0895541491445,-12.5116846281221,-9.81920730742513));
#67077=CARTESIAN_POINT('Ctrl Pts',(36.0919483849455,-12.4928298429131,-9.52879526530289));
#67078=CARTESIAN_POINT('',(36.0900673707834,-11.222829801326,-9.52326984187138));
#67079=CARTESIAN_POINT('Ctrl Pts',(36.0919483849455,-12.4928298429131,-9.52879526530289));
#67080=CARTESIAN_POINT('Ctrl Pts',(36.0980453197133,-12.4448160276354,-8.78925938672623));
#67081=CARTESIAN_POINT('Ctrl Pts',(36.7293203004083,-12.3299336118711,-7.0075733048701));
#67082=CARTESIAN_POINT('Ctrl Pts',(39.6920471758748,-12.14818259562,-5.88918093587763));
#67083=CARTESIAN_POINT('Ctrl Pts',(42.5136842856469,-11.94757679416,-7.94804692653049));
#67084=CARTESIAN_POINT('Ctrl Pts',(42.3317557451001,-11.7469709927,-11.4386305882703));
#67085=CARTESIAN_POINT('Ctrl Pts',(39.3094778593138,-11.5463651912402,-13.1930895342595));
#67086=CARTESIAN_POINT('Ctrl Pts',(36.59108955988,-11.3716514746445,-11.8247205883103));
#67087=CARTESIAN_POINT('Ctrl Pts',(36.096963550306,-11.2638063585355,-10.1556712558172));
#67088=CARTESIAN_POINT('Ctrl Pts',(36.0937128061288,-11.2228298429131,-9.52327251182905));
#67089=CARTESIAN_POINT('',(36.0897701688195,-9.95282984294777,-9.52397523911836));
#67090=CARTESIAN_POINT('Ctrl Pts',(36.089770481347,-11.2228297979391,-9.52326962442624));
#67091=CARTESIAN_POINT('Ctrl Pts',(36.0898309229459,-11.2157993567217,-9.41463006205864));
#67092=CARTESIAN_POINT('Ctrl Pts',(36.0955876081903,-11.2087689155044,-9.30619309129701));
#67093=CARTESIAN_POINT('Ctrl Pts',(36.1069524548467,-11.201738474287,-9.19852253321102));
#67094=CARTESIAN_POINT('Ctrl Pts',(36.1183588864254,-11.1946823080986,-9.09045799956816));
#67095=CARTESIAN_POINT('Ctrl Pts',(36.1354144747909,-11.1876261419101,-8.98316573382048));
#67096=CARTESIAN_POINT('Ctrl Pts',(36.1579801913597,-11.1805699757217,-8.87719899912097));
#67097=CARTESIAN_POINT('Ctrl Pts',(36.1806584687337,-11.1734786124347,-8.77070368820889));
#67098=CARTESIAN_POINT('Ctrl Pts',(36.2089018643949,-11.1663872491478,-8.66554739650279));
#67099=CARTESIAN_POINT('Ctrl Pts',(36.2425206599758,-11.1592958858608,-8.56227127069456));
#67100=CARTESIAN_POINT('Ctrl Pts',(36.2648693015945,-11.1545817866806,-8.49361678490559));
#67101=CARTESIAN_POINT('Ctrl Pts',(36.2895924108059,-11.1498676875004,-8.42579274376721));
#67102=CARTESIAN_POINT('Ctrl Pts',(36.3166228666883,-11.1451535883202,-8.35895241949765));
#67103=CARTESIAN_POINT('Ctrl Pts',(36.3529354112524,-11.1388206971065,-8.26915954792089));
#67104=CARTESIAN_POINT('Ctrl Pts',(36.3935094163776,-11.1324878058927,-8.18090867255315));
#67105=CARTESIAN_POINT('Ctrl Pts',(36.4381928691988,-11.126154914679,-8.09463220633452));
#67106=CARTESIAN_POINT('Ctrl Pts',(36.4828162017387,-11.1198305441855,-8.00847182258245));
#67107=CARTESIAN_POINT('Ctrl Pts',(36.5315377931203,-11.113506173692,-7.92428095303794));
#67108=CARTESIAN_POINT('Ctrl Pts',(36.5841572587825,-11.1071818031986,-7.84247291073221));
#67109=CARTESIAN_POINT('Ctrl Pts',(36.6367216630998,-11.1008640505668,-7.76075047288447));
#67110=CARTESIAN_POINT('Ctrl Pts',(36.6931755975997,-11.0945462979349,-7.6814062710863));
#67111=CARTESIAN_POINT('Ctrl Pts',(36.753272853838,-11.0882285453031,-7.60482893336719));
#67112=CARTESIAN_POINT('Ctrl Pts',(36.8133274642926,-11.0819152758296,-7.52830593590889));
#67113=CARTESIAN_POINT('Ctrl Pts',(36.8770199874541,-11.0756020063561,-7.4545462421718));
#67114=CARTESIAN_POINT('Ctrl Pts',(36.9440615576594,-11.0692887368826,-7.38390859670361));
#67115=CARTESIAN_POINT('Ctrl Pts',(37.0110789088195,-11.0629777481038,-7.31329646937764));
#67116=CARTESIAN_POINT('Ctrl Pts',(37.0814426023051,-11.0566667593251,-7.24580446610108));
#67117=CARTESIAN_POINT('Ctrl Pts',(37.1548248613583,-11.0503557705463,-7.1817566696602));
#67118=CARTESIAN_POINT('Ctrl Pts',(37.2282004815662,-11.0440453527186,-7.11771466758188));
#67119=CARTESIAN_POINT('Ctrl Pts',(37.3045937948049,-11.0377349348909,-7.05711654018844));
#67120=CARTESIAN_POINT('Ctrl Pts',(37.3836424801294,-11.0314245170632,-7.00024733629027));
#67121=CARTESIAN_POINT('Ctrl Pts',(37.4627054188214,-11.0251129613961,-6.9433678782346));
#67122=CARTESIAN_POINT('Ctrl Pts',(37.5444243255732,-11.0188014057291,-6.89021893441362));
#67123=CARTESIAN_POINT('Ctrl Pts',(37.6284072016717,-11.012489850062,-6.84104271100627));
#67124=CARTESIAN_POINT('Ctrl Pts',(37.7124798640876,-11.0061715466939,-6.79181391316701));
#67125=CARTESIAN_POINT('Ctrl Pts',(37.7988209501189,-10.9998532433258,-6.7465665364544));
#67126=CARTESIAN_POINT('Ctrl Pts',(37.8870132974164,-10.9935349399577,-6.70549710556298));
#67127=CARTESIAN_POINT('Ctrl Pts',(37.9752573118236,-10.9872129350386,-6.66440361432102));
#67128=CARTESIAN_POINT('Ctrl Pts',(38.0653543426938,-10.9808909301195,-6.62749310851382));
#67129=CARTESIAN_POINT('Ctrl Pts',(38.1568686178513,-10.9745689252004,-6.59491338481667));
#67130=CARTESIAN_POINT('Ctrl Pts',(38.2485295699489,-10.9682367875196,-6.56228144310026));
#67131=CARTESIAN_POINT('Ctrl Pts',(38.3416118840624,-10.9619046498389,-6.53399427107727));
#67132=CARTESIAN_POINT('Ctrl Pts',(38.4356661006116,-10.9555725121581,-6.51014936636229));
#67133=CARTESIAN_POINT('Ctrl Pts',(38.4902512424626,-10.9518976037254,-6.49631077885345));
#67134=CARTESIAN_POINT('Ctrl Pts',(38.5451635539952,-10.9482226952928,-6.48396745765534));
#67135=CARTESIAN_POINT('Ctrl Pts',(38.6003142679106,-10.9445477868601,-6.47313046222019));
#67136=CARTESIAN_POINT('Ctrl Pts',(38.6953519381646,-10.9382150540441,-6.45445576654372));
#67137=CARTESIAN_POINT('Ctrl Pts',(38.7914277571371,-10.9318823212281,-6.44019219959787));
#67138=CARTESIAN_POINT('Ctrl Pts',(38.8880965579976,-10.9255495884122,-6.43044883775255));
#67139=CARTESIAN_POINT('Ctrl Pts',(38.9846353012854,-10.9192253756135,-6.42071858456255));
#67140=CARTESIAN_POINT('Ctrl Pts',(39.0817650093881,-10.9129011628148,-6.41549649276756));
#67141=CARTESIAN_POINT('Ctrl Pts',(39.1790300674642,-10.9065769500162,-6.41484069301435));
#67142=CARTESIAN_POINT('Ctrl Pts',(39.2761933584161,-10.9002593541565,-6.41418557941563));
#67143=CARTESIAN_POINT('Ctrl Pts',(39.3734912828146,-10.8939417582968,-6.41808726258191));
#67144=CARTESIAN_POINT('Ctrl Pts',(39.4704638476505,-10.887624162437,-6.42655200785715));
#67145=CARTESIAN_POINT('Ctrl Pts',(39.5673676294268,-10.8813110476754,-6.43501074905195));
#67146=CARTESIAN_POINT('Ctrl Pts',(39.6639460760389,-10.8749979329137,-6.44802607988394));
#67147=CARTESIAN_POINT('Ctrl Pts',(39.7597409005073,-10.8686848181521,-6.46555221041456));
#67148=CARTESIAN_POINT('Ctrl Pts',(39.8555011381581,-10.8623739827468,-6.48307201311813));
#67149=CARTESIAN_POINT('Ctrl Pts',(39.9504778861266,-10.8560631473416,-6.50509930079477));
#67150=CARTESIAN_POINT('Ctrl Pts',(40.0442206129504,-10.8497523119364,-6.53153675326226));
#67151=CARTESIAN_POINT('Ctrl Pts',(40.137954881549,-10.8434420459457,-6.55797182032949));
#67152=CARTESIAN_POINT('Ctrl Pts',(40.2304549295605,-10.8371317799549,-6.58881614213147));
#67153=CARTESIAN_POINT('Ctrl Pts',(40.3212840296132,-10.8308215139642,-6.62392213516521));
#67154=CARTESIAN_POINT('Ctrl Pts',(40.4121295325585,-10.824510108398,-6.65903446801553));
#67155=CARTESIAN_POINT('Ctrl Pts',(40.5013030803449,-10.8181987028317,-6.69840984297876));
#67156=CARTESIAN_POINT('Ctrl Pts',(40.5883875993672,-10.8118872972655,-6.74185240656854));
#67157=CARTESIAN_POINT('Ctrl Pts',(40.6755652724881,-10.8055691404041,-6.78534144056311));
#67158=CARTESIAN_POINT('Ctrl Pts',(40.7606490635793,-10.7992509835427,-6.83290615351406));
#67159=CARTESIAN_POINT('Ctrl Pts',(40.8432463974884,-10.7929328266812,-6.8843046502784));
#67160=CARTESIAN_POINT('Ctrl Pts',(40.9258921455622,-10.7866109664522,-6.93573327410819));
#67161=CARTESIAN_POINT('Ctrl Pts',(41.006048174458,-10.7802891062233,-6.99099990834741));
#67162=CARTESIAN_POINT('Ctrl Pts',(41.0833525415978,-10.7739672459943,-7.0498204394515));
#67163=CARTESIAN_POINT('Ctrl Pts',(41.1607808659939,-10.7676352486867,-7.10873528905162));
#67164=CARTESIAN_POINT('Ctrl Pts',(41.2353480629236,-10.761303251379,-7.17121513406714));
#67165=CARTESIAN_POINT('Ctrl Pts',(41.3067268284427,-10.7549712540714,-7.23693690576073));
#67166=CARTESIAN_POINT('Ctrl Pts',(41.3481700752881,-10.751294831181,-7.27509564369365));
#67167=CARTESIAN_POINT('Ctrl Pts',(41.3885391791425,-10.7476184082906,-7.31434658483823));
#67168=CARTESIAN_POINT('Ctrl Pts',(41.4277762873863,-10.7439419854002,-7.35462135417361));
#67169=CARTESIAN_POINT('Ctrl Pts',(41.4953605833667,-10.7376094990398,-7.42399297846341));
#67170=CARTESIAN_POINT('Ctrl Pts',(41.5598189499684,-10.7312770126794,-7.49664495904801));
#67171=CARTESIAN_POINT('Ctrl Pts',(41.6208167091706,-10.724944526319,-7.57226419772146));
#67172=CARTESIAN_POINT('Ctrl Pts',(41.6817323540334,-10.7186205646641,-7.6477816388222));
#67173=CARTESIAN_POINT('Ctrl Pts',(41.7391963784556,-10.7122966030092,-7.72625806128481));
#67174=CARTESIAN_POINT('Ctrl Pts',(41.7929110505019,-10.7059726413543,-7.80734376632425));
#67175=CARTESIAN_POINT('Ctrl Pts',(41.8465694827374,-10.6996553009519,-7.88834457380142));
#67176=CARTESIAN_POINT('Ctrl Pts',(41.8964861266362,-10.6933379605496,-7.97194886994616));
#67177=CARTESIAN_POINT('Ctrl Pts',(41.9424042851038,-10.6870206201472,-8.05777493548391));
#67178=CARTESIAN_POINT('Ctrl Pts',(41.9882898331519,-10.6807077662296,-8.14354004857711));
#67179=CARTESIAN_POINT('Ctrl Pts',(42.0301823354706,-10.6743949123121,-8.23152340964769));
#67180=CARTESIAN_POINT('Ctrl Pts',(42.0678696155352,-10.6680820583945,-8.32131627028119));
#67181=CARTESIAN_POINT('Ctrl Pts',(42.1055432686988,-10.6617714870677,-8.41107666376871));
#67182=CARTESIAN_POINT('Ctrl Pts',(42.1390145518075,-10.6554609157409,-8.50264485392143));
#67183=CARTESIAN_POINT('Ctrl Pts',(42.1681186764902,-10.649150344414,-8.59559041581756));
#67184=CARTESIAN_POINT('Ctrl Pts',(42.1972201616111,-10.6428403454165,-8.68852754813379));
#67185=CARTESIAN_POINT('Ctrl Pts',(42.2219551453044,-10.6365303464189,-8.78284138641357));
#67186=CARTESIAN_POINT('Ctrl Pts',(42.2422084733341,-10.6302203474213,-8.87808558705612));
#67187=CARTESIAN_POINT('Ctrl Pts',(42.2624654507439,-10.6239092114459,-8.97334694943624));
#67188=CARTESIAN_POINT('Ctrl Pts',(42.2782390776999,-10.6175980754705,-9.0695385793586));
#67189=CARTESIAN_POINT('Ctrl Pts',(42.2894653629619,-10.611286939495,-9.16620420298098));
#67190=CARTESIAN_POINT('Ctrl Pts',(42.3007036532935,-10.6049690545707,-9.26297319806607));
#67191=CARTESIAN_POINT('Ctrl Pts',(42.3073848430886,-10.5986511696463,-9.36021676366926));
#67192=CARTESIAN_POINT('Ctrl Pts',(42.3094968866886,-10.592333284722,-9.45747397113558));
#67193=CARTESIAN_POINT('Ctrl Pts',(42.3116101677337,-10.5860116981524,-9.55478816154437));
#67194=CARTESIAN_POINT('Ctrl Pts',(42.3091489828831,-10.5796901115829,-9.65211557273019));
#67195=CARTESIAN_POINT('Ctrl Pts',(42.3021533838499,-10.5733685250134,-9.74899784813421));
#67196=CARTESIAN_POINT('Ctrl Pts',(42.295146566964,-10.5670368014096,-9.84603547993994));
#67197=CARTESIAN_POINT('Ctrl Pts',(42.2835908685082,-10.5607050778058,-9.94262611666422));
#67198=CARTESIAN_POINT('Ctrl Pts',(42.2675778949649,-10.5543733542021,-10.0383191124656));
#67199=CARTESIAN_POINT('Ctrl Pts',(42.2582735345488,-10.5506942974481,-10.093921659977));
#67200=CARTESIAN_POINT('Ctrl Pts',(42.2474652583428,-10.5470152406942,-10.1492213645));
#67201=CARTESIAN_POINT('Ctrl Pts',(42.2351787567165,-10.5433361839402,-10.2041322166387));
#67202=CARTESIAN_POINT('Ctrl Pts',(42.2140303184225,-10.5370035184584,-10.2986488498879));
#67203=CARTESIAN_POINT('Ctrl Pts',(42.1884260203412,-10.5306708529766,-10.392340839025));
#67204=CARTESIAN_POINT('Ctrl Pts',(42.1584451326556,-10.5243381874949,-10.4847567660436));
#67205=CARTESIAN_POINT('Ctrl Pts',(42.1285045921532,-10.5180140442829,-10.5770483230842));
#67206=CARTESIAN_POINT('Ctrl Pts',(42.0941993022163,-10.5116899010709,-10.6680668187252));
#67207=CARTESIAN_POINT('Ctrl Pts',(42.0556593764814,-10.505365757859,-10.7573717695623));
#67208=CARTESIAN_POINT('Ctrl Pts',(42.0171597880662,-10.4990482337305,-10.8465832505161));
#67209=CARTESIAN_POINT('Ctrl Pts',(41.9744345475036,-10.4927307096021,-10.934084352748));
#67210=CARTESIAN_POINT('Ctrl Pts',(41.9276630113239,-10.4864131854736,-11.019451454399));
#67211=CARTESIAN_POINT('Ctrl Pts',(41.8809246723569,-10.4801001453585,-11.1047579647148));
#67212=CARTESIAN_POINT('Ctrl Pts',(41.8301459569201,-10.4737871052434,-11.1879331032524));
#67213=CARTESIAN_POINT('Ctrl Pts',(41.7755531900407,-10.4674740651283,-11.2685757563614));
#67214=CARTESIAN_POINT('Ctrl Pts',(41.7209801495324,-10.4611633061464,-11.3491892703188));
#67215=CARTESIAN_POINT('Ctrl Pts',(41.6625960408975,-10.4548525471645,-11.4272717553604));
#67216=CARTESIAN_POINT('Ctrl Pts',(41.6006712428079,-10.4485417881826,-11.5024499328314));
#67217=CARTESIAN_POINT('Ctrl Pts',(41.5387520486998,-10.4422316003026,-11.5776213069357));
#67218=CARTESIAN_POINT('Ctrl Pts',(41.4732930804004,-10.4359214124227,-11.64988855863));
#67219=CARTESIAN_POINT('Ctrl Pts',(41.4046051764515,-10.4296112245428,-11.7189112718757));
#67220=CARTESIAN_POINT('Ctrl Pts',(41.3359048853634,-10.4232998986871,-11.78794643264));
#67221=CARTESIAN_POINT('Ctrl Pts',(41.2639748105852,-10.4169885728313,-11.8537355828928));
#67222=CARTESIAN_POINT('Ctrl Pts',(41.1891620717469,-10.4106772469755,-11.9159757224246));
#67223=CARTESIAN_POINT('Ctrl Pts',(41.1142693282935,-10.4043591717987,-11.9782824214551));
#67224=CARTESIAN_POINT('Ctrl Pts',(41.0364881030367,-10.3980410966219,-12.037032252502));
#67225=CARTESIAN_POINT('Ctrl Pts',(40.9561978070758,-10.391723021445,-12.0919631698414));
#67226=CARTESIAN_POINT('Ctrl Pts',(40.8758604642909,-10.385401244135,-12.146926274448));
#67227=CARTESIAN_POINT('Ctrl Pts',(40.7930114951643,-10.3790794668249,-12.1980657798235));
#67228=CARTESIAN_POINT('Ctrl Pts',(40.7080566338598,-10.3727576895149,-12.2451646718483));
#67229=CARTESIAN_POINT('Ctrl Pts',(40.6229655613931,-10.3664257762736,-12.2923390792081));
#67230=CARTESIAN_POINT('Ctrl Pts',(40.5357622463171,-10.3600938630323,-12.3354597431534));
#67231=CARTESIAN_POINT('Ctrl Pts',(40.4468741463487,-10.3537619497909,-12.3743570355551));
#67232=CARTESIAN_POINT('Ctrl Pts',(40.3952533580996,-10.3500847606874,-12.3969462111055));
#67233=CARTESIAN_POINT('Ctrl Pts',(40.3430646999005,-10.3464075715838,-12.4181119386258));
#67234=CARTESIAN_POINT('Ctrl Pts',(40.2903941024023,-10.3427303824802,-12.4378287547239));
#67235=CARTESIAN_POINT('Ctrl Pts',(40.1996880264142,-10.3363977527002,-12.4717838473977));
#67236=CARTESIAN_POINT('Ctrl Pts',(40.107236841428,-10.3300651229201,-12.5015569736709));
#67237=CARTESIAN_POINT('Ctrl Pts',(40.0134618815896,-10.32373249314,-12.5269677580049));
#67238=CARTESIAN_POINT('Ctrl Pts',(39.9198131233972,-10.3174083857661,-12.5523443446936));
#67239=CARTESIAN_POINT('Ctrl Pts',(39.8248445497447,-10.3110842783923,-12.5733701445375));
#67240=CARTESIAN_POINT('Ctrl Pts',(39.7289961307342,-10.3047601710184,-12.5899133342671));
#67241=CARTESIAN_POINT('Ctrl Pts',(39.6332480321042,-10.2984426828133,-12.606439208958));
#67242=CARTESIAN_POINT('Ctrl Pts',(39.5366223475779,-10.2921251946082,-12.6184917269789));
#67243=CARTESIAN_POINT('Ctrl Pts',(39.4395718451484,-10.2858077064031,-12.6259895168982));
#67244=CARTESIAN_POINT('Ctrl Pts',(39.3425902266162,-10.2794947021852,-12.6334819850831));
#67245=CARTESIAN_POINT('Ctrl Pts',(39.2451848244055,-10.2731816979672,-12.636426118629));
#67246=CARTESIAN_POINT('Ctrl Pts',(39.1478152327065,-10.2668686937493,-12.6347921800279));
#67247=CARTESIAN_POINT('Ctrl Pts',(39.0504808239462,-10.2605579706341,-12.6331588318243));
#67248=CARTESIAN_POINT('Ctrl Pts',(38.9531826367933,-10.2542472475189,-12.6269507057427));
#67249=CARTESIAN_POINT('Ctrl Pts',(38.856381037686,-10.2479365244037,-12.6161901691158));
#67250=CARTESIAN_POINT('Ctrl Pts',(38.7595881976793,-10.2416263723147,-12.6054306061569));
#67251=CARTESIAN_POINT('Ctrl Pts',(38.663292290989,-10.2353162202258,-12.5901195001764));
#67252=CARTESIAN_POINT('Ctrl Pts',(38.5679482817613,-10.2290060681369,-12.5703310621953));
#67253=CARTESIAN_POINT('Ctrl Pts',(38.4725870763213,-10.2226947779512,-12.5505390551784));
#67254=CARTESIAN_POINT('Ctrl Pts',(38.3781785375033,-10.2163834877655,-12.5262682012066));
#67255=CARTESIAN_POINT('Ctrl Pts',(38.285166130107,-10.2100721975797,-12.4976435446243));
#67256=CARTESIAN_POINT('Ctrl Pts',(38.1920542488689,-10.2037541576678,-12.4689882748729));
#67257=CARTESIAN_POINT('Ctrl Pts',(38.1003418986366,-10.1974361177559,-12.4359700353948));
#67258=CARTESIAN_POINT('Ctrl Pts',(38.0104559008266,-10.191118077844,-12.3987632973197));
#67259=CARTESIAN_POINT('Ctrl Pts',(37.9205172306873,-10.1847963356215,-12.3615347564543));
#67260=CARTESIAN_POINT('Ctrl Pts',(37.8324074396652,-10.178474593399,-12.3201130155421));
#67261=CARTESIAN_POINT('Ctrl Pts',(37.7465300291259,-10.1721528511766,-12.2747192032401));
#67262=CARTESIAN_POINT('Ctrl Pts',(37.6605149189724,-10.1658209723948,-12.2292526045044));
#67263=CARTESIAN_POINT('Ctrl Pts',(37.5767397132873,-10.159489093613,-12.1798014387739));
#67264=CARTESIAN_POINT('Ctrl Pts',(37.4955801076958,-10.1531572148312,-12.1266309276333));
#67265=CARTESIAN_POINT('Ctrl Pts',(37.4484427445428,-10.1494796702275,-12.0957495837134));
#67266=CARTESIAN_POINT('Ctrl Pts',(37.4021871093497,-10.1458021256239,-12.0636143887629));
#67267=CARTESIAN_POINT('Ctrl Pts',(37.3568815158417,-10.1421245810202,-12.0302833983911));
#67268=CARTESIAN_POINT('Ctrl Pts',(37.2795150877967,-10.1358445950862,-11.9733654889544));
#67269=CARTESIAN_POINT('Ctrl Pts',(37.2046422003673,-10.1295646091522,-11.9127532616935));
#67270=CARTESIAN_POINT('Ctrl Pts',(37.1326407205089,-10.1232846232183,-11.8486945286337));
#67271=CARTESIAN_POINT('Ctrl Pts',(37.0607364833283,-10.1170131188134,-11.7847223110559));
#67272=CARTESIAN_POINT('Ctrl Pts',(36.9916962788464,-10.1107416144085,-11.7173131289113));
#67273=CARTESIAN_POINT('Ctrl Pts',(36.9258678285865,-10.1044701100037,-11.6467571773986));
#67274=CARTESIAN_POINT('Ctrl Pts',(36.8595477246366,-10.098151765543,-11.5756742638537));
#67275=CARTESIAN_POINT('Ctrl Pts',(36.7964879299382,-10.0918334210823,-11.5013976382766));
#67276=CARTESIAN_POINT('Ctrl Pts',(36.7370090233934,-10.0855150766217,-11.4242646213875));
#67277=CARTESIAN_POINT('Ctrl Pts',(36.6780731830441,-10.0792544211719,-11.3478358597793));
#67278=CARTESIAN_POINT('Ctrl Pts',(36.6226533882408,-10.0729937657222,-11.2686030111864));
#67279=CARTESIAN_POINT('Ctrl Pts',(36.5710225829619,-10.0667331102724,-11.1869291181046));
#67280=CARTESIAN_POINT('Ctrl Pts',(36.5194087470668,-10.0604745124986,-11.1052820686024));
#67281=CARTESIAN_POINT('Ctrl Pts',(36.4715816646951,-10.0542159147247,-11.0211959445787));
#67282=CARTESIAN_POINT('Ctrl Pts',(36.4277710784546,-10.0479573169509,-10.9350629274778));
#67283=CARTESIAN_POINT('Ctrl Pts',(36.3839625177518,-10.041699008537,-10.848933892649));
#67284=CARTESIAN_POINT('Ctrl Pts',(36.3441702851032,-10.035440700123,-10.7607585503843));
#67285=CARTESIAN_POINT('Ctrl Pts',(36.3085777172643,-10.0291823917091,-10.6709528069686));
#67286=CARTESIAN_POINT('Ctrl Pts',(36.2723913778188,-10.0228196793123,-10.5796488827869));
#67287=CARTESIAN_POINT('Ctrl Pts',(36.2405462905674,-10.0164569669155,-10.4866600999831));
#67288=CARTESIAN_POINT('Ctrl Pts',(36.2131831840949,-10.0100942545187,-10.3924421946889));
#67289=CARTESIAN_POINT('Ctrl Pts',(36.1862342561534,-10.0038278505903,-10.2996504079402));
#67290=CARTESIAN_POINT('Ctrl Pts',(36.1636326108138,-9.99756144666187,-10.2056669037343));
#67291=CARTESIAN_POINT('Ctrl Pts',(36.1454612557528,-9.99129504273344,-10.1109383182494));
#67292=CARTESIAN_POINT('Ctrl Pts',(36.1268709868953,-9.9848841761025,-10.0140259049072));
#67293=CARTESIAN_POINT('Ctrl Pts',(36.1129178675833,-9.97847330947155,-9.91633412434151));
#67294=CARTESIAN_POINT('Ctrl Pts',(36.1036345934322,-9.9720624428406,-9.81834607873639));
#67295=CARTESIAN_POINT('Ctrl Pts',(36.094351319281,-9.96565157620966,-9.7203580331313));
#67296=CARTESIAN_POINT('Ctrl Pts',(36.0897378470939,-9.95924070957871,-9.62207421712648));
#67297=CARTESIAN_POINT('Ctrl Pts',(36.0897701688195,-9.95282984294777,-9.52397523911838));
#67298=CARTESIAN_POINT('',(36.0897711821211,-8.68282986586788,-9.52771170347425));
#67299=CARTESIAN_POINT('Ctrl Pts',(36.0897701688197,-9.95282984291314,-9.52397523858839));
#67300=CARTESIAN_POINT('Ctrl Pts',(36.0897891778604,-9.94905948846218,-9.46628133546143));
#67301=CARTESIAN_POINT('Ctrl Pts',(36.091413392757,-9.94528913401121,-9.40861613371628));
#67302=CARTESIAN_POINT('Ctrl Pts',(36.0946386559873,-9.94151877956024,-9.35104145317981));
#67303=CARTESIAN_POINT('Ctrl Pts',(36.1000557567198,-9.9351861522987,-9.25433993710724));
#67304=CARTESIAN_POINT('Ctrl Pts',(36.1100035216219,-9.92885352503716,-9.15772373237964));
#67305=CARTESIAN_POINT('Ctrl Pts',(36.1244775265326,-9.92252089777562,-9.06165113780548));
#67306=CARTESIAN_POINT('Ctrl Pts',(36.1389320519434,-9.91619679313193,-8.96570784027888));
#67307=CARTESIAN_POINT('Ctrl Pts',(36.1579006455556,-9.90987268848823,-8.87030712758677));
#67308=CARTESIAN_POINT('Ctrl Pts',(36.1813269362864,-9.90354858384453,-8.77590482092732));
#67309=CARTESIAN_POINT('Ctrl Pts',(36.2047287069587,-9.8972310985764,-8.68160132419543));
#67310=CARTESIAN_POINT('Ctrl Pts',(36.2325787940897,-9.89091361330827,-8.58829457815231));
#67311=CARTESIAN_POINT('Ctrl Pts',(36.2647694900105,-9.88459612804013,-8.49643181746348));
#67312=CARTESIAN_POINT('Ctrl Pts',(36.2969373362904,-9.87828312705746,-8.40463426291674));
#67313=CARTESIAN_POINT('Ctrl Pts',(36.3334395218242,-9.87197012607479,-8.31427906755525));
#67314=CARTESIAN_POINT('Ctrl Pts',(36.3741183233008,-9.86565712509212,-8.22579893696325));
#67315=CARTESIAN_POINT('Ctrl Pts',(36.4147824249554,-9.8593464053957,-8.13735077983468));
#67316=CARTESIAN_POINT('Ctrl Pts',(36.4596199611181,-9.85303568569929,-8.05077673804627));
#67317=CARTESIAN_POINT('Ctrl Pts',(36.5084251979139,-9.84672496600288,-7.96648925647748));
#67318=CARTESIAN_POINT('Ctrl Pts',(36.5572260171697,-9.84041481751273,-7.88220940407609));
#67319=CARTESIAN_POINT('Ctrl Pts',(36.6099936037103,-9.83410466902258,-7.80021607874136));
#67320=CARTESIAN_POINT('Ctrl Pts',(36.6664769368874,-9.82779452053243,-7.72089591719979));
#67321=CARTESIAN_POINT('Ctrl Pts',(36.7229704558046,-9.82148323412194,-7.64156145171203));
#67322=CARTESIAN_POINT('Ctrl Pts',(36.7831807985061,-9.81517194771146,-7.56490146364139));
#67323=CARTESIAN_POINT('Ctrl Pts',(36.8468150360541,-9.80886066130098,-7.49127160654161));
#67324=CARTESIAN_POINT('Ctrl Pts',(36.9105173259497,-9.80254262541296,-7.41756300748115));
#67325=CARTESIAN_POINT('Ctrl Pts',(36.9776505344837,-9.79622458952494,-7.34689134030989));
#67326=CARTESIAN_POINT('Ctrl Pts',(37.0478831820992,-9.78990655363693,-7.27957713225137));
#67327=CARTESIAN_POINT('Ctrl Pts',(37.1181569837697,-9.78358481558467,-7.21222348024881));
#67328=CARTESIAN_POINT('Ctrl Pts',(37.1915335115763,-9.77726307753242,-7.14823149221863));
#67329=CARTESIAN_POINT('Ctrl Pts',(37.267647957252,-9.77094133948016,-7.08788157124288));
#67330=CARTESIAN_POINT('Ctrl Pts',(37.3438844459462,-9.76460946506039,-7.02743488431868));
#67331=CARTESIAN_POINT('Ctrl Pts',(37.4228672637757,-9.75827759064061,-6.97064218053304));
#67332=CARTESIAN_POINT('Ctrl Pts',(37.50420242666,-9.75194571622084,-6.91774066438448));
#67333=CARTESIAN_POINT('Ctrl Pts',(37.5514422323692,-9.74826813684732,-6.88701524064454));
#67334=CARTESIAN_POINT('Ctrl Pts',(37.5994750806433,-9.74459055747381,-6.85760159529307));
#67335=CARTESIAN_POINT('Ctrl Pts',(37.6482203312017,-9.7409129781003,-6.8295389054182));
#67336=CARTESIAN_POINT('Ctrl Pts',(37.7321573860576,-9.73458035742289,-6.78121625834086));
#67337=CARTESIAN_POINT('Ctrl Pts',(37.8184995468397,-9.72824773674547,-6.73673412833242));
#67338=CARTESIAN_POINT('Ctrl Pts',(37.9068606253913,-9.72191511606806,-6.69633932562838));
#67339=CARTESIAN_POINT('Ctrl Pts',(37.9951027844579,-9.71559101805699,-6.65599888768778));
#67340=CARTESIAN_POINT('Ctrl Pts',(38.0853580665042,-9.70926692004591,-6.61973502410073));
#67341=CARTESIAN_POINT('Ctrl Pts',(38.1772139628289,-9.70294282203483,-6.58774969145156));
#67342=CARTESIAN_POINT('Ctrl Pts',(38.2689737138614,-9.69662534343825,-6.55579783775452));
#67343=CARTESIAN_POINT('Ctrl Pts',(38.3623303376579,-9.69030786484167,-6.52811575492159));
#67344=CARTESIAN_POINT('Ctrl Pts',(38.4568504540997,-9.68399038624509,-6.50485771770135));
#67345=CARTESIAN_POINT('Ctrl Pts',(38.5513034776338,-9.67767739196384,-6.48161618965821));
#67346=CARTESIAN_POINT('Ctrl Pts',(38.6469179284761,-9.67136439768259,-6.4627925683058));
#67347=CARTESIAN_POINT('Ctrl Pts',(38.7432452533336,-9.66505140340134,-6.44849130436827));
#67348=CARTESIAN_POINT('Ctrl Pts',(38.8395377687616,-9.6587406904222,-6.43419520842267));
#67349=CARTESIAN_POINT('Ctrl Pts',(38.9365422142011,-9.65242997744306,-6.42441828682276));
#67350=CARTESIAN_POINT('Ctrl Pts',(39.0338007587653,-9.64611926446391,-6.41921371226013));
#67351=CARTESIAN_POINT('Ctrl Pts',(39.1310504999795,-9.63980912269849,-6.41400960878917));
#67352=CARTESIAN_POINT('Ctrl Pts',(39.2285538578922,-9.63349898093307,-6.41337705265527));
#67353=CARTESIAN_POINT('Ctrl Pts',(39.3258498582418,-9.62718883916764,-6.41731718702173));
#67354=CARTESIAN_POINT('Ctrl Pts',(39.4231634041853,-9.62087755948098,-6.42125803192098));
#67355=CARTESIAN_POINT('Ctrl Pts',(39.5202690813507,-9.61456627979432,-6.42977318735595));
#67356=CARTESIAN_POINT('Ctrl Pts',(39.6167089523252,-9.60825500010766,-6.44281176727443));
#67357=CARTESIAN_POINT('Ctrl Pts',(39.71325195973,-9.6019369709008,-6.45586429114134));
#67358=CARTESIAN_POINT('Ctrl Pts',(39.8091273053147,-9.59561894169395,-6.47344983864871));
#67359=CARTESIAN_POINT('Ctrl Pts',(39.9038853932927,-9.58930091248709,-6.49546604144974));
#67360=CARTESIAN_POINT('Ctrl Pts',(39.9986990067124,-9.58297918110165,-6.51749514509557));
#67361=CARTESIAN_POINT('Ctrl Pts',(40.0923936382179,-9.57665744971622,-6.54395995502503));
#67362=CARTESIAN_POINT('Ctrl Pts',(40.1845350731388,-9.57033571833079,-6.57470826143251));
#67363=CARTESIAN_POINT('Ctrl Pts',(40.276824250434,-9.56400385048931,-6.60550587060807));
#67364=CARTESIAN_POINT('Ctrl Pts',(40.3675548505607,-9.55767198264784,-6.64060053336553));
#67365=CARTESIAN_POINT('Ctrl Pts',(40.4563128844983,-9.55134011480636,-6.67979199545207));
#67366=CARTESIAN_POINT('Ctrl Pts',(40.5078649133095,-9.547662468751,-6.70255499833763));
#67367=CARTESIAN_POINT('Ctrl Pts',(40.5587519517666,-9.54398482269563,-6.72669917366006));
#67368=CARTESIAN_POINT('Ctrl Pts',(40.6088971099685,-9.54030717664027,-6.75217840703331));
#67369=CARTESIAN_POINT('Ctrl Pts',(40.695243138506,-9.53397455864416,-6.79605164805693));
#67370=CARTESIAN_POINT('Ctrl Pts',(40.7796878691838,-9.52764194064806,-6.84403817627217));
#67371=CARTESIAN_POINT('Ctrl Pts',(40.8618135300702,-9.52130932265195,-6.89594951661712));
#67372=CARTESIAN_POINT('Ctrl Pts',(40.943828662441,-9.51498522738624,-6.94779099227758));
#67373=CARTESIAN_POINT('Ctrl Pts',(41.0235305618395,-9.50866113212053,-7.00354654977566));
#67374=CARTESIAN_POINT('Ctrl Pts',(41.1005246285842,-9.50233703685482,-7.06298115583068));
#67375=CARTESIAN_POINT('Ctrl Pts',(41.1774381051049,-9.49601956106352,-7.12235355127105));
#67376=CARTESIAN_POINT('Ctrl Pts',(41.2516490393578,-9.48970208527221,-7.18539707370326));
#67377=CARTESIAN_POINT('Ctrl Pts',(41.3227913507861,-9.48338460948091,-7.25183314868272));
#67378=CARTESIAN_POINT('Ctrl Pts',(41.3938831625975,-9.47707161808294,-7.31822206471739));
#67379=CARTESIAN_POINT('Ctrl Pts',(41.4619103633229,-9.47075862668498,-7.3879984480901));
#67380=CARTESIAN_POINT('Ctrl Pts',(41.5265403001393,-9.46444563528701,-7.46084378383622));
#67381=CARTESIAN_POINT('Ctrl Pts',(41.5911468813939,-9.45813492523835,-7.53366279519109));
#67382=CARTESIAN_POINT('Ctrl Pts',(41.6523583482207,-9.45182421518967,-7.60954822845637));
#67383=CARTESIAN_POINT('Ctrl Pts',(41.7098799157295,-9.44551350514101,-7.68814577020454));
#67384=CARTESIAN_POINT('Ctrl Pts',(41.7673962762773,-9.43920336634975,-7.76673619715462));
#67385=CARTESIAN_POINT('Ctrl Pts',(41.821223143508,-9.43289322755849,-7.84803789144386));
#67386=CARTESIAN_POINT('Ctrl Pts',(41.8711075828414,-9.42658308876723,-7.93166546708255));
#67387=CARTESIAN_POINT('Ctrl Pts',(41.9210010176277,-9.42027181209495,-8.0153081229332));
#67388=CARTESIAN_POINT('Ctrl Pts',(41.9669503885398,-9.41396053542268,-8.10127711756356));
#67389=CARTESIAN_POINT('Ctrl Pts',(42.0087479892801,-9.4076492587504,-8.18916116779949));
#67390=CARTESIAN_POINT('Ctrl Pts',(42.0505902896826,-9.40133123260137,-8.27713920398867));
#67391=CARTESIAN_POINT('Ctrl Pts',(42.088271767496,-9.39501320645234,-8.36703598896984));
#67392=CARTESIAN_POINT('Ctrl Pts',(42.1216323864224,-9.38869518030331,-8.45841908346919));
#67393=CARTESIAN_POINT('Ctrl Pts',(42.1550125535429,-9.38237345200471,-8.54985572537026));
#67394=CARTESIAN_POINT('Ctrl Pts',(42.1840666896732,-9.37605172370611,-8.64277999384018));
#67395=CARTESIAN_POINT('Ctrl Pts',(42.2086849024328,-9.36972999540751,-8.73674508515785));
#67396=CARTESIAN_POINT('Ctrl Pts',(42.2333425887402,-9.3633981306686,-8.83086084279547));
#67397=CARTESIAN_POINT('Ctrl Pts',(42.2535500581075,-9.35706626592969,-8.92602032824715));
#67398=CARTESIAN_POINT('Ctrl Pts',(42.2692487054047,-9.35073440119079,-9.02176741235114));
#67399=CARTESIAN_POINT('Ctrl Pts',(42.2783667978414,-9.34705672585397,-9.07737925882956));
#67400=CARTESIAN_POINT('Ctrl Pts',(42.2859648013331,-9.34337905051714,-9.13318923338017));
#67401=CARTESIAN_POINT('Ctrl Pts',(42.2920393016566,-9.33970137518032,-9.18910774062048));
#67402=CARTESIAN_POINT('Ctrl Pts',(42.3024990367058,-9.33336875396508,-9.28539430559504));
#67403=CARTESIAN_POINT('Ctrl Pts',(42.3084750904721,-9.32703613274984,-9.38233715826476));
#67404=CARTESIAN_POINT('Ctrl Pts',(42.3098969268498,-9.3207035115346,-9.47948343960724));
#67405=CARTESIAN_POINT('Ctrl Pts',(42.3113168496662,-9.31437941300128,-9.57649897779818));
#67406=CARTESIAN_POINT('Ctrl Pts',(42.3081947308959,-9.30805531446795,-9.67371696693394));
#67407=CARTESIAN_POINT('Ctrl Pts',(42.300511687823,-9.30173121593463,-9.77067850246445));
#67408=CARTESIAN_POINT('Ctrl Pts',(42.2928366865873,-9.29541373683206,-9.86753854840454));
#67409=CARTESIAN_POINT('Ctrl Pts',(42.2806102861883,-9.28909625772948,-9.96414224073453));
#67410=CARTESIAN_POINT('Ctrl Pts',(42.2638656535685,-9.28277877862691,-10.060030755923));
#67411=CARTESIAN_POINT('Ctrl Pts',(42.2471329068064,-9.27646578386628,-10.1558512064796));
#67412=CARTESIAN_POINT('Ctrl Pts',(42.2258883789053,-9.27015278910564,-10.2509570595708));
#67413=CARTESIAN_POINT('Ctrl Pts',(42.2002169544868,-9.26383979434501,-10.3448956512325));
#67414=CARTESIAN_POINT('Ctrl Pts',(42.1745548069178,-9.25752908090316,-10.4388002964264));
#67415=CARTESIAN_POINT('Ctrl Pts',(42.1444690567,-9.25121836746131,-10.5315380969185));
#67416=CARTESIAN_POINT('Ctrl Pts',(42.110095264744,-9.24490765401946,-10.622668530575));
#67417=CARTESIAN_POINT('Ctrl Pts',(42.0757245842234,-9.23859751180864,-10.7137907153174));
#67418=CARTESIAN_POINT('Ctrl Pts',(42.0370667882152,-9.23228736959783,-10.8033054134044));
#67419=CARTESIAN_POINT('Ctrl Pts',(41.9943063333778,-9.22597722738702,-10.8907901625597));
#67420=CARTESIAN_POINT('Ctrl Pts',(41.9515381675793,-9.21966594727296,-10.9782906877748));
#67421=CARTESIAN_POINT('Ctrl Pts',(41.9046660656227,-9.21335466715889,-11.0637601441468));
#67422=CARTESIAN_POINT('Ctrl Pts',(41.8539208926113,-9.20704338704483,-11.1467997868606));
#67423=CARTESIAN_POINT('Ctrl Pts',(41.8031214510481,-9.20072535744087,-11.229928234891));
#67424=CARTESIAN_POINT('Ctrl Pts',(41.7484408975837,-9.19440732783692,-11.310621307687));
#67425=CARTESIAN_POINT('Ctrl Pts',(41.6901538703592,-9.18808929823297,-11.3885086141028));
#67426=CARTESIAN_POINT('Ctrl Pts',(41.6318326888123,-9.18176756646698,-11.4664415599737));
#67427=CARTESIAN_POINT('Ctrl Pts',(41.5699011034469,-9.17544583470099,-11.5415651283521));
#67428=CARTESIAN_POINT('Ctrl Pts',(41.5046731905301,-9.169124102935,-11.6135430658121));
#67429=CARTESIAN_POINT('Ctrl Pts',(41.4393406895139,-9.16279223474305,-11.685636414533));
#67430=CARTESIAN_POINT('Ctrl Pts',(41.3707016152595,-9.1564603665511,-11.7545737510813));
#67431=CARTESIAN_POINT('Ctrl Pts',(41.2991058875574,-9.15012849835915,-11.8200566715709));
#67432=CARTESIAN_POINT('Ctrl Pts',(41.2575220429871,-9.14645085681287,-11.8580901084119));
#67433=CARTESIAN_POINT('Ctrl Pts',(41.2149413990742,-9.14277321526659,-11.8949589726356));
#67434=CARTESIAN_POINT('Ctrl Pts',(41.1714371129706,-9.13909557372031,-11.9306114321524));
#67435=CARTESIAN_POINT('Ctrl Pts',(41.0965260282759,-9.13276295360344,-11.9920022663353));
#67436=CARTESIAN_POINT('Ctrl Pts',(41.0186145161548,-9.12643033348657,-12.0499972896543));
#67437=CARTESIAN_POINT('Ctrl Pts',(40.9380432358095,-9.12009771336969,-12.104289895176));
#67438=CARTESIAN_POINT('Ctrl Pts',(40.857580391501,-9.11377361594509,-12.1585094315475));
#67439=CARTESIAN_POINT('Ctrl Pts',(40.7744652532317,-9.10744951852048,-12.2090362114775));
#67440=CARTESIAN_POINT('Ctrl Pts',(40.6890717773488,-9.10112542109588,-12.2556035770143));
#67441=CARTESIAN_POINT('Ctrl Pts',(40.6037676829078,-9.09480794311076,-12.3021222004401));
#67442=CARTESIAN_POINT('Ctrl Pts',(40.5161903737469,-9.08849046512565,-12.3446894403163));
#67443=CARTESIAN_POINT('Ctrl Pts',(40.4267421897094,-9.08217298714054,-12.3830822683903));
#67444=CARTESIAN_POINT('Ctrl Pts',(40.337357498887,-9.07585999350571,-12.4214478439927));
#67445=CARTESIAN_POINT('Ctrl Pts',(40.2461049740665,-9.06954699987087,-12.4556447266813));
#67446=CARTESIAN_POINT('Ctrl Pts',(40.1534100670551,-9.06323400623604,-12.4854965625614));
#67447=CARTESIAN_POINT('Ctrl Pts',(40.0607486571582,-9.05692329392471,-12.5153376108979));
#67448=CARTESIAN_POINT('Ctrl Pts',(39.9666463166037,-9.05061258161338,-12.5408365984476));
#67449=CARTESIAN_POINT('Ctrl Pts',(39.8715460304821,-9.04430186930205,-12.5618662436538));
#67450=CARTESIAN_POINT('Ctrl Pts',(39.7764543526678,-9.03799172822508,-12.5828939852942));
#67451=CARTESIAN_POINT('Ctrl Pts',(39.6803653359286,-9.03168158714811,-12.5994530947248));
#67452=CARTESIAN_POINT('Ctrl Pts',(39.583733569712,-9.02537144607114,-12.6114671066409));
#67453=CARTESIAN_POINT('Ctrl Pts',(39.487084377987,-9.01906016709284,-12.6234832850316));
#67454=CARTESIAN_POINT('Ctrl Pts',(39.3898926763658,-9.01274888811454,-12.6309526841345));
#67455=CARTESIAN_POINT('Ctrl Pts',(39.2926185614714,-9.00643760913624,-12.6338506646301));
#67456=CARTESIAN_POINT('Ctrl Pts',(39.1952404183684,-9.00011958066403,-12.6367517443235));
#67457=CARTESIAN_POINT('Ctrl Pts',(39.0977801238736,-8.99380155219182,-12.6350716320868));
#67458=CARTESIAN_POINT('Ctrl Pts',(39.0006979589456,-8.98748352371961,-12.6288378419839));
#67459=CARTESIAN_POINT('Ctrl Pts',(38.9035589069733,-8.98116179308475,-12.6226003990795));
#67460=CARTESIAN_POINT('Ctrl Pts',(38.8067988602019,-8.9748400624499,-12.6118040134485));
#67461=CARTESIAN_POINT('Ctrl Pts',(38.7108710709203,-8.96851833181504,-12.5965278842357));
#67462=CARTESIAN_POINT('Ctrl Pts',(38.614789468363,-8.96218646474209,-12.581227260854));
#67463=CARTESIAN_POINT('Ctrl Pts',(38.5195432158814,-8.95585459766914,-12.5614326397369));
#67464=CARTESIAN_POINT('Ctrl Pts',(38.425573464008,-8.94952273059619,-12.5372739240068));
#67465=CARTESIAN_POINT('Ctrl Pts',(38.3709942830016,-8.94584507781758,-12.5232421436474));
#67466=CARTESIAN_POINT('Ctrl Pts',(38.3168454266995,-8.94216742503896,-12.5077390755156));
#67467=CARTESIAN_POINT('Ctrl Pts',(38.2632102881944,-8.93848977226034,-12.4907976479786));
#67468=CARTESIAN_POINT('Ctrl Pts',(38.1708549285897,-8.93215715237089,-12.4616258834225));
#67469=CARTESIAN_POINT('Ctrl Pts',(38.0797030675351,-8.92582453248145,-12.428085402372));
#67470=CARTESIAN_POINT('Ctrl Pts',(37.9901976627439,-8.919491912592,-12.3902938693387));
#67471=CARTESIAN_POINT('Ctrl Pts',(37.9008127179915,-8.91316781540169,-12.3525531976979));
#67472=CARTESIAN_POINT('Ctrl Pts',(37.8130702248328,-8.90684371821139,-12.3105730139726));
#67473=CARTESIAN_POINT('Ctrl Pts',(37.7273978892981,-8.90051962102109,-12.264520701958));
#67474=CARTESIAN_POINT('Ctrl Pts',(37.6418152271798,-8.8942021432768,-12.2185165929966));
#67475=CARTESIAN_POINT('Ctrl Pts',(37.5582987980726,-8.88788466553251,-12.1684490353812));
#67476=CARTESIAN_POINT('Ctrl Pts',(37.477255288265,-8.88156718778823,-12.114533029542));
#67477=CARTESIAN_POINT('Ctrl Pts',(37.3962693058775,-8.87525419440299,-12.0606552951046));
#67478=CARTESIAN_POINT('Ctrl Pts',(37.3177531160937,-8.86894120101776,-12.0029347848817));
#67479=CARTESIAN_POINT('Ctrl Pts',(37.242086954399,-8.86262820763253,-11.9416313659235));
#67480=CARTESIAN_POINT('Ctrl Pts',(37.166448136214,-8.85631749557613,-11.8803501002053));
#67481=CARTESIAN_POINT('Ctrl Pts',(37.0936576391097,-8.85000678351973,-11.8154887734607));
#67482=CARTESIAN_POINT('Ctrl Pts',(37.0240641903321,-8.84369607146334,-11.7473487586571));
#67483=CARTESIAN_POINT('Ctrl Pts',(36.9544770410844,-8.83738593064634,-11.6792149118201));
#67484=CARTESIAN_POINT('Ctrl Pts',(36.8880866771076,-8.83107578982933,-11.6078032730928));
#67485=CARTESIAN_POINT('Ctrl Pts',(36.8252056162223,-8.82476564901233,-11.5334527098436));
#67486=CARTESIAN_POINT('Ctrl Pts',(36.7623132161059,-8.81845437029873,-11.459088739088));
#67487=CARTESIAN_POINT('Ctrl Pts',(36.7029316583213,-8.81214309158513,-11.3817851251468));
#67488=CARTESIAN_POINT('Ctrl Pts',(36.647333072897,-8.80583181287153,-11.3019136760615));
#67489=CARTESIAN_POINT('Ctrl Pts',(36.5916750285238,-8.79951378466971,-11.2219568098318));
#67490=CARTESIAN_POINT('Ctrl Pts',(36.5398082836528,-8.79319575646789,-11.1394269854742));
#67491=CARTESIAN_POINT('Ctrl Pts',(36.491961396797,-8.78687772826606,-11.0547246734176));
#67492=CARTESIAN_POINT('Ctrl Pts',(36.4440864732217,-8.7805559979052,-10.9699727285609));
#67493=CARTESIAN_POINT('Ctrl Pts',(36.4002362949917,-8.77423426754433,-10.8830461513752));
#67494=CARTESIAN_POINT('Ctrl Pts',(36.3605922984875,-8.76791253718347,-10.7943677786565));
#67495=CARTESIAN_POINT('Ctrl Pts',(36.3208847357169,-8.76158067038753,-10.7055472166138));
#67496=CARTESIAN_POINT('Ctrl Pts',(36.2853969812979,-8.7552488035916,-10.6149696571239));
#67497=CARTESIAN_POINT('Ctrl Pts',(36.2542613979903,-8.74891693679567,-10.5230755189512));
#67498=CARTESIAN_POINT('Ctrl Pts',(36.2361773245804,-8.7452392814639,-10.4697018492103));
#67499=CARTESIAN_POINT('Ctrl Pts',(36.2195605060004,-8.74156162613213,-10.41588429103));
#67500=CARTESIAN_POINT('Ctrl Pts',(36.2044289529257,-8.73788397080036,-10.3617106756999));
#67501=CARTESIAN_POINT('Ctrl Pts',(36.1717147563767,-8.72993293373437,-10.2445881112859));
#67502=CARTESIAN_POINT('Ctrl Pts',(36.145853683177,-8.72198189666838,-10.1254742577294));
#67503=CARTESIAN_POINT('Ctrl Pts',(36.1270448627367,-8.71403085960239,-10.0050805945535));
#67504=CARTESIAN_POINT('Ctrl Pts',(36.1085403106784,-8.70620844565722,-9.88663452746552));
#67505=CARTESIAN_POINT('Ctrl Pts',(36.0968616954961,-8.69838603171205,-9.76694960462697));
#67506=CARTESIAN_POINT('Ctrl Pts',(36.0921528599655,-8.69056361776688,-9.64672430767749));
#67507=CARTESIAN_POINT('Ctrl Pts',(36.0906010386658,-8.68798570046722,-9.60710343424426));
#67508=CARTESIAN_POINT('Ctrl Pts',(36.0898058059764,-8.68540778316755,-9.56742405163508));
#67509=CARTESIAN_POINT('Ctrl Pts',(36.0897711821211,-8.68282986586788,-9.52771170347425));
#67510=CARTESIAN_POINT('',(36.0898198219825,-7.4128297998923,-9.52336150973275));
#67511=CARTESIAN_POINT('Ctrl Pts',(36.0909909580655,-8.68282984291315,-9.5277102865178));
#67512=CARTESIAN_POINT('Ctrl Pts',(36.097370143227,-8.63431261838889,-8.78059823168395));
#67513=CARTESIAN_POINT('Ctrl Pts',(36.7410355037994,-8.51892679337797,-6.99391762846478));
#67514=CARTESIAN_POINT('Ctrl Pts',(39.7185698196114,-8.33667236788041,-5.89196606192947));
#67515=CARTESIAN_POINT('Ctrl Pts',(42.5256954705718,-8.1360665664204,-7.97335575183573));
#67516=CARTESIAN_POINT('Ctrl Pts',(42.3172061964241,-7.93546076496045,-11.4617177794319));
#67517=CARTESIAN_POINT('Ctrl Pts',(39.2821521939203,-7.73485496350045,-13.193937346696));
#67518=CARTESIAN_POINT('Ctrl Pts',(36.5817564488487,-7.56064465615136,-11.8091234637841));
#67519=CARTESIAN_POINT('Ctrl Pts',(36.0968486952276,-7.45330294928892,-10.1480485640383));
#67520=CARTESIAN_POINT('Ctrl Pts',(36.0938362662056,-7.41282984291315,-9.5233642896731));
#67521=CARTESIAN_POINT('',(36.0897702134563,-6.14282984295053,-9.52384769963274));
#67522=CARTESIAN_POINT('Ctrl Pts',(36.0897704316019,-7.41282979936327,-9.52336147554771));
#67523=CARTESIAN_POINT('Ctrl Pts',(36.0898273887419,-7.4058341701422,-9.41524604241845));
#67524=CARTESIAN_POINT('Ctrl Pts',(36.0955258185163,-7.39883854092113,-9.30732612022363));
#67525=CARTESIAN_POINT('Ctrl Pts',(36.106780042231,-7.39184291170005,-9.2001601228919));
#67526=CARTESIAN_POINT('Ctrl Pts',(36.1180725251958,-7.38482350051631,-9.09262980983287));
#67527=CARTESIAN_POINT('Ctrl Pts',(36.1349585203378,-7.37780408933257,-8.98585880502142));
#67528=CARTESIAN_POINT('Ctrl Pts',(36.1573013842396,-7.37078467814884,-8.88039485997273));
#67529=CARTESIAN_POINT('Ctrl Pts',(36.1797517784313,-7.36373148439706,-8.77442334487207));
#67530=CARTESIAN_POINT('Ctrl Pts',(36.2077115733386,-7.35667829064528,-8.66977174456544));
#67531=CARTESIAN_POINT('Ctrl Pts',(36.2409934482374,-7.3496250968935,-8.56697553291882));
#67532=CARTESIAN_POINT('Ctrl Pts',(36.2661310982796,-7.34429785145583,-8.48933401777315));
#67533=CARTESIAN_POINT('Ctrl Pts',(36.2943038279069,-7.33897060601816,-8.41275055453054));
#67534=CARTESIAN_POINT('Ctrl Pts',(36.325413315959,-7.3336433605805,-8.3374470332511));
#67535=CARTESIAN_POINT('Ctrl Pts',(36.3623938855919,-7.32731074043165,-8.24793199180745));
#67536=CARTESIAN_POINT('Ctrl Pts',(36.4036239373028,-7.3209781202828,-8.15999048092687));
#67537=CARTESIAN_POINT('Ctrl Pts',(36.4489482718138,-7.31464550013395,-8.07405374264119));
#67538=CARTESIAN_POINT('Ctrl Pts',(36.4942116070148,-7.30832140267967,-7.98823266146978));
#67539=CARTESIAN_POINT('Ctrl Pts',(36.5435580708494,-7.30199730522538,-7.90441137383109));
#67540=CARTESIAN_POINT('Ctrl Pts',(36.5967842350216,-7.2956732077711,-7.82300166455189));
#67541=CARTESIAN_POINT('Ctrl Pts',(36.649954687292,-7.28935572975863,-7.74167716693145));
#67542=CARTESIAN_POINT('Ctrl Pts',(36.7069965286074,-7.28303825174617,-7.66275959353606));
#67543=CARTESIAN_POINT('Ctrl Pts',(36.767660690969,-7.2767207737337,-7.58663570538395));
#67544=CARTESIAN_POINT('Ctrl Pts',(36.8282817919105,-7.27040778007515,-7.51056585247427));
#67545=CARTESIAN_POINT('Ctrl Pts',(36.8925198303435,-7.2640947864166,-7.43728608341478));
#67546=CARTESIAN_POINT('Ctrl Pts',(36.9600833039791,-7.25778179275805,-7.36715296005788));
#67547=CARTESIAN_POINT('Ctrl Pts',(37.0276223622105,-7.25147108042526,-7.29704518069929));
#67548=CARTESIAN_POINT('Ctrl Pts',(37.0984841647337,-7.24516036809247,-7.23008210223094));
#67549=CARTESIAN_POINT('Ctrl Pts',(37.1723385567986,-7.23884965575968,-7.16658533657574));
#67550=CARTESIAN_POINT('Ctrl Pts',(37.2461862636697,-7.23253951466354,-7.10309431855691));
#67551=CARTESIAN_POINT('Ctrl Pts',(37.3230256897622,-7.22622937356739,-7.04306927445219));
#67552=CARTESIAN_POINT('Ctrl Pts',(37.402492427576,-7.21991923247124,-6.98679252621495));
#67553=CARTESIAN_POINT('Ctrl Pts',(37.4819734955165,-7.21360795347609,-6.93050562966963));
#67554=CARTESIAN_POINT('Ctrl Pts',(37.5640824592646,-7.20729667448094,-6.8779686241699));
#67555=CARTESIAN_POINT('Ctrl Pts',(37.6484255536837,-7.20098539548579,-6.82942076902972));
#67556=CARTESIAN_POINT('Ctrl Pts',(37.7328588473938,-7.19466736700043,-6.78082099520979));
#67557=CARTESIAN_POINT('Ctrl Pts',(37.8195306621525,-7.18834933851507,-6.73621910736065));
#67558=CARTESIAN_POINT('Ctrl Pts',(37.908022410618,-7.18203131002971,-6.69580849686087));
#67559=CARTESIAN_POINT('Ctrl Pts',(37.9965660123893,-7.17570957938377,-6.65537420704884));
#67560=CARTESIAN_POINT('Ctrl Pts',(38.0869312656922,-7.16938784873782,-6.61913624775709));
#67561=CARTESIAN_POINT('Ctrl Pts',(38.1786813381664,-7.16306611809187,-6.58723914453703));
#67562=CARTESIAN_POINT('Ctrl Pts',(38.2705785252,-7.15673425101123,-6.55529089663493));
#67563=CARTESIAN_POINT('Ctrl Pts',(38.3638645461799,-7.15040238393059,-6.52769752715895));
#67564=CARTESIAN_POINT('Ctrl Pts',(38.4580892577887,-7.14407051684995,-6.50455316161806));
#67565=CARTESIAN_POINT('Ctrl Pts',(38.5128165205381,-7.14039286427346,-6.49111053332556));
#67566=CARTESIAN_POINT('Ctrl Pts',(38.5678602730804,-7.13671521169698,-6.479167805297));
#67567=CARTESIAN_POINT('Ctrl Pts',(38.6231314638014,-7.13303755912049,-6.46873539351645));
#67568=CARTESIAN_POINT('Ctrl Pts',(38.7183039818019,-7.1267049389712,-6.45077162459775));
#67569=CARTESIAN_POINT('Ctrl Pts',(38.8144817016523,-7.1203723188219,-6.43722641490242));
#67570=CARTESIAN_POINT('Ctrl Pts',(38.9112186743944,-7.11403969867261,-6.42820552847279));
#67571=CARTESIAN_POINT('Ctrl Pts',(39.0078254546328,-7.10771560121789,-6.41919678271448));
#67572=CARTESIAN_POINT('Ctrl Pts',(39.1049895600594,-7.10139150376317,-6.41470029827978));
#67573=CARTESIAN_POINT('Ctrl Pts',(39.2022549719265,-7.09506740630845,-6.41477081744743));
#67574=CARTESIAN_POINT('Ctrl Pts',(39.2994185759482,-7.08874992829556,-6.41484126280258));
#67575=CARTESIAN_POINT('Ctrl Pts',(39.3966828405869,-7.08243245028267,-6.41946920799966));
#67576=CARTESIAN_POINT('Ctrl Pts',(39.4935877540451,-7.07611497226978,-6.42865749898775));
#67577=CARTESIAN_POINT('Ctrl Pts',(39.5904238812048,-7.0698019786108,-6.43783926782436));
#67578=CARTESIAN_POINT('Ctrl Pts',(39.6869007301712,-7.06348898495182,-6.45157490577345));
#67579=CARTESIAN_POINT('Ctrl Pts',(39.7825603819843,-7.05717599129284,-6.46981521765995));
#67580=CARTESIAN_POINT('Ctrl Pts',(39.8781854652806,-7.05086527895962,-6.48804893804712));
#67581=CARTESIAN_POINT('Ctrl Pts',(39.9729935090707,-7.0445545666264,-6.51078401598165));
#67582=CARTESIAN_POINT('Ctrl Pts',(40.0665347326534,-7.03824385429318,-6.53791978514046));
#67583=CARTESIAN_POINT('Ctrl Pts',(40.1600674890183,-7.03193371319662,-6.56505309800825));
#67584=CARTESIAN_POINT('Ctrl Pts',(40.2523332332299,-7.02562357210006,-6.5965861880615));
#67585=CARTESIAN_POINT('Ctrl Pts',(40.3428963620796,-7.0193134310035,-6.63236822971793));
#67586=CARTESIAN_POINT('Ctrl Pts',(40.4334758220529,-7.01300215200794,-6.66815672390034));
#67587=CARTESIAN_POINT('Ctrl Pts',(40.5223516501643,-7.00669087301236,-6.7081955307434));
#67588=CARTESIAN_POINT('Ctrl Pts',(40.6091082556239,-7.0003795940168,-6.75228570227067));
#67589=CARTESIAN_POINT('Ctrl Pts',(40.6959576414627,-6.99406156553103,-6.79642302528356));
#67590=CARTESIAN_POINT('Ctrl Pts',(40.7806828894738,-6.98774353704526,-6.8446201644518));
#67591=CARTESIAN_POINT('Ctrl Pts',(40.8628932495411,-6.98142550855949,-6.89663231386275));
#67592=CARTESIAN_POINT('Ctrl Pts',(40.9451517822235,-6.97510377791315,-6.94867494071292));
#67593=CARTESIAN_POINT('Ctrl Pts',(41.0248921345258,-6.9687820472668,-7.00453677843929));
#67594=CARTESIAN_POINT('Ctrl Pts',(41.1017545025994,-6.96246031662045,-7.06393103210355));
#67595=CARTESIAN_POINT('Ctrl Pts',(41.1787401138824,-6.95612844953942,-7.12342052012791));
#67596=CARTESIAN_POINT('Ctrl Pts',(41.2528381934284,-6.94979658245839,-7.18645345087234));
#67597=CARTESIAN_POINT('Ctrl Pts',(41.3237238654314,-6.94346471537735,-7.25270433343348));
#67598=CARTESIAN_POINT('Ctrl Pts',(41.3648954299389,-6.93978706280508,-7.29118393598174));
#67599=CARTESIAN_POINT('Ctrl Pts',(41.4049840050208,-6.9361094102328,-7.33074843506157));
#67600=CARTESIAN_POINT('Ctrl Pts',(41.4439321912292,-6.93243175766053,-7.37132895407274));
#67601=CARTESIAN_POINT('Ctrl Pts',(41.5109978163644,-6.92609913751051,-7.44120532421315));
#67602=CARTESIAN_POINT('Ctrl Pts',(41.574912884085,-6.9197665173605,-7.51433869978135));
#67603=CARTESIAN_POINT('Ctrl Pts',(41.6353450654081,-6.91343389721048,-7.59041346399488));
#67604=CARTESIAN_POINT('Ctrl Pts',(41.6956959146744,-6.90710979975502,-7.6663858437351));
#67605=CARTESIAN_POINT('Ctrl Pts',(41.7525729242711,-6.90078570229956,-7.74529140461175));
#67606=CARTESIAN_POINT('Ctrl Pts',(41.8056809855595,-6.8944616048441,-7.82677820812661));
#67607=CARTESIAN_POINT('Ctrl Pts',(41.8587334585644,-6.88814412683046,-7.9081797192881));
#67608=CARTESIAN_POINT('Ctrl Pts',(41.9080245885148,-6.88182664881682,-7.99215673735205));
#67609=CARTESIAN_POINT('Ctrl Pts',(41.9533005411212,-6.87550917080318,-8.07832561259919));
#67610=CARTESIAN_POINT('Ctrl Pts',(41.9985443553659,-6.86919617714343,-8.16443332234162));
#67611=CARTESIAN_POINT('Ctrl Pts',(42.0397784556136,-6.86288318348368,-8.25272941011052));
#67612=CARTESIAN_POINT('Ctrl Pts',(42.0767937298344,-6.85657018982393,-8.34280353202805));
#67613=CARTESIAN_POINT('Ctrl Pts',(42.1137956278501,-6.85025947748994,-8.43284510387106));
#67614=CARTESIAN_POINT('Ctrl Pts',(42.1465815630955,-6.84394876515594,-8.5246630290721));
#67615=CARTESIAN_POINT('Ctrl Pts',(42.1749899730535,-6.83763805282195,-8.6178256434779));
#67616=CARTESIAN_POINT('Ctrl Pts',(42.2033958115229,-6.8313279117246,-8.71097982493722));
#67617=CARTESIAN_POINT('Ctrl Pts',(42.227424785183,-6.82501777062725,-8.80547803523857));
#67618=CARTESIAN_POINT('Ctrl Pts',(42.2469650836379,-6.8187076295299,-8.90087306419978));
#67619=CARTESIAN_POINT('Ctrl Pts',(42.2665089057679,-6.81239635053354,-8.9962852956145));
#67620=CARTESIAN_POINT('Ctrl Pts',(42.2815623573302,-6.80608507153719,-9.09259423847046));
#67621=CARTESIAN_POINT('Ctrl Pts',(42.292064863898,-6.79977379254083,-9.18934313600433));
#67622=CARTESIAN_POINT('Ctrl Pts',(42.3025786021932,-6.79345576405426,-9.28619550000468));
#67623=CARTESIAN_POINT('Ctrl Pts',(42.3085316316604,-6.7871377355677,-9.38348832253946));
#67624=CARTESIAN_POINT('Ctrl Pts',(42.3099153568417,-6.78081970708113,-9.48076058115117));
#67625=CARTESIAN_POINT('Ctrl Pts',(42.3112998928413,-6.77449797643398,-9.578089838164));
#67626=CARTESIAN_POINT('Ctrl Pts',(42.3081098073144,-6.76817624578682,-9.67539807037417));
#67627=CARTESIAN_POINT('Ctrl Pts',(42.3003885814515,-6.76185451513967,-9.77222721716105));
#67628=CARTESIAN_POINT('Ctrl Pts',(42.2926549751652,-6.75552264805783,-9.86921162243274));
#67629=CARTESIAN_POINT('Ctrl Pts',(42.280375776071,-6.74919078097599,-9.96571497482189));
#67630=CARTESIAN_POINT('Ctrl Pts',(42.2636459609728,-6.74285891389416,-10.0612873098584));
#67631=CARTESIAN_POINT('Ctrl Pts',(42.2539290091472,-6.73918126132962,-10.1167972942758));
#67632=CARTESIAN_POINT('Ctrl Pts',(42.2427116025523,-6.73550360876508,-10.1719934283378));
#67633=CARTESIAN_POINT('Ctrl Pts',(42.2300200415556,-6.73182595620054,-10.2267899975574));
#67634=CARTESIAN_POINT('Ctrl Pts',(42.2081662004202,-6.72549333605104,-10.3211452560473));
#67635=CARTESIAN_POINT('Ctrl Pts',(42.1818628489603,-6.71916071590154,-10.4146426367809));
#67636=CARTESIAN_POINT('Ctrl Pts',(42.1511926215263,-6.71282809575204,-10.506831331517));
#67637=CARTESIAN_POINT('Ctrl Pts',(42.1205636713164,-6.70650399829711,-10.5988959550047));
#67638=CARTESIAN_POINT('Ctrl Pts',(42.0855796630611,-6.70017990084217,-10.6896549816782));
#67639=CARTESIAN_POINT('Ctrl Pts',(42.0463739915869,-6.69385580338724,-10.778668916787));
#67640=CARTESIAN_POINT('Ctrl Pts',(42.0072093567449,-6.68753832537413,-10.8675896808831));
#67641=CARTESIAN_POINT('Ctrl Pts',(41.9638320188586,-6.68122084736102,-10.9547685866518));
#67642=CARTESIAN_POINT('Ctrl Pts',(41.9164244884842,-6.67490336934791,-11.039783367767));
#67643=CARTESIAN_POINT('Ctrl Pts',(41.8690506095358,-6.6685903756887,-11.1247378025913));
#67644=CARTESIAN_POINT('Ctrl Pts',(41.8176524378495,-6.66227738202948,-11.2075307858949));
#67645=CARTESIAN_POINT('Ctrl Pts',(41.7624592832083,-6.65596438837028,-11.2877629094123));
#67646=CARTESIAN_POINT('Ctrl Pts',(41.7072860737107,-6.64965367603682,-11.3679660394569));
#67647=CARTESIAN_POINT('Ctrl Pts',(41.6483208538315,-6.64334296370337,-11.4456097886015));
#67648=CARTESIAN_POINT('Ctrl Pts',(41.5858367780203,-6.63703225136992,-11.5203229115974));
#67649=CARTESIAN_POINT('Ctrl Pts',(41.5233583581783,-6.63072211027312,-11.5950292716684));
#67650=CARTESIAN_POINT('Ctrl Pts',(41.4573619964096,-6.62441196917632,-11.6668051976961));
#67651=CARTESIAN_POINT('Ctrl Pts',(41.3881610605712,-6.61810182807952,-11.7353126081846));
#67652=CARTESIAN_POINT('Ctrl Pts',(41.3189476458239,-6.61179054908371,-11.8038323725195));
#67653=CARTESIAN_POINT('Ctrl Pts',(41.2465288200725,-6.6054792700879,-11.8690821430423));
#67654=CARTESIAN_POINT('Ctrl Pts',(41.1712539518533,-6.5991679910921,-11.9307615239676));
#67655=CARTESIAN_POINT('Ctrl Pts',(41.0958985822038,-6.59284996260608,-11.9925068668601));
#67656=CARTESIAN_POINT('Ctrl Pts',(41.0176814110704,-6.58653193412006,-12.050673919519));
#67657=CARTESIAN_POINT('Ctrl Pts',(40.9369837916899,-6.58021390563404,-12.1050034806772));
#67658=CARTESIAN_POINT('Ctrl Pts',(40.8562388861115,-6.57389217498744,-12.1593648772031));
#67659=CARTESIAN_POINT('Ctrl Pts',(40.7730110117137,-6.56757044434084,-12.2098840777438));
#67660=CARTESIAN_POINT('Ctrl Pts',(40.6877075076263,-6.56124871369424,-12.2563471080498));
#67661=CARTESIAN_POINT('Ctrl Pts',(40.6022672255828,-6.55491684661295,-12.3028846384411));
#67662=CARTESIAN_POINT('Ctrl Pts',(40.5147450613693,-6.54858497953166,-12.3453528209146));
#67663=CARTESIAN_POINT('Ctrl Pts',(40.4255697230247,-6.54225311245038,-12.3835852282039));
#67664=CARTESIAN_POINT('Ctrl Pts',(40.3737752194401,-6.53857545988044,-12.4057912393404));
#67665=CARTESIAN_POINT('Ctrl Pts',(40.3214233513951,-6.53489780731049,-12.4265692408719));
#67666=CARTESIAN_POINT('Ctrl Pts',(40.2686002708934,-6.53122015474055,-12.4458944030804));
#67667=CARTESIAN_POINT('Ctrl Pts',(40.1776432004288,-6.52488753459096,-12.4791707687154));
#67668=CARTESIAN_POINT('Ctrl Pts',(40.0849723144736,-6.51855491444136,-12.5082522645267));
#67669=CARTESIAN_POINT('Ctrl Pts',(39.9910102810063,-6.51222229429177,-12.5329616666843));
#67670=CARTESIAN_POINT('Ctrl Pts',(39.8971747054179,-6.50589819683673,-12.557637813936));
#67671=CARTESIAN_POINT('Ctrl Pts',(39.8020518553959,-6.4995740993817,-12.5779534522547));
#67672=CARTESIAN_POINT('Ctrl Pts',(39.7060826718468,-6.49325000192667,-12.5937800478621));
#67673=CARTESIAN_POINT('Ctrl Pts',(39.6102139393791,-6.48693252391347,-12.6095900777492));
#67674=CARTESIAN_POINT('Ctrl Pts',(39.513501063732,-6.48061504590026,-12.620920335358));
#67675=CARTESIAN_POINT('Ctrl Pts',(39.4163974066349,-6.47429756788705,-12.6276928328956));
#67676=CARTESIAN_POINT('Ctrl Pts',(39.3193626769108,-6.46798457422775,-12.6344605230914));
#67677=CARTESIAN_POINT('Ctrl Pts',(39.2219381522197,-6.46167158056845,-12.6366768547426));
#67678=CARTESIAN_POINT('Ctrl Pts',(39.1245836347157,-6.45535858690914,-12.6343155235111));
#67679=CARTESIAN_POINT('Ctrl Pts',(39.0272642982019,-6.44904787457559,-12.6319550455936));
#67680=CARTESIAN_POINT('Ctrl Pts',(38.9300153553479,-6.44273716224204,-12.6250202023584));
#67681=CARTESIAN_POINT('Ctrl Pts',(38.8332969914423,-6.4364264499085,-12.6135367986175));
#67682=CARTESIAN_POINT('Ctrl Pts',(38.7365873823446,-6.4301163088116,-12.602054434338));
#67683=CARTESIAN_POINT('Ctrl Pts',(38.6404086909423,-6.4238061677147,-12.5860243799323));
#67684=CARTESIAN_POINT('Ctrl Pts',(38.5452153132195,-6.4174960266178,-12.5655242421099));
#67685=CARTESIAN_POINT('Ctrl Pts',(38.4500047694067,-6.4111847476219,-12.5450204075259));
#67686=CARTESIAN_POINT('Ctrl Pts',(38.3557803196677,-6.404873468626,-12.52004498064));
#67687=CARTESIAN_POINT('Ctrl Pts',(38.2629844813214,-6.39856218963009,-12.490726314186));
#67688=CARTESIAN_POINT('Ctrl Pts',(38.1700894040406,-6.39224416114398,-12.4613762933818));
#67689=CARTESIAN_POINT('Ctrl Pts',(38.0786264060121,-6.38592613265787,-12.4276738918791));
#67690=CARTESIAN_POINT('Ctrl Pts',(37.9890209924694,-6.37960810417175,-12.3897967635105));
#67691=CARTESIAN_POINT('Ctrl Pts',(37.8993630730492,-6.37328637352506,-12.3518974403684));
#67692=CARTESIAN_POINT('Ctrl Pts',(37.8115652997706,-6.36696464287836,-12.3098187081198));
#67693=CARTESIAN_POINT('Ctrl Pts',(37.7260295099797,-6.36064291223166,-12.2637847026463));
#67694=CARTESIAN_POINT('Ctrl Pts',(37.6403565697794,-6.35431104515028,-12.2176768849977));
#67695=CARTESIAN_POINT('Ctrl Pts',(37.5569532300908,-6.3479791780689,-12.1676013552421));
#67696=CARTESIAN_POINT('Ctrl Pts',(37.4761931939458,-6.34164731098752,-12.1138261332699));
#67697=CARTESIAN_POINT('Ctrl Pts',(37.4292864363366,-6.33796965841854,-12.0825925996705));
#67698=CARTESIAN_POINT('Ctrl Pts',(37.3832708016008,-6.33429200584956,-12.0501117623405));
#67699=CARTESIAN_POINT('Ctrl Pts',(37.3382141739985,-6.33061435328058,-12.016442190981));
#67700=CARTESIAN_POINT('Ctrl Pts',(37.2613403634718,-6.32433968999983,-11.9589965190133));
#67701=CARTESIAN_POINT('Ctrl Pts',(37.1869821423794,-6.31806502671907,-11.8978805724172));
#67702=CARTESIAN_POINT('Ctrl Pts',(37.115515165223,-6.31179036343831,-11.8333443474674));
#67703=CARTESIAN_POINT('Ctrl Pts',(37.0441447272916,-6.30552417611602,-11.7688952995242));
#67704=CARTESIAN_POINT('Ctrl Pts',(36.975658102416,-6.29925798879374,-11.7010354484271));
#67705=CARTESIAN_POINT('Ctrl Pts',(36.9104005139929,-6.29299180147145,-11.6300569699122));
#67706=CARTESIAN_POINT('Ctrl Pts',(36.8452155369337,-6.28673258646332,-11.5591574683294));
#67707=CARTESIAN_POINT('Ctrl Pts',(36.783252753632,-6.2804733714552,-11.4851465648293));
#67708=CARTESIAN_POINT('Ctrl Pts',(36.7248220139306,-6.27421415644708,-11.4083546108414));
#67709=CARTESIAN_POINT('Ctrl Pts',(36.6664270297752,-6.2679587716429,-11.3316096481846));
#67710=CARTESIAN_POINT('Ctrl Pts',(36.6115600668311,-6.26170338683871,-11.2520873684212));
#67711=CARTESIAN_POINT('Ctrl Pts',(36.5604914148224,-6.25544800203453,-11.1701519934868));
#67712=CARTESIAN_POINT('Ctrl Pts',(36.5094395360291,-6.24919467177677,-11.0882435297717));
#67713=CARTESIAN_POINT('Ctrl Pts',(36.4621837258304,-6.24294134151901,-11.0039239236958));
#67714=CARTESIAN_POINT('Ctrl Pts',(36.4189508886379,-6.23668801126125,-10.917586260557));
#67715=CARTESIAN_POINT('Ctrl Pts',(36.3757199953772,-6.23043496217974,-10.8312524795257));
#67716=CARTESIAN_POINT('Ctrl Pts',(36.3365119143669,-6.22418191309823,-10.7429012213437));
#67717=CARTESIAN_POINT('Ctrl Pts',(36.3015069900995,-6.21792886401671,-10.6529489901842));
#67718=CARTESIAN_POINT('Ctrl Pts',(36.2664716805982,-6.21167038711718,-10.5629186780223));
#67719=CARTESIAN_POINT('Ctrl Pts',(36.2356469794486,-6.20541191021766,-10.4712850331532));
#67720=CARTESIAN_POINT('Ctrl Pts',(36.2091644294996,-6.19915343331813,-10.3784830069365));
#67721=CARTESIAN_POINT('Ctrl Pts',(36.1826710455795,-6.1928923960852,-10.2856430155517));
#67722=CARTESIAN_POINT('Ctrl Pts',(36.1605234540233,-6.18663135885228,-10.1916341254886));
#67723=CARTESIAN_POINT('Ctrl Pts',(36.142802276078,-6.18037032161936,-10.096902727521));
#67724=CARTESIAN_POINT('Ctrl Pts',(36.1250519834966,-6.17409899794718,-10.0020156925982));
#67725=CARTESIAN_POINT('Ctrl Pts',(36.1117426976542,-6.167827674275,-9.90640422079789));
#67726=CARTESIAN_POINT('Ctrl Pts',(36.1029032457584,-6.16155635060282,-9.81052118619469));
#67727=CARTESIAN_POINT('Ctrl Pts',(36.094104887165,-6.15531418138539,-9.71508389761573));
#67728=CARTESIAN_POINT('Ctrl Pts',(36.0897348207007,-6.14907201216796,-9.61937800194409));
#67729=CARTESIAN_POINT('Ctrl Pts',(36.0897702134563,-6.14282984295053,-9.52384769963273));
#67730=CARTESIAN_POINT('',(36.0897712021404,-4.87282984294947,-9.52773456847233));
#67731=CARTESIAN_POINT('Ctrl Pts',(36.0897702134565,-6.14282984291314,-9.52384769906051));
#67732=CARTESIAN_POINT('Ctrl Pts',(36.0897944454732,-6.13855607921562,-9.458441920427));
#67733=CARTESIAN_POINT('Ctrl Pts',(36.0918816780826,-6.13428231551811,-9.39307717011422));
#67734=CARTESIAN_POINT('Ctrl Pts',(36.096025077601,-6.1300085518206,-9.32784439135976));
#67735=CARTESIAN_POINT('Ctrl Pts',(36.1021645315192,-6.12367593167103,-9.23118616727646));
#67736=CARTESIAN_POINT('Ctrl Pts',(36.1128338748575,-6.11734331152145,-9.13464709945906));
#67737=CARTESIAN_POINT('Ctrl Pts',(36.1280252602644,-6.11101069137187,-9.03868543993983));
#67738=CARTESIAN_POINT('Ctrl Pts',(36.1431962004947,-6.10468659391685,-8.94285292947643));
#67739=CARTESIAN_POINT('Ctrl Pts',(36.1628770188918,-6.09836249646183,-8.84759671107667));
#67740=CARTESIAN_POINT('Ctrl Pts',(36.18700794114,-6.0920383990068,-8.75337217122086));
#67741=CARTESIAN_POINT('Ctrl Pts',(36.2111136055174,-6.0857209209936,-8.65924625632523));
#67742=CARTESIAN_POINT('Ctrl Pts',(36.2396600056321,-6.07940344298039,-8.56615029457657));
#67743=CARTESIAN_POINT('Ctrl Pts',(36.2725360961542,-6.07308596496719,-8.47453070269516));
#67744=CARTESIAN_POINT('Ctrl Pts',(36.3053888501448,-6.06677297130788,-8.38297614541677));
#67745=CARTESIAN_POINT('Ctrl Pts',(36.3425650372436,-6.06045997764858,-8.29289628501466));
#67746=CARTESIAN_POINT('Ctrl Pts',(36.3839037064072,-6.05414698398928,-8.20472263591588));
#67747=CARTESIAN_POINT('Ctrl Pts',(36.425227437021,-6.04783627165573,-8.11658085011804));
#67748=CARTESIAN_POINT('Ctrl Pts',(36.4707104753977,-6.04152555932218,-8.03034430243137));
#67749=CARTESIAN_POINT('Ctrl Pts',(36.5201440126228,-6.03521484698863,-7.9464238884937));
#67750=CARTESIAN_POINT('Ctrl Pts',(36.5695730751947,-6.02890470589173,-7.86251107091183));
#67751=CARTESIAN_POINT('Ctrl Pts',(36.6229517035027,-6.02259456479483,-7.78091434693321));
#67752=CARTESIAN_POINT('Ctrl Pts',(36.680025995923,-6.01628442369793,-7.70201846644678));
#67753=CARTESIAN_POINT('Ctrl Pts',(36.7371105804714,-6.00997314470202,-7.62310835877551));
#67754=CARTESIAN_POINT('Ctrl Pts',(36.7978918964089,-6.00366186570612,-7.5469004162128));
#67755=CARTESIAN_POINT('Ctrl Pts',(36.8620743664621,-5.99735058671021,-7.4737480932498));
#67756=CARTESIAN_POINT('Ctrl Pts',(36.9263254753686,-5.99103255822409,-7.40051753877649));
#67757=CARTESIAN_POINT('Ctrl Pts',(36.9939847111832,-5.98471452973798,-7.3303494571126));
#67758=CARTESIAN_POINT('Ctrl Pts',(37.0647182095184,-5.97839650125186,-7.26356188938593));
#67759=CARTESIAN_POINT('Ctrl Pts',(37.1354931553986,-5.97207477060516,-7.19673518630221));
#67760=CARTESIAN_POINT('Ctrl Pts',(37.2093456193398,-5.96575303995846,-7.13329322644822));
#67761=CARTESIAN_POINT('Ctrl Pts',(37.2859087089586,-5.95943130931176,-7.07351367891653));
#67762=CARTESIAN_POINT('Ctrl Pts',(37.3625945619155,-5.95309944223037,-7.01363827923407));
#67763=CARTESIAN_POINT('Ctrl Pts',(37.4419993626041,-5.94676757514898,-6.95743727053224));
#67764=CARTESIAN_POINT('Ctrl Pts',(37.5237273663984,-5.9404357080676,-6.90514490653809));
#67765=CARTESIAN_POINT('Ctrl Pts',(37.571196335543,-5.93675805549859,-6.87477264124715));
#67766=CARTESIAN_POINT('Ctrl Pts',(37.6194485560584,-5.93308040292958,-6.84571809514552));
#67767=CARTESIAN_POINT('Ctrl Pts',(37.6684030922134,-5.92940275036057,-6.81801984400356));
#67768=CARTESIAN_POINT('Ctrl Pts',(37.7526988423567,-5.92307013021093,-6.77032569671804));
#67769=CARTESIAN_POINT('Ctrl Pts',(37.8393709364328,-5.91673751006129,-6.72648992809303));
#67770=CARTESIAN_POINT('Ctrl Pts',(37.9280313531574,-5.91040488991165,-6.68675645612477));
#67771=CARTESIAN_POINT('Ctrl Pts',(38.0165724471319,-5.90408079245658,-6.64707645905908));
#67772=CARTESIAN_POINT('Ctrl Pts',(38.1070961494503,-5.8977566950015,-6.61148796266889));
#67773=CARTESIAN_POINT('Ctrl Pts',(38.1991884541281,-5.89143259754643,-6.58018983590632));
#67774=CARTESIAN_POINT('Ctrl Pts',(38.2911843656593,-5.88511511953318,-6.54892446893764));
#67775=CARTESIAN_POINT('Ctrl Pts',(38.3847452035775,-5.87879764151992,-6.52194068377684));
#67776=CARTESIAN_POINT('Ctrl Pts',(38.4794364473037,-5.87248016350667,-6.499389512937));
#67777=CARTESIAN_POINT('Ctrl Pts',(38.5740604760673,-5.86616716984732,-6.47685434966073));
#67778=CARTESIAN_POINT('Ctrl Pts',(38.6698128912126,-5.85985417618798,-6.45874564647037));
#67779=CARTESIAN_POINT('Ctrl Pts',(38.7662443716592,-5.85354118252863,-6.44516449988272));
#67780=CARTESIAN_POINT('Ctrl Pts',(38.8626410046733,-5.84723047019504,-6.43158826111238));
#67781=CARTESIAN_POINT('Ctrl Pts',(38.9597157827883,-5.84091975786145,-6.42253638887785));
#67782=CARTESIAN_POINT('Ctrl Pts',(39.0570104906991,-5.83460904552786,-6.41805863377986));
#67783=CARTESIAN_POINT('Ctrl Pts',(39.1542963916323,-5.82829890443091,-6.41358128400185));
#67784=CARTESIAN_POINT('Ctrl Pts',(39.2518017459218,-5.82198876333397,-6.41367724804504));
#67785=CARTESIAN_POINT('Ctrl Pts',(39.349065583702,-5.81567862223703,-6.41834422494935));
#67786=CARTESIAN_POINT('Ctrl Pts',(39.4463469609353,-5.80936734324108,-6.42301204344313));
#67787=CARTESIAN_POINT('Ctrl Pts',(39.5433862983558,-5.80305606424513,-6.43225249093647));
#67788=CARTESIAN_POINT('Ctrl Pts',(39.6397260515868,-5.79674478524918,-6.44601126139509));
#67789=CARTESIAN_POINT('Ctrl Pts',(39.7361688337319,-5.79042675676303,-6.45978474593726));
#67790=CARTESIAN_POINT('Ctrl Pts',(39.8319101043967,-5.78410872827687,-6.47808613842611));
#67791=CARTESIAN_POINT('Ctrl Pts',(39.9265010452396,-5.77779069979071,-6.5008097142928));
#67792=CARTESIAN_POINT('Ctrl Pts',(40.021147413318,-5.77146896914397,-6.52354660544084));
#67793=CARTESIAN_POINT('Ctrl Pts',(40.1146416895832,-5.76514723849724,-6.55071071790727));
#67794=CARTESIAN_POINT('Ctrl Pts',(40.2065508087619,-5.7588255078505,-6.58214660197272));
#67795=CARTESIAN_POINT('Ctrl Pts',(40.2986072975196,-5.75249364076907,-6.61363289118881));
#67796=CARTESIAN_POINT('Ctrl Pts',(40.3890731474761,-5.74616177368765,-6.64940446849916));
#67797=CARTESIAN_POINT('Ctrl Pts',(40.4775358774011,-5.73982990660623,-6.68925799219093));
#67798=CARTESIAN_POINT('Ctrl Pts',(40.5289164862711,-5.7361522540377,-6.71240557439457));
#67799=CARTESIAN_POINT('Ctrl Pts',(40.5796218014761,-5.73247460146918,-6.73692932702247));
#67800=CARTESIAN_POINT('Ctrl Pts',(40.6295752793794,-5.72879694890065,-6.76278256223605));
#67801=CARTESIAN_POINT('Ctrl Pts',(40.715591126396,-5.72246432875102,-6.80729974138662));
#67802=CARTESIAN_POINT('Ctrl Pts',(40.7996749930196,-5.7161317086014,-6.85591588969245));
#67803=CARTESIAN_POINT('Ctrl Pts',(40.881410527064,-5.70979908845177,-6.90843941549633));
#67804=CARTESIAN_POINT('Ctrl Pts',(40.9630360581437,-5.7034749909967,-6.96089225302942));
#67805=CARTESIAN_POINT('Ctrl Pts',(41.0423191734523,-5.69715089354164,-7.01724178172022));
#67806=CARTESIAN_POINT('Ctrl Pts',(41.1188670403116,-5.69082679608657,-7.0772500261453));
#67807=CARTESIAN_POINT('Ctrl Pts',(41.1953347844096,-5.68450931807333,-7.13719545985538));
#67808=CARTESIAN_POINT('Ctrl Pts',(41.2690726294599,-5.67819184006008,-7.20079172751996));
#67809=CARTESIAN_POINT('Ctrl Pts',(41.3397165864681,-5.67187436204684,-7.26775752687196));
#67810=CARTESIAN_POINT('Ctrl Pts',(41.4103103980697,-5.66556136838749,-7.33467579169472));
#67811=CARTESIAN_POINT('Ctrl Pts',(41.4778143712153,-5.65924837472814,-7.40495853315345));
#67812=CARTESIAN_POINT('Ctrl Pts',(41.5418982421559,-5.6529353810688,-7.47828475935532));
#67813=CARTESIAN_POINT('Ctrl Pts',(41.6059589551157,-5.64662466873521,-7.55158448766765));
#67814=CARTESIAN_POINT('Ctrl Pts',(41.6666017341748,-5.64031395640162,-7.62792518641353));
#67815=CARTESIAN_POINT('Ctrl Pts',(41.723534449953,-5.63400324406803,-7.70695034919272));
#67816=CARTESIAN_POINT('Ctrl Pts',(41.7804620122632,-5.62769310297109,-7.78596835872728));
#67817=CARTESIAN_POINT('Ctrl Pts',(41.8336799235433,-5.62138296187415,-7.86766999422618));
#67818=CARTESIAN_POINT('Ctrl Pts',(41.8829381357321,-5.61507282077721,-7.95166799030393));
#67819=CARTESIAN_POINT('Ctrl Pts',(41.9322052305862,-5.60876154178126,-8.03568113362403));
#67820=CARTESIAN_POINT('Ctrl Pts',(41.9775109869771,-5.60245026278531,-8.12199108273024));
#67821=CARTESIAN_POINT('Ctrl Pts',(42.0186507773681,-5.59613898378937,-8.21018501372167));
#67822=CARTESIAN_POINT('Ctrl Pts',(42.0598345640097,-5.58982095530321,-8.29847326221576));
#67823=CARTESIAN_POINT('Ctrl Pts',(42.0968433048717,-5.58350292681706,-8.38864911804939));
#67824=CARTESIAN_POINT('Ctrl Pts',(42.1295201991624,-5.5771848983309,-8.48027895799909));
#67825=CARTESIAN_POINT('Ctrl Pts',(42.1622162410575,-5.57086316768416,-8.57196249007483));
#67826=CARTESIAN_POINT('Ctrl Pts',(42.1905752545655,-5.56454143703742,-8.6651012846412));
#67827=CARTESIAN_POINT('Ctrl Pts',(42.2144906887407,-5.55821970639069,-8.75924772909551));
#67828=CARTESIAN_POINT('Ctrl Pts',(42.2384444695729,-5.55188783930926,-8.85354513051687));
#67829=CARTESIAN_POINT('Ctrl Pts',(42.2579403562005,-5.54555597222784,-8.94885297991142));
#67830=CARTESIAN_POINT('Ctrl Pts',(42.272923153174,-5.53922410514642,-9.04471472270413));
#67831=CARTESIAN_POINT('Ctrl Pts',(42.2816254081433,-5.53554645257782,-9.1003927999724));
#67832=CARTESIAN_POINT('Ctrl Pts',(42.2888061551775,-5.53186880000923,-9.15625763958687));
#67833=CARTESIAN_POINT('Ctrl Pts',(42.2944626496101,-5.52819114744063,-9.21221962486703));
#67834=CARTESIAN_POINT('Ctrl Pts',(42.3042026753334,-5.521858527291,-9.30858163541264));
#67835=CARTESIAN_POINT('Ctrl Pts',(42.309454243118,-5.51552590714138,-9.40556641534358));
#67836=CARTESIAN_POINT('Ctrl Pts',(42.3101502022979,-5.50919328699175,-9.50272059142064));
#67837=CARTESIAN_POINT('Ctrl Pts',(42.3108452248279,-5.50286918953669,-9.59974401350508));
#67838=CARTESIAN_POINT('Ctrl Pts',(42.306996821536,-5.49654509208163,-9.69693594500563));
#67839=CARTESIAN_POINT('Ctrl Pts',(42.2985895388713,-5.49022099462656,-9.79383735324039));
#67840=CARTESIAN_POINT('Ctrl Pts',(42.2901910561214,-5.48390351661333,-9.89063733463299));
#67841=CARTESIAN_POINT('Ctrl Pts',(42.2772432181393,-5.47758603860009,-9.98714696391991));
#67842=CARTESIAN_POINT('Ctrl Pts',(42.2597826189743,-5.47126856058685,-10.0829076783148));
#67843=CARTESIAN_POINT('Ctrl Pts',(42.2423344139175,-5.46495556692751,-10.1786004186017));
#67844=CARTESIAN_POINT('Ctrl Pts',(42.2203798942647,-5.45864257326817,-10.2735448718582));
#67845=CARTESIAN_POINT('Ctrl Pts',(42.1940073242801,-5.45232957960883,-10.367289021095));
#67846=CARTESIAN_POINT('Ctrl Pts',(42.1676442845479,-5.44601886727525,-10.4609992940199));
#67847=CARTESIAN_POINT('Ctrl Pts',(42.1368664851563,-5.43970815494167,-10.5535097042536));
#67848=CARTESIAN_POINT('Ctrl Pts',(42.1018127745279,-5.43339744260809,-10.6443807549206));
#67849=CARTESIAN_POINT('Ctrl Pts',(42.0667622369112,-5.42708730151116,-10.7352435800702));
#67850=CARTESIAN_POINT('Ctrl Pts',(42.0274367151852,-5.42077716041423,-10.8244669327597));
#67851=CARTESIAN_POINT('Ctrl Pts',(41.984023817222,-5.41446701931729,-10.911629740789));
#67852=CARTESIAN_POINT('Ctrl Pts',(41.9406030906711,-5.40815574032136,-10.9988082667667));
#67853=CARTESIAN_POINT('Ctrl Pts',(41.893093718963,-5.40184446132542,-11.0839251186632));
#67854=CARTESIAN_POINT('Ctrl Pts',(41.8417295399151,-5.39553318232948,-11.166583287817));
#67855=CARTESIAN_POINT('Ctrl Pts',(41.7903104303177,-5.38921515384333,-11.2493298543469));
#67856=CARTESIAN_POINT('Ctrl Pts',(41.7350285143128,-5.38289712535718,-11.3296121166364));
#67857=CARTESIAN_POINT('Ctrl Pts',(41.6761611896886,-5.37657909687103,-11.4070617459531));
#67858=CARTESIAN_POINT('Ctrl Pts',(41.617259370714,-5.3702573662243,-11.4845567582504));
#67859=CARTESIAN_POINT('Ctrl Pts',(41.5547682401544,-5.36393563557758,-11.5592154972016));
#67860=CARTESIAN_POINT('Ctrl Pts',(41.4890043777611,-5.35761390493085,-11.6307040655065));
#67861=CARTESIAN_POINT('Ctrl Pts',(41.423135067804,-5.35128203784943,-11.7023072605241));
#67862=CARTESIAN_POINT('Ctrl Pts',(41.3539828581687,-5.34495017076802,-11.7707298273728));
#67863=CARTESIAN_POINT('Ctrl Pts',(41.2818998883338,-5.3386183036866,-11.8356759850433));
#67864=CARTESIAN_POINT('Ctrl Pts',(41.2400329135915,-5.33494065111796,-11.8733977818703));
#67865=CARTESIAN_POINT('Ctrl Pts',(41.1971778625174,-5.33126299854931,-11.9099475839306));
#67866=CARTESIAN_POINT('Ctrl Pts',(41.1534082781751,-5.32758534598067,-11.9452741067195));
#67867=CARTESIAN_POINT('Ctrl Pts',(41.0780405955099,-5.32125272583104,-12.0061035205517));
#67868=CARTESIAN_POINT('Ctrl Pts',(40.9996979413289,-5.31492010568141,-12.0635148002651));
#67869=CARTESIAN_POINT('Ctrl Pts',(40.9187232561712,-5.30858748553178,-12.1172038927515));
#67870=CARTESIAN_POINT('Ctrl Pts',(40.8378575499975,-5.30226338807672,-12.1708207283007));
#67871=CARTESIAN_POINT('Ctrl Pts',(40.7543672147178,-5.29593929062166,-12.2207250935565));
#67872=CARTESIAN_POINT('Ctrl Pts',(40.6686281886044,-5.2896151931666,-12.2666531320604));
#67873=CARTESIAN_POINT('Ctrl Pts',(40.5829789056518,-5.28329771515335,-12.312533097621));
#67874=CARTESIAN_POINT('Ctrl Pts',(40.4950859946145,-5.2769802371401,-12.3544448053281));
#67875=CARTESIAN_POINT('Ctrl Pts',(40.4053534504851,-5.27066275912686,-12.3921682392744));
#67876=CARTESIAN_POINT('Ctrl Pts',(40.31568460147,-5.26434976546752,-12.4298648958852));
#67877=CARTESIAN_POINT('Ctrl Pts',(40.2241791174292,-5.25803677180818,-12.4633790201888));
#67878=CARTESIAN_POINT('Ctrl Pts',(40.1312637559423,-5.25172377814884,-12.4925374420162));
#67879=CARTESIAN_POINT('Ctrl Pts',(40.0383819712683,-5.24541306581526,-12.5216853268683));
#67880=CARTESIAN_POINT('Ctrl Pts',(39.9440917383314,-5.23910235348167,-12.546480506031));
#67881=CARTESIAN_POINT('Ctrl Pts',(39.8488369808566,-5.23279164114809,-12.5667990113045));
#67882=CARTESIAN_POINT('Ctrl Pts',(39.753590845706,-5.22648150005116,-12.587115677376));
#67883=CARTESIAN_POINT('Ctrl Pts',(39.6573807873376,-5.22017135895423,-12.6029563842081));
#67884=CARTESIAN_POINT('Ctrl Pts',(39.560661953831,-5.2138612178573,-12.614248065138));
#67885=CARTESIAN_POINT('Ctrl Pts',(39.4639256791511,-5.20754993886136,-12.625541782281));
#67886=CARTESIAN_POINT('Ctrl Pts',(39.3666808814735,-5.20123865986541,-12.6322847935888));
#67887=CARTESIAN_POINT('Ctrl Pts',(39.2693878286774,-5.19492738086947,-12.6344558980843));
#67888=CARTESIAN_POINT('Ctrl Pts',(39.1719907274772,-5.18860935238332,-12.6366293244307));
#67889=CARTESIAN_POINT('Ctrl Pts',(39.0745457060551,-5.18229132389718,-12.6342210728767));
#67890=CARTESIAN_POINT('Ctrl Pts',(38.977512826952,-5.17597329541103,-12.6272620957503));
#67891=CARTESIAN_POINT('Ctrl Pts',(38.8804230897165,-5.16965156476429,-12.6202990408882));
#67892=CARTESIAN_POINT('Ctrl Pts',(38.7837464097462,-5.16332983411757,-12.6087800022855));
#67893=CARTESIAN_POINT('Ctrl Pts',(38.6879354349393,-5.15700810347083,-12.5927875633931));
#67894=CARTESIAN_POINT('Ctrl Pts',(38.5919708342123,-5.15067623638942,-12.5767694817896));
#67895=CARTESIAN_POINT('Ctrl Pts',(38.4968751376486,-5.144344369308,-12.556263769252));
#67896=CARTESIAN_POINT('Ctrl Pts',(38.4030885128886,-5.13801250222659,-12.5314036213739));
#67897=CARTESIAN_POINT('Ctrl Pts',(38.3486156983116,-5.13433484965795,-12.5169644385033));
#67898=CARTESIAN_POINT('Ctrl Pts',(38.2945841892687,-5.13065719708931,-12.5010572242992));
#67899=CARTESIAN_POINT('Ctrl Pts',(38.241077130484,-5.12697954452068,-12.4837155292828));
#67900=CARTESIAN_POINT('Ctrl Pts',(38.1489423047267,-5.12064692437105,-12.4538545336504));
#67901=CARTESIAN_POINT('Ctrl Pts',(38.0580435855754,-5.11431430422142,-12.4196339351882));
#67902=CARTESIAN_POINT('Ctrl Pts',(37.9688230392589,-5.10798168407179,-12.3811747047826));
#67903=CARTESIAN_POINT('Ctrl Pts',(37.8797225695374,-5.10165758661673,-12.3427672343542));
#67904=CARTESIAN_POINT('Ctrl Pts',(37.7922961818727,-5.09533348916167,-12.3001326416317));
#67905=CARTESIAN_POINT('Ctrl Pts',(37.7069703197477,-5.0890093917066,-12.253441501441));
#67906=CARTESIAN_POINT('Ctrl Pts',(37.621733768324,-5.08269191369335,-12.2067992329333));
#67907=CARTESIAN_POINT('Ctrl Pts',(37.538593753088,-5.0763744356801,-12.1561090670222));
#67908=CARTESIAN_POINT('Ctrl Pts',(37.4579553425894,-5.07005695766685,-12.1015890367863));
#67909=CARTESIAN_POINT('Ctrl Pts',(37.3773741718898,-5.06374396400751,-12.047107706663));
#67910=CARTESIAN_POINT('Ctrl Pts',(37.2992914369405,-5.05743097034817,-11.9888021611274));
#67911=CARTESIAN_POINT('Ctrl Pts',(37.224085420997,-5.05111797668883,-11.9269351009932));
#67912=CARTESIAN_POINT('Ctrl Pts',(37.1489065822425,-5.04480726435524,-11.8650903977512));
#67913=CARTESIAN_POINT('Ctrl Pts',(37.0766027342587,-5.03849655202166,-11.7996870147826));
#67914=CARTESIAN_POINT('Ctrl Pts',(37.007520342822,-5.03218583968808,-11.7310289222403));
#67915=CARTESIAN_POINT('Ctrl Pts',(36.9384442046246,-5.02587569859115,-11.6623770445304));
#67916=CARTESIAN_POINT('Ctrl Pts',(36.8725892532328,-5.01956555749422,-11.5904713514222));
#67917=CARTESIAN_POINT('Ctrl Pts',(36.8102654658623,-5.01325541639729,-11.5156530358779));
#67918=CARTESIAN_POINT('Ctrl Pts',(36.7479304397294,-5.00694413740134,-11.4408212284502));
#67919=CARTESIAN_POINT('Ctrl Pts',(36.6891281221875,-5.0006328584054,-11.3630760914411));
#67920=CARTESIAN_POINT('Ctrl Pts',(36.6341278576655,-4.99432157940945,-11.2827914558023));
#67921=CARTESIAN_POINT('Ctrl Pts',(36.5790687740441,-4.9880035509233,-11.2024209611226));
#67922=CARTESIAN_POINT('Ctrl Pts',(36.5278201086319,-4.98168552243715,-11.119505907188));
#67923=CARTESIAN_POINT('Ctrl Pts',(36.4806074214034,-4.975367493951,-11.0344484609862));
#67924=CARTESIAN_POINT('Ctrl Pts',(36.4333670690655,-4.96904576330426,-10.9493411738688));
#67925=CARTESIAN_POINT('Ctrl Pts',(36.3901675981309,-4.96272403265752,-10.8620893864293));
#67926=CARTESIAN_POINT('Ctrl Pts',(36.3511872806435,-4.95640230201078,-10.7731172793183));
#67927=CARTESIAN_POINT('Ctrl Pts',(36.312144461056,-4.95007043492936,-10.6840025119134));
#67928=CARTESIAN_POINT('Ctrl Pts',(36.2773344600279,-4.94373856784794,-10.5931623248813));
#67929=CARTESIAN_POINT('Ctrl Pts',(36.2468863459858,-4.93740670076652,-10.5010381136896));
#67930=CARTESIAN_POINT('Ctrl Pts',(36.2292015804377,-4.93372904819791,-10.4475308562624));
#67931=CARTESIAN_POINT('Ctrl Pts',(36.2129873431153,-4.93005139562931,-10.3935906862479));
#67932=CARTESIAN_POINT('Ctrl Pts',(36.1982609879107,-4.9263737430607,-10.3393055668488));
#67933=CARTESIAN_POINT('Ctrl Pts',(36.1660748354605,-4.91833580803964,-10.2206591601533));
#67934=CARTESIAN_POINT('Ctrl Pts',(36.1409082916263,-4.91029787301858,-10.1000336223966));
#67935=CARTESIAN_POINT('Ctrl Pts',(36.1229598946395,-4.90225993799752,-9.97816094591516));
#67936=CARTESIAN_POINT('Ctrl Pts',(36.1053275701443,-4.89436355155888,-9.85843445555557));
#67937=CARTESIAN_POINT('Ctrl Pts',(36.0946614047826,-4.88646716512023,-9.73750420175503));
#67938=CARTESIAN_POINT('Ctrl Pts',(36.0911040387368,-4.87857077868159,-9.61608542661328));
#67939=CARTESIAN_POINT('Ctrl Pts',(36.0902419309021,-4.87665713343755,-9.58666026316763));
#67940=CARTESIAN_POINT('Ctrl Pts',(36.0897971143992,-4.87474348819351,-9.55720651418373));
#67941=CARTESIAN_POINT('Ctrl Pts',(36.0897712021404,-4.87282984294947,-9.52773456847233));
#67942=CARTESIAN_POINT('',(36.0898800655558,-3.60282980867964,-9.52346476277984));
#67943=CARTESIAN_POINT('Ctrl Pts',(36.0897712021399,-4.87282984291314,-9.52773456791281));
#67944=CARTESIAN_POINT('Ctrl Pts',(36.089686528353,-4.86657660100476,-9.43142873138466));
#67945=CARTESIAN_POINT('Ctrl Pts',(36.0940791608739,-4.86032335909639,-9.33502132983258));
#67946=CARTESIAN_POINT('Ctrl Pts',(36.1029506472896,-4.85407011718802,-9.23896510741516));
#67947=CARTESIAN_POINT('Ctrl Pts',(36.1118176278476,-4.84782005132219,-9.14295767227547));
#67948=CARTESIAN_POINT('Ctrl Pts',(36.1251589041781,-4.84156998545637,-9.04730150610461));
#67949=CARTESIAN_POINT('Ctrl Pts',(36.1429239802186,-4.83531991959055,-8.95244706604761));
#67950=CARTESIAN_POINT('Ctrl Pts',(36.1606850819456,-4.82907125195803,-8.85761384634896));
#67951=CARTESIAN_POINT('Ctrl Pts',(36.1828679350296,-4.82282258432551,-8.76358243547113));
#67952=CARTESIAN_POINT('Ctrl Pts',(36.2093706344023,-4.816573916693,-8.67079472576857));
#67953=CARTESIAN_POINT('Ctrl Pts',(36.2358749365348,-4.81032487117019,-8.5780014046978));
#67954=CARTESIAN_POINT('Ctrl Pts',(36.2666994798357,-4.80407582564738,-8.48645236351399));
#67955=CARTESIAN_POINT('Ctrl Pts',(36.3016923605483,-4.79782678012457,-8.39657477873092));
#67956=CARTESIAN_POINT('Ctrl Pts',(36.3367199778045,-4.79157153133306,-8.30660797475332));
#67957=CARTESIAN_POINT('Ctrl Pts',(36.3759240331927,-4.78531628254155,-8.2183163578517));
#67958=CARTESIAN_POINT('Ctrl Pts',(36.4191043846771,-4.77906103375005,-8.13210724405014));
#67959=CARTESIAN_POINT('Ctrl Pts',(36.4623064306282,-4.77280264222621,-8.04585481747588));
#67960=CARTESIAN_POINT('Ctrl Pts',(36.509488531073,-4.76654425070238,-7.96168736670024));
#67961=CARTESIAN_POINT('Ctrl Pts',(36.5604055732342,-4.76028585917854,-7.87998574015689));
#67962=CARTESIAN_POINT('Ctrl Pts',(36.6114083467711,-4.75401693011184,-7.79814654881139));
#67963=CARTESIAN_POINT('Ctrl Pts',(36.6661583687463,-4.74774800104514,-7.71878184229606));
#67964=CARTESIAN_POINT('Ctrl Pts',(36.7243683708865,-4.74147907197844,-7.64224173356406));
#67965=CARTESIAN_POINT('Ctrl Pts',(36.7729968220505,-4.7362420285192,-7.57830036949065));
#67966=CARTESIAN_POINT('Ctrl Pts',(36.8240391302687,-4.73100498505996,-7.51632976422507));
#67967=CARTESIAN_POINT('Ctrl Pts',(36.8773082980014,-4.72576794160072,-7.45651410196568));
#67968=CARTESIAN_POINT('Ctrl Pts',(36.9417212454141,-4.7194353214511,-7.3841851493734));
#67969=CARTESIAN_POINT('Ctrl Pts',(37.0096277937264,-4.71310270130147,-7.31474217133556));
#67970=CARTESIAN_POINT('Ctrl Pts',(37.0807393049553,-4.70677008115185,-7.24854117995982));
#67971=CARTESIAN_POINT('Ctrl Pts',(37.1517551114562,-4.70044598369678,-7.18242928453731));
#67972=CARTESIAN_POINT('Ctrl Pts',(37.2259669904762,-4.6941218862417,-7.11955099918333));
#67973=CARTESIAN_POINT('Ctrl Pts',(37.3030471805889,-4.68779778878663,-7.06022807265494));
#67974=CARTESIAN_POINT('Ctrl Pts',(37.3800466907567,-4.68148031077339,-7.00096723951837));
#67975=CARTESIAN_POINT('Ctrl Pts',(37.4599081986313,-4.67516283276015,-6.94525463220614));
#67976=CARTESIAN_POINT('Ctrl Pts',(37.5422690983968,-4.6688453547469,-6.8933733337022));
#67977=CARTESIAN_POINT('Ctrl Pts',(37.6245715356838,-4.66253236108756,-6.84152886225219));
#67978=CARTESIAN_POINT('Ctrl Pts',(37.7093694687744,-4.65621936742822,-6.79351052532837));
#67979=CARTESIAN_POINT('Ctrl Pts',(37.7962701792758,-4.64990637376888,-6.74955891013526));
#67980=CARTESIAN_POINT('Ctrl Pts',(37.8831394864779,-4.64359566143529,-6.70562317773202));
#67981=CARTESIAN_POINT('Ctrl Pts',(37.9721096713557,-4.63728494910171,-6.6657514441378));
#67982=CARTESIAN_POINT('Ctrl Pts',(38.0627630390549,-4.63097423676812,-6.63013856159568));
#67983=CARTESIAN_POINT('Ctrl Pts',(38.1534082009409,-4.62466409567119,-6.59452890268074));
#67984=CARTESIAN_POINT('Ctrl Pts',(38.2457358356171,-4.61835395457426,-6.56317748805104));
#67985=CARTESIAN_POINT('Ctrl Pts',(38.3393088559079,-4.61204381347733,-6.53623078719995));
#67986=CARTESIAN_POINT('Ctrl Pts',(38.432898750092,-4.60573253448138,-6.50927922708757));
#67987=CARTESIAN_POINT('Ctrl Pts',(38.5277340556931,-4.59942125548543,-6.48673407930736));
#67988=CARTESIAN_POINT('Ctrl Pts',(38.6233641581208,-4.59310997648948,-6.46869148174464));
#67989=CARTESIAN_POINT('Ctrl Pts',(38.7190965305384,-4.58679194800333,-6.4506295888322));
#67990=CARTESIAN_POINT('Ctrl Pts',(38.8156249662858,-4.58047391951718,-6.43707994058349));
#67991=CARTESIAN_POINT('Ctrl Pts',(38.9124905298923,-4.57415589103103,-6.42808718923209));
#67992=CARTESIAN_POINT('Ctrl Pts',(39.0094128535899,-4.5678341603843,-6.41908916841891));
#67993=CARTESIAN_POINT('Ctrl Pts',(39.1066722618487,-4.56151242973756,-6.41465338150445));
#67994=CARTESIAN_POINT('Ctrl Pts',(39.2038086960325,-4.55519069909083,-6.41477233200936));
#67995=CARTESIAN_POINT('Ctrl Pts',(39.3011008814141,-4.54885883200941,-6.41489147324274));
#67996=CARTESIAN_POINT('Ctrl Pts',(39.3982692624579,-4.542526964928,-6.41957991402117));
#67997=CARTESIAN_POINT('Ctrl Pts',(39.4948578214015,-4.53619509784658,-6.42877818655408));
#67998=CARTESIAN_POINT('Ctrl Pts',(39.5509580454476,-4.53251744527797,-6.43412069456515));
#67999=CARTESIAN_POINT('Ctrl Pts',(39.6068628189766,-4.52883979270935,-6.4409836188567));
#68000=CARTESIAN_POINT('Ctrl Pts',(39.6624846319725,-4.52516214014074,-6.44934744841209));
#68001=CARTESIAN_POINT('Ctrl Pts',(39.758260893369,-4.51882951999112,-6.46374928615569));
#68002=CARTESIAN_POINT('Ctrl Pts',(39.853530161358,-4.51249689984149,-6.48265412890254));
#68003=CARTESIAN_POINT('Ctrl Pts',(39.9478365430096,-4.50616427969187,-6.50601487949353));
#68004=CARTESIAN_POINT('Ctrl Pts',(40.0420160033448,-4.4998401822368,-6.52934419024806));
#68005=CARTESIAN_POINT('Ctrl Pts',(40.1352347320877,-4.49351608478173,-6.55711738538795));
#68006=CARTESIAN_POINT('Ctrl Pts',(40.2270441421906,-4.48719198732666,-6.58923587751127));
#68007=CARTESIAN_POINT('Ctrl Pts',(40.318757455253,-4.48087450931341,-6.62132075116313));
#68008=CARTESIAN_POINT('Ctrl Pts',(40.4090639717026,-4.47455703130016,-6.65774173605245));
#68009=CARTESIAN_POINT('Ctrl Pts',(40.4975284358924,-4.4682395532869,-6.6983499312878));
#68010=CARTESIAN_POINT('Ctrl Pts',(40.5859301050926,-4.46192655962756,-6.73892930148905));
#68011=CARTESIAN_POINT('Ctrl Pts',(40.6724919252063,-4.45561356596822,-6.78368979116446));
#68012=CARTESIAN_POINT('Ctrl Pts',(40.7567977656624,-4.44930057230888,-6.83243405471126));
#68013=CARTESIAN_POINT('Ctrl Pts',(40.841073140527,-4.4429898599753,-6.88116070354941));
#68014=CARTESIAN_POINT('Ctrl Pts',(40.9230937774273,-4.43667914764172,-6.93386804705558));
#68015=CARTESIAN_POINT('Ctrl Pts',(41.0024681907966,-4.43036843530814,-6.99031282520575));
#68016=CARTESIAN_POINT('Ctrl Pts',(41.0818354193077,-4.4240582942112,-7.04675249405542));
#68017=CARTESIAN_POINT('Ctrl Pts',(41.1585565442667,-4.41774815311426,-7.10692867131198));
#68018=CARTESIAN_POINT('Ctrl Pts',(41.2322699947175,-4.41143801201733,-7.17055541125491));
#68019=CARTESIAN_POINT('Ctrl Pts',(41.3059967378123,-4.40512673302141,-7.23419362491946));
#68020=CARTESIAN_POINT('Ctrl Pts',(41.3767143981656,-4.3988154540255,-7.3012833513382));
#68021=CARTESIAN_POINT('Ctrl Pts',(41.4440961572377,-4.39250417502958,-7.37149980497542));
#68022=CARTESIAN_POINT('Ctrl Pts',(41.5115499765888,-4.38618614654343,-7.44179135040758));
#68023=CARTESIAN_POINT('Ctrl Pts',(41.5756604690033,-4.37986811805728,-7.51521598277214));
#68024=CARTESIAN_POINT('Ctrl Pts',(41.6361393807236,-4.37355008957113,-7.5914138057517));
#68025=CARTESIAN_POINT('Ctrl Pts',(41.6966537311323,-4.3672283589244,-7.6676562781939));
#68026=CARTESIAN_POINT('Ctrl Pts',(41.7535320080731,-4.36090662827766,-7.7466748223001));
#68027=CARTESIAN_POINT('Ctrl Pts',(41.8065290122119,-4.35458489763093,-7.82808009576247));
#68028=CARTESIAN_POINT('Ctrl Pts',(41.8596109931871,-4.34825303054952,-7.90961589665206));
#68029=CARTESIAN_POINT('Ctrl Pts',(41.9087990534684,-4.34192116346811,-7.99354569158422));
#68030=CARTESIAN_POINT('Ctrl Pts',(41.9538937223544,-4.33558929638669,-8.07945511350316));
#68031=CARTESIAN_POINT('Ctrl Pts',(41.9800854479115,-4.33191164381805,-8.12935271907964));
#68032=CARTESIAN_POINT('Ctrl Pts',(42.0048971680573,-4.3282339912494,-8.17991774628832));
#68033=CARTESIAN_POINT('Ctrl Pts',(42.0282973863272,-4.32455633868076,-8.23106625077054));
#68034=CARTESIAN_POINT('Ctrl Pts',(42.0685906687826,-4.31822371853114,-8.31913983685877));
#68035=CARTESIAN_POINT('Ctrl Pts',(42.104836085978,-4.31189109838151,-8.40925030370235));
#68036=CARTESIAN_POINT('Ctrl Pts',(42.1368238765099,-4.30555847823189,-8.50099015079872));
#68037=CARTESIAN_POINT('Ctrl Pts',(42.1687686165885,-4.29923438077683,-8.59260653072394));
#68038=CARTESIAN_POINT('Ctrl Pts',(42.1964669760499,-4.29291028332177,-8.68584752299583));
#68039=CARTESIAN_POINT('Ctrl Pts',(42.2197563040006,-4.28658618586671,-8.78028359938236));
#68040=CARTESIAN_POINT('Ctrl Pts',(42.2430212549784,-4.28026870785348,-8.87462082939295));
#68041=CARTESIAN_POINT('Ctrl Pts',(42.2618862450071,-4.27395122984026,-8.97015023431466));
#68042=CARTESIAN_POINT('Ctrl Pts',(42.276238041974,-4.26763375182703,-9.06642594707965));
#68043=CARTESIAN_POINT('Ctrl Pts',(42.290579651563,-4.26132075816769,-9.16263332017403));
#68044=CARTESIAN_POINT('Ctrl Pts',(42.3004143727697,-4.25500776450834,-9.25958551662242));
#68045=CARTESIAN_POINT('Ctrl Pts',(42.3056799943147,-4.248694770849,-9.35682620354653));
#68046=CARTESIAN_POINT('Ctrl Pts',(42.3109437130226,-4.24238405851542,-9.45403175061534));
#68047=CARTESIAN_POINT('Ctrl Pts',(42.3116415892697,-4.23607334618183,-9.55152514478004));
#68048=CARTESIAN_POINT('Ctrl Pts',(42.3077633310885,-4.22976263384824,-9.64884559274261));
#68049=CARTESIAN_POINT('Ctrl Pts',(42.3038854239617,-4.22345249275131,-9.74615723139746));
#68050=CARTESIAN_POINT('Ctrl Pts',(42.2954322236033,-4.21714235165438,-9.84329551801961));
#68051=CARTESIAN_POINT('Ctrl Pts',(42.2824455341499,-4.21083221055745,-9.93980137644355));
#68052=CARTESIAN_POINT('Ctrl Pts',(42.2694565028247,-4.20452093156151,-10.0363246376352));
#68053=CARTESIAN_POINT('Ctrl Pts',(42.2519324170684,-4.19820965256559,-10.1322148107252));
#68054=CARTESIAN_POINT('Ctrl Pts',(42.2299666010881,-4.19189837356966,-10.2270206900018));
#68055=CARTESIAN_POINT('Ctrl Pts',(42.2079772941387,-4.18558034508351,-10.3219279578171));
#68056=CARTESIAN_POINT('Ctrl Pts',(42.1815368724549,-4.17926231659735,-10.4157481900525));
#68057=CARTESIAN_POINT('Ctrl Pts',(42.1507891416017,-4.1729442881112,-10.5080432822138));
#68058=CARTESIAN_POINT('Ctrl Pts',(42.1200233935715,-4.16662255746446,-10.6003924563177));
#68059=CARTESIAN_POINT('Ctrl Pts',(42.0849454679997,-4.16030082681771,-10.6912143030178));
#68060=CARTESIAN_POINT('Ctrl Pts',(42.0457473623408,-4.15397909617096,-10.7800906750632));
#68061=CARTESIAN_POINT('Ctrl Pts',(42.0064864053742,-4.14764722908955,-10.8691095538983));
#68062=CARTESIAN_POINT('Ctrl Pts',(41.9630922714297,-4.14131536200813,-10.9561763379827));
#68063=CARTESIAN_POINT('Ctrl Pts',(41.9158029093577,-4.13498349492671,-11.0408974933763));
#68064=CARTESIAN_POINT('Ctrl Pts',(41.8883364698924,-4.13130584235806,-11.0901049342062));
#68065=CARTESIAN_POINT('Ctrl Pts',(41.8595568068561,-4.12762818978942,-11.1385216093164));
#68066=CARTESIAN_POINT('Ctrl Pts',(41.829516997139,-4.12395053722077,-11.1860752585771));
#68067=CARTESIAN_POINT('Ctrl Pts',(41.7777908754473,-4.11761791707114,-11.267958794848));
#68068=CARTESIAN_POINT('Ctrl Pts',(41.7221464678276,-4.11128529692151,-11.3475661211635));
#68069=CARTESIAN_POINT('Ctrl Pts',(41.6628103481133,-4.10495267677189,-11.4244988397275));
#68070=CARTESIAN_POINT('Ctrl Pts',(41.6035540853321,-4.09862857931681,-11.5013280191488));
#68071=CARTESIAN_POINT('Ctrl Pts',(41.5406162503143,-4.09230448186174,-11.5754894018221));
#68072=CARTESIAN_POINT('Ctrl Pts',(41.4742676140015,-4.08598038440666,-11.6466119986473));
#68073=CARTESIAN_POINT('Ctrl Pts',(41.407988424901,-4.07966290639342,-11.7176601513489));
#68074=CARTESIAN_POINT('Ctrl Pts',(41.3383058287592,-4.07334542838017,-11.7856755234971));
#68075=CARTESIAN_POINT('Ctrl Pts',(41.2655312915966,-4.06702795036693,-11.8503195772485));
#68076=CARTESIAN_POINT('Ctrl Pts',(41.1928084121967,-4.06071495670759,-11.9149177445221));
#68077=CARTESIAN_POINT('Ctrl Pts',(41.1169982811168,-4.05440196304824,-11.9761490613708));
#68078=CARTESIAN_POINT('Ctrl Pts',(41.0384490172052,-4.0480889693889,-12.0337119930429));
#68079=CARTESIAN_POINT('Ctrl Pts',(40.9599281386316,-4.04177825705531,-12.0912541232053));
#68080=CARTESIAN_POINT('Ctrl Pts',(40.8786704464283,-4.03546754472172,-12.1451302440273));
#68081=CARTESIAN_POINT('Ctrl Pts',(40.7950561745941,-4.02915683238813,-12.1950798588786));
#68082=CARTESIAN_POINT('Ctrl Pts',(40.711449471404,-4.02284669129119,-12.2450249523624));
#68083=CARTESIAN_POINT('Ctrl Pts',(40.625486988232,-4.01653655019425,-12.2910440224433));
#68084=CARTESIAN_POINT('Ctrl Pts',(40.537575997897,-4.01022640909731,-12.3329211354221));
#68085=CARTESIAN_POINT('Ctrl Pts',(40.449649154695,-4.00391513010138,-12.3748058000425));
#68086=CARTESIAN_POINT('Ctrl Pts',(40.3597735012785,-3.99760385110545,-12.4125468360616));
#68087=CARTESIAN_POINT('Ctrl Pts',(40.2683778817386,-3.99129257210951,-12.4459757538726));
#68088=CARTESIAN_POINT('Ctrl Pts',(40.1768845207044,-3.98497454362336,-12.4794404216725));
#68089=CARTESIAN_POINT('Ctrl Pts',(40.0838683597006,-3.9786565151372,-12.5085836141476));
#68090=CARTESIAN_POINT('Ctrl Pts',(39.9897748661653,-3.97233848665105,-12.5332862752194));
#68091=CARTESIAN_POINT('Ctrl Pts',(39.8956262368825,-3.96601675600431,-12.5580034112527));
#68092=CARTESIAN_POINT('Ctrl Pts',(39.8003994455534,-3.95969502535756,-12.5782747435621));
#68093=CARTESIAN_POINT('Ctrl Pts',(39.7045495903878,-3.95337329471082,-12.5940324800724));
#68094=CARTESIAN_POINT('Ctrl Pts',(39.6085460469604,-3.94704142762941,-12.6098154829656));
#68095=CARTESIAN_POINT('Ctrl Pts',(39.511917878896,-3.940709560548,-12.6210703880341));
#68096=CARTESIAN_POINT('Ctrl Pts',(39.4151246915751,-3.93437769346659,-12.6277813361522));
#68097=CARTESIAN_POINT('Ctrl Pts',(39.3589056160012,-3.93070004089799,-12.6316791652234));
#68098=CARTESIAN_POINT('Ctrl Pts',(39.3026308801833,-3.92702238832939,-12.634045077682));
#68099=CARTESIAN_POINT('Ctrl Pts',(39.2463900062488,-3.92334473576079,-12.6348840203809));
#68100=CARTESIAN_POINT('Ctrl Pts',(39.1495477720066,-3.91701211561117,-12.6363286118261));
#68101=CARTESIAN_POINT('Ctrl Pts',(39.0524697847135,-3.91067949546155,-12.6332478837387));
#68102=CARTESIAN_POINT('Ctrl Pts',(38.9556135048535,-3.90434687531193,-12.6256137930884));
#68103=CARTESIAN_POINT('Ctrl Pts',(38.8588875780654,-3.89802277785687,-12.617989976704));
#68104=CARTESIAN_POINT('Ctrl Pts',(38.76238319794,-3.89169868040181,-12.6058250117094));
#68105=CARTESIAN_POINT('Ctrl Pts',(38.6665590324013,-3.88537458294675,-12.5891428470271));
#68106=CARTESIAN_POINT('Ctrl Pts',(38.5708351661537,-3.87905710493354,-12.5724781435904));
#68107=CARTESIAN_POINT('Ctrl Pts',(38.4757905276088,-3.87273962692033,-12.5513057148846));
#68108=CARTESIAN_POINT('Ctrl Pts',(38.381878855308,-3.86642214890712,-12.5257013256084));
#68109=CARTESIAN_POINT('Ctrl Pts',(38.2880338446038,-3.86010915524777,-12.5001151111705));
#68110=CARTESIAN_POINT('Ctrl Pts',(38.195320622029,-3.85379616158843,-12.4701033052074));
#68111=CARTESIAN_POINT('Ctrl Pts',(38.1041819755489,-3.84748316792909,-12.4357925914067));
#68112=CARTESIAN_POINT('Ctrl Pts',(38.0130762638306,-3.8411724555955,-12.4014942764645));
#68113=CARTESIAN_POINT('Ctrl Pts',(37.9235444064454,-3.83486174326192,-12.3629002944186));
#68114=CARTESIAN_POINT('Ctrl Pts',(37.8360123815432,-3.82855103092834,-12.3201866538027));
#68115=CARTESIAN_POINT('Ctrl Pts',(37.7484882799147,-3.8222408898314,-12.2774768795643));
#68116=CARTESIAN_POINT('Ctrl Pts',(37.662964043779,-3.81593074873447,-12.2306483801479));
#68117=CARTESIAN_POINT('Ctrl Pts',(37.5798431150426,-3.80962060763754,-12.179924164835));
#68118=CARTESIAN_POINT('Ctrl Pts',(37.4967071972242,-3.8033093286416,-12.1291908024947));
#68119=CARTESIAN_POINT('Ctrl Pts',(37.415975820834,-3.79699804964566,-12.0745605568153));
#68120=CARTESIAN_POINT('Ctrl Pts',(37.338024490238,-3.79068677064972,-12.0163004343007));
#68121=CARTESIAN_POINT('Ctrl Pts',(37.2599897959144,-3.78436874216357,-11.9579780064867));
#68122=CARTESIAN_POINT('Ctrl Pts',(37.1847414338276,-3.77805071367743,-11.8960182140504));
#68123=CARTESIAN_POINT('Ctrl Pts',(37.1126226002573,-3.77173268519128,-11.8307290048796));
#68124=CARTESIAN_POINT('Ctrl Pts',(37.0404615073804,-3.76541095454456,-11.7654015383417));
#68125=CARTESIAN_POINT('Ctrl Pts',(36.9714339045352,-3.75908922389784,-11.696741078499));
#68126=CARTESIAN_POINT('Ctrl Pts',(36.9058453248355,-3.75276749325112,-11.6250916597427));
#68127=CARTESIAN_POINT('Ctrl Pts',(36.8401515786248,-3.74643562616969,-11.5533273563614));
#68128=CARTESIAN_POINT('Ctrl Pts',(36.7779081461245,-3.74010375908826,-11.4785648599999));
#68129=CARTESIAN_POINT('Ctrl Pts',(36.7193795364619,-3.73377189200683,-11.4011803668027));
#68130=CARTESIAN_POINT('Ctrl Pts',(36.685385157095,-3.73009423943816,-11.3562341800741));
#68131=CARTESIAN_POINT('Ctrl Pts',(36.652643151416,-3.72641658686948,-11.3104040099088));
#68132=CARTESIAN_POINT('Ctrl Pts',(36.6211983115091,-3.7227389343008,-11.2637675245231));
#68133=CARTESIAN_POINT('Ctrl Pts',(36.5662323739882,-3.71631035581507,-11.182246418056));
#68134=CARTESIAN_POINT('Ctrl Pts',(36.5150453840929,-3.70988177732934,-11.0979827664567));
#68135=CARTESIAN_POINT('Ctrl Pts',(36.467916808164,-3.70345319884361,-11.0113553026741));
#68136=CARTESIAN_POINT('Ctrl Pts',(36.4208567825603,-3.69703397097238,-10.9248538418673));
#68137=CARTESIAN_POINT('Ctrl Pts',(36.3778436321412,-3.69061474310115,-10.8359957709156));
#68138=CARTESIAN_POINT('Ctrl Pts',(36.339113950261,-3.68419551522991,-10.7451891916045));
#68139=CARTESIAN_POINT('Ctrl Pts',(36.3004312822952,-3.67778407965171,-10.6544928422914));
#68140=CARTESIAN_POINT('Ctrl Pts',(36.2660219051206,-3.6713726440735,-10.561853072782));
#68141=CARTESIAN_POINT('Ctrl Pts',(36.2360764098612,-3.6649612084953,-10.4677022884871));
#68142=CARTESIAN_POINT('Ctrl Pts',(36.2061647874513,-3.65855702521297,-10.3736580028596));
#68143=CARTESIAN_POINT('Ctrl Pts',(36.1807071210664,-3.65215284193065,-10.2781065038215));
#68144=CARTESIAN_POINT('Ctrl Pts',(36.1598454211839,-3.64574865864833,-10.1814988878921));
#68145=CARTESIAN_POINT('Ctrl Pts',(36.1389974530624,-3.63934869078057,-10.0849548618279));
#68146=CARTESIAN_POINT('Ctrl Pts',(36.122739522412,-3.63294872291281,-9.98735651102084));
#68147=CARTESIAN_POINT('Ctrl Pts',(36.1111633069834,-3.62654875504505,-9.889168280846));
#68148=CARTESIAN_POINT('Ctrl Pts',(36.0995920289091,-3.62015151681797,-9.7910219287856));
#68149=CARTESIAN_POINT('Ctrl Pts',(36.092698541246,-3.61375427859088,-9.692286614564));
#68150=CARTESIAN_POINT('Ctrl Pts',(36.0905229700006,-3.60735704036379,-9.59343429553861));
#68151=CARTESIAN_POINT('Ctrl Pts',(36.0900097672587,-3.60584797454691,-9.5701156930002));
#68152=CARTESIAN_POINT('Ctrl Pts',(36.0897588686184,-3.60433890873002,-9.54679059957209));
#68153=CARTESIAN_POINT('Ctrl Pts',(36.0897703786693,-3.60282984291314,-9.52346523708319));
#68154=CARTESIAN_POINT('',(36.0895800927968,-2.33282991063404,-9.52372422996978));
#68155=CARTESIAN_POINT('Ctrl Pts',(36.0939567706053,-3.60282853633159,-9.52344713446587));
#68156=CARTESIAN_POINT('Ctrl Pts',(36.0920877916079,-3.57593006850133,-9.10824092314765));
#68157=CARTESIAN_POINT('Ctrl Pts',(36.3622061427194,-3.48216300018445,-7.66318432907408));
#68158=CARTESIAN_POINT('Ctrl Pts',(38.5462979006151,-3.32152733138084,-5.91383345726613));
#68159=CARTESIAN_POINT('Ctrl Pts',(41.8665981283961,-3.12092152992086,-7.00367006210291));
#68160=CARTESIAN_POINT('Ctrl Pts',(42.768927986537,-2.92031572846088,-10.3797533334323));
#68161=CARTESIAN_POINT('Ctrl Pts',(40.435088873085,-2.71970992700091,-12.9807785967394));
#68162=CARTESIAN_POINT('Ctrl Pts',(37.0635739275412,-2.52388181452703,-12.460917710667));
#68163=CARTESIAN_POINT('Ctrl Pts',(36.0904109778155,-2.39492230253986,-10.475455999417));
#68164=CARTESIAN_POINT('Ctrl Pts',(36.0854229188962,-2.33283139103934,-9.52374521463249));
#68165=CARTESIAN_POINT('',(36.0897712174216,-1.06282984297027,-9.52775189410162));
#68166=CARTESIAN_POINT('Ctrl Pts',(36.0897702620449,-2.33282984291314,-9.52372327002978));
#68167=CARTESIAN_POINT('Ctrl Pts',(36.0898002776313,-2.32805266996907,-9.45060258528132));
#68168=CARTESIAN_POINT('Ctrl Pts',(36.092408661042,-2.323275497025,-9.37753813353249));
#68169=CARTESIAN_POINT('Ctrl Pts',(36.0975847896046,-2.31849832408093,-9.30465818552244));
#68170=CARTESIAN_POINT('Ctrl Pts',(36.1044462652967,-2.31216570393131,-9.20804853109387));
#68171=CARTESIAN_POINT('Ctrl Pts',(36.1158366136766,-2.30583308378168,-9.1115918752));
#68172=CARTESIAN_POINT('Ctrl Pts',(36.1317445637288,-2.29950046363206,-9.01574639844953));
#68173=CARTESIAN_POINT('Ctrl Pts',(36.1476311042228,-2.293176366177,-8.92002991439162));
#68174=CARTESIAN_POINT('Ctrl Pts',(36.1680230911667,-2.28685226872195,-8.82492340238974));
#68175=CARTESIAN_POINT('Ctrl Pts',(36.1928573494404,-2.28052817126689,-8.73088178960229));
#68176=CARTESIAN_POINT('Ctrl Pts',(36.2176656136605,-2.27421069325365,-8.63693861030494));
#68177=CARTESIAN_POINT('Ctrl Pts',(36.2469067942496,-2.26789321524041,-8.54405853487825));
#68178=CARTESIAN_POINT('Ctrl Pts',(36.2804665135229,-2.26157573722717,-8.45268713789364));
#68179=CARTESIAN_POINT('Ctrl Pts',(36.3140024110025,-2.25526274356783,-8.36138059933508));
#68180=CARTESIAN_POINT('Ctrl Pts',(36.3518506025418,-2.2489497499085,-8.27158101952218));
#68181=CARTESIAN_POINT('Ctrl Pts',(36.3938469174799,-2.24263675624916,-8.18371869827279));
#68182=CARTESIAN_POINT('Ctrl Pts',(36.4358280562148,-2.23632604391558,-8.09588812781981));
#68183=CARTESIAN_POINT('Ctrl Pts',(36.4819541514066,-2.23001533158199,-8.00999381904815));
#68184=CARTESIAN_POINT('Ctrl Pts',(36.5320133299145,-2.22370461924841,-7.92644509598633));
#68185=CARTESIAN_POINT('Ctrl Pts',(36.5820679771372,-2.21739447815148,-7.84290393563538));
#68186=CARTESIAN_POINT('Ctrl Pts',(36.6360547748898,-2.21108433705455,-7.76170831387778));
#68187=CARTESIAN_POINT('Ctrl Pts',(36.6937169539322,-2.20477419595762,-7.68324107280751));
#68188=CARTESIAN_POINT('Ctrl Pts',(36.7513895311155,-2.19846291696169,-7.60475968184839));
#68189=CARTESIAN_POINT('Ctrl Pts',(36.8127385469611,-2.19215163796576,-7.52900800113037));
#68190=CARTESIAN_POINT('Ctrl Pts',(36.8774657915695,-2.18584035896983,-7.45633726683872));
#68191=CARTESIAN_POINT('Ctrl Pts',(36.9422622576313,-2.17952233048368,-7.38358881606356));
#68192=CARTESIAN_POINT('Ctrl Pts',(37.0104438738492,-2.17320430199754,-7.31392821683122));
#68193=CARTESIAN_POINT('Ctrl Pts',(37.0816744088738,-2.16688627351139,-7.24767100688552));
#68194=CARTESIAN_POINT('Ctrl Pts',(37.1529466826908,-2.16056454286467,-7.18137497235528));
#68195=CARTESIAN_POINT('Ctrl Pts',(37.2272710991643,-2.15424281221793,-7.11848658061029));
#68196=CARTESIAN_POINT('Ctrl Pts',(37.304278701515,-2.14792108157121,-7.05928075171351));
#68197=CARTESIAN_POINT('Ctrl Pts',(37.3814097799477,-2.14158921448979,-6.99997999058203));
#68198=CARTESIAN_POINT('Ctrl Pts',(37.4612322765795,-2.13525734740838,-6.94437383280194));
#68199=CARTESIAN_POINT('Ctrl Pts',(37.5433487075768,-2.12892548032697,-6.89269356870965));
#68200=CARTESIAN_POINT('Ctrl Pts',(37.5910432816265,-2.1252478277583,-6.86267682111454));
#68201=CARTESIAN_POINT('Ctrl Pts',(37.6395112396921,-2.12157017518962,-6.83398360808067));
#68202=CARTESIAN_POINT('Ctrl Pts',(37.6886713600782,-2.11789252262095,-6.80665189958092));
#68203=CARTESIAN_POINT('Ctrl Pts',(37.7733211096405,-2.11155990247132,-6.7595889090625));
#68204=CARTESIAN_POINT('Ctrl Pts',(37.8603183084808,-2.10522728232169,-6.7164019446356));
#68205=CARTESIAN_POINT('Ctrl Pts',(37.9492731236839,-2.09889466217206,-6.67733201834192));
#68206=CARTESIAN_POINT('Ctrl Pts',(38.0381082199237,-2.09257056471699,-6.63831467392438));
#68207=CARTESIAN_POINT('Ctrl Pts',(38.1288952990446,-2.08624646726192,-6.60340352926506));
#68208=CARTESIAN_POINT('Ctrl Pts',(38.2212188807458,-2.07992236980685,-6.5727943544713));
#68209=CARTESIAN_POINT('Ctrl Pts',(38.3134458272225,-2.0736048917936,-6.54221721834442));
#68210=CARTESIAN_POINT('Ctrl Pts',(38.4072056660689,-2.06728741378035,-6.51593323704319));
#68211=CARTESIAN_POINT('Ctrl Pts',(38.5020627603779,-2.0609699357671,-6.49409019229397));
#68212=CARTESIAN_POINT('Ctrl Pts',(38.596852521998,-2.05465694210776,-6.47226265245712));
#68213=CARTESIAN_POINT('Ctrl Pts',(38.6927375656928,-2.04834394844841,-6.45486988002064));
#68214=CARTESIAN_POINT('Ctrl Pts',(38.7892678275694,-2.04203095478907,-6.44200961152481));
#68215=CARTESIAN_POINT('Ctrl Pts',(38.8857632063168,-2.03572024245548,-6.42915399034266));
#68216=CARTESIAN_POINT('Ctrl Pts',(38.9829029069063,-2.02940953012189,-6.42082767624792));
#68217=CARTESIAN_POINT('Ctrl Pts',(39.0802283551054,-2.02309881778831,-6.41707699484379));
#68218=CARTESIAN_POINT('Ctrl Pts',(39.1775449935443,-2.01678867669137,-6.41332665294597));
#68219=CARTESIAN_POINT('Ctrl Pts',(39.2750469091687,-2.01047853559443,-6.41415113688605));
#68220=CARTESIAN_POINT('Ctrl Pts',(39.3722731621719,-2.00416839449749,-6.41954470157832));
#68221=CARTESIAN_POINT('Ctrl Pts',(39.4695169478507,-1.99785711550154,-6.42493923888464));
#68222=CARTESIAN_POINT('Ctrl Pts',(39.5664845355442,-1.99154583650559,-6.43490446912655));
#68223=CARTESIAN_POINT('Ctrl Pts',(39.6627187994011,-1.98523455750964,-6.44938266918967));
#68224=CARTESIAN_POINT('Ctrl Pts',(39.7590559793581,-1.97891652902349,-6.46387635271813));
#68225=CARTESIAN_POINT('Ctrl Pts',(39.8546578366261,-1.97259850053733,-6.48289257638167));
#68226=CARTESIAN_POINT('Ctrl Pts',(39.9490763553248,-1.96628047205118,-6.50632226516421));
#68227=CARTESIAN_POINT('Ctrl Pts',(40.0435502002251,-1.95995874140444,-6.52976568298745));
#68228=CARTESIAN_POINT('Ctrl Pts',(40.1368389069724,-1.95363701075771,-6.55762759056469));
#68229=CARTESIAN_POINT('Ctrl Pts',(40.2285105838422,-1.94731528011097,-6.58974930681813));
#68230=CARTESIAN_POINT('Ctrl Pts',(40.3203292495694,-1.94098341302955,-6.62192252790419));
#68231=CARTESIAN_POINT('Ctrl Pts',(40.4105253028673,-1.93465154594813,-6.65836903282714));
#68232=CARTESIAN_POINT('Ctrl Pts',(40.4986877933102,-1.92831967886671,-6.69888240364859));
#68233=CARTESIAN_POINT('Ctrl Pts',(40.5498940181504,-1.92464202629813,-6.72241323592088));
#68234=CARTESIAN_POINT('Ctrl Pts',(40.6004146859581,-1.92096437372955,-6.74731515466951));
#68235=CARTESIAN_POINT('Ctrl Pts',(40.6501736040664,-1.91728672116097,-6.77354090145443));
#68236=CARTESIAN_POINT('Ctrl Pts',(40.7358544348572,-1.91095410101134,-6.81869951538878));
#68237=CARTESIAN_POINT('Ctrl Pts',(40.8195727132583,-1.90462148086172,-6.86794254904839));
#68238=CARTESIAN_POINT('Ctrl Pts',(40.9009135302045,-1.89828886071209,-6.92107530530023));
#68239=CARTESIAN_POINT('Ctrl Pts',(40.982144875412,-1.89196476325703,-6.97413655335452));
#68240=CARTESIAN_POINT('Ctrl Pts',(41.0610047556517,-1.88564066580197,-7.0310768821671));
#68241=CARTESIAN_POINT('Ctrl Pts',(41.1371021272715,-1.87931656834691,-7.09165538786217));
#68242=CARTESIAN_POINT('Ctrl Pts',(41.2131198476639,-1.87299909033367,-7.15217048594894));
#68243=CARTESIAN_POINT('Ctrl Pts',(41.2863804675783,-1.86668161232043,-7.21631591932709));
#68244=CARTESIAN_POINT('Ctrl Pts',(41.3565221099628,-1.86036413430719,-7.28380767399548));
#68245=CARTESIAN_POINT('Ctrl Pts',(41.4266139635002,-1.85405114064785,-7.35125152079422));
#68246=CARTESIAN_POINT('Ctrl Pts',(41.49359092675,-1.84773814698851,-7.42203666422981));
#68247=CARTESIAN_POINT('Ctrl Pts',(41.5571251435103,-1.84142515332918,-7.49583965376528));
#68248=CARTESIAN_POINT('Ctrl Pts',(41.6206364009184,-1.8351144409956,-7.5696159731233));
#68249=CARTESIAN_POINT('Ctrl Pts',(41.6807070988664,-1.82880372866201,-7.64640764054255));
#68250=CARTESIAN_POINT('Ctrl Pts',(41.7370477798076,-1.82249301632844,-7.72585597689531));
#68251=CARTESIAN_POINT('Ctrl Pts',(41.793383360871,-1.8161828752315,-7.8052971216984));
#68252=CARTESIAN_POINT('Ctrl Pts',(41.8459893434284,-1.80987273413457,-7.88739410046962));
#68253=CARTESIAN_POINT('Ctrl Pts',(41.8946185798966,-1.80356259303764,-7.97175779037008));
#68254=CARTESIAN_POINT('Ctrl Pts',(41.9432565856077,-1.7972513140417,-8.0561366934579));
#68255=CARTESIAN_POINT('Ctrl Pts',(41.9879162025771,-1.79094003504576,-8.14278274062103));
#68256=CARTESIAN_POINT('Ctrl Pts',(42.0283958934414,-1.78462875604982,-8.23128159058329));
#68257=CARTESIAN_POINT('Ctrl Pts',(42.0689188746241,-1.77831072756368,-8.31987508413867));
#68258=CARTESIAN_POINT('Ctrl Pts',(42.1052528230875,-1.77199269907753,-8.41032493800567));
#68259=CARTESIAN_POINT('Ctrl Pts',(42.1372441822829,-1.76567467059138,-8.5021963695092));
#68260=CARTESIAN_POINT('Ctrl Pts',(42.1692542873814,-1.75935293994465,-8.59412163470362));
#68261=CARTESIAN_POINT('Ctrl Pts',(42.1969166119891,-1.75303120929792,-8.6874697171569));
#68262=CARTESIAN_POINT('Ctrl Pts',(42.2201279525242,-1.74670947865119,-8.78179222065277));
#68263=CARTESIAN_POINT('Ctrl Pts',(42.2433765107533,-1.74037761156977,-8.87626596341354));
#68264=CARTESIAN_POINT('Ctrl Pts',(42.2621597495313,-1.73404574448836,-8.97171681826881));
#68265=CARTESIAN_POINT('Ctrl Pts',(42.27642588615,-1.72771387740694,-9.06768783098812));
#68266=CARTESIAN_POINT('Ctrl Pts',(42.2847118929953,-1.72403622483829,-9.12342937402826));
#68267=CARTESIAN_POINT('Ctrl Pts',(42.2914750389586,-1.72035857226964,-9.17934630607834));
#68268=CARTESIAN_POINT('Ctrl Pts',(42.2967132490314,-1.71668091970099,-9.23534899245219));
#68269=CARTESIAN_POINT('Ctrl Pts',(42.3057330229322,-1.71034829955137,-9.33178108698647));
#68270=CARTESIAN_POINT('Ctrl Pts',(42.3102598110864,-1.70401567940174,-9.42880239748814));
#68271=CARTESIAN_POINT('Ctrl Pts',(42.3102298521332,-1.69768305925211,-9.52595906164897));
#68272=CARTESIAN_POINT('Ctrl Pts',(42.3101999335,-1.69135896179705,-9.62298496846862));
#68273=CARTESIAN_POINT('Ctrl Pts',(42.3056254568274,-1.68503486434198,-9.72014543326724));
#68274=CARTESIAN_POINT('Ctrl Pts',(42.296494398712,-1.67871076688692,-9.81698132071288));
#68275=CARTESIAN_POINT('Ctrl Pts',(42.2873728980881,-1.67239328887368,-9.91371584989706));
#68276=CARTESIAN_POINT('Ctrl Pts',(42.2737043386173,-1.66607581086044,-10.0101260440443));
#68277=CARTESIAN_POINT('Ctrl Pts',(42.2555287395324,-1.65975833284719,-10.1057536265848));
#68278=CARTESIAN_POINT('Ctrl Pts',(42.2373660420863,-1.65344533918785,-10.2013133295186));
#68279=CARTESIAN_POINT('Ctrl Pts',(42.2147027467418,-1.64713234552851,-10.2960910968563));
#68280=CARTESIAN_POINT('Ctrl Pts',(42.1876304925971,-1.64081935186917,-10.3896355837021));
#68281=CARTESIAN_POINT('Ctrl Pts',(42.1605680215496,-1.63450863953558,-10.483146266388));
#68282=CARTESIAN_POINT('Ctrl Pts',(42.1290998789849,-1.628197927202,-10.5754241344851));
#68283=CARTESIAN_POINT('Ctrl Pts',(42.0933681932019,-1.62188721486841,-10.6660307408074));
#68284=CARTESIAN_POINT('Ctrl Pts',(42.0576397418,-1.61557707377148,-10.7566291455495));
#68285=CARTESIAN_POINT('Ctrl Pts',(42.0176486751247,-1.60926693267455,-10.8455561825538));
#68286=CARTESIAN_POINT('Ctrl Pts',(41.9735857419016,-1.60295679157761,-10.9323921931075));
#68287=CARTESIAN_POINT('Ctrl Pts',(41.9295148628708,-1.59664551258167,-11.0192438626788));
#68288=CARTESIAN_POINT('Ctrl Pts',(41.8813708568461,-1.59033423358572,-11.1040033669291));
#68289=CARTESIAN_POINT('Ctrl Pts',(41.829390521414,-1.58402295458978,-11.1862754554251));
#68290=CARTESIAN_POINT('Ctrl Pts',(41.7773545964945,-1.57770492610363,-11.2686355284099));
#68291=CARTESIAN_POINT('Ctrl Pts',(41.7214743853249,-1.57138689761748,-11.3485025045336));
#68292=CARTESIAN_POINT('Ctrl Pts',(41.6620300299614,-1.56506886913133,-11.4255101379547));
#68293=CARTESIAN_POINT('Ctrl Pts',(41.602550842126,-1.5587471384846,-11.5025628953611));
#68294=CARTESIAN_POINT('Ctrl Pts',(41.5395036344395,-1.55242540783787,-11.5767526406318));
#68295=CARTESIAN_POINT('Ctrl Pts',(41.4732074725687,-1.54610367719113,-11.647747851149));
#68296=CARTESIAN_POINT('Ctrl Pts',(41.4068050096307,-1.53977181010971,-11.7188568973157));
#68297=CARTESIAN_POINT('Ctrl Pts',(41.3371435030825,-1.5334399430283,-11.7867608755279));
#68298=CARTESIAN_POINT('Ctrl Pts',(41.2645772925355,-1.52710807594688,-11.8511666440836));
#68299=CARTESIAN_POINT('Ctrl Pts',(41.2224296436379,-1.52343042337825,-11.8885745740223));
#68300=CARTESIAN_POINT('Ctrl Pts',(41.1793027026836,-1.51975277080963,-11.924803159381));
#68301=CARTESIAN_POINT('Ctrl Pts',(41.1352703938616,-1.51607511824101,-11.9598016665722));
#68302=CARTESIAN_POINT('Ctrl Pts',(41.0594503208998,-1.50974249809138,-12.0200662640866));
#68303=CARTESIAN_POINT('Ctrl Pts',(40.9806808984483,-1.50340987794174,-12.0768905950471));
#68304=CARTESIAN_POINT('Ctrl Pts',(40.8993073292417,-1.49707725779211,-12.1299731771528));
#68305=CARTESIAN_POINT('Ctrl Pts',(40.8180432758533,-1.49075316033705,-12.1829843185872));
#68306=CARTESIAN_POINT('Ctrl Pts',(40.7341824047728,-1.48442906288198,-12.232263483133));
#68307=CARTESIAN_POINT('Ctrl Pts',(40.6481026152132,-1.47810496542692,-12.2775496305631));
#68308=CARTESIAN_POINT('Ctrl Pts',(40.5621129254919,-1.47178748741368,-12.3227883769181));
#68309=CARTESIAN_POINT('Ctrl Pts',(40.4739093196116,-1.46547000940043,-12.3640422126576));
#68310=CARTESIAN_POINT('Ctrl Pts',(40.3838974251622,-1.45915253138719,-12.4010941465109));
#68311=CARTESIAN_POINT('Ctrl Pts',(40.2939494241192,-1.45283953772784,-12.4381197796817));
#68312=CARTESIAN_POINT('Ctrl Pts',(40.202196089592,-1.4465265440685,-12.4709492746601));
#68313=CARTESIAN_POINT('Ctrl Pts',(40.1090654611092,-1.44021355040915,-12.4994126546796));
#68314=CARTESIAN_POINT('Ctrl Pts',(40.0159684872305,-1.43390283807557,-12.5278657488909));
#68315=CARTESIAN_POINT('Ctrl Pts',(39.9214956261486,-1.42759212574198,-12.5519557355248));
#68316=CARTESIAN_POINT('Ctrl Pts',(39.8260917154402,-1.4212814134084,-12.5715619666695));
#68317=CARTESIAN_POINT('Ctrl Pts',(39.7306964405573,-1.41497127231146,-12.5911664230862));
#68318=CARTESIAN_POINT('Ctrl Pts',(39.6343707120116,-1.40866113121453,-12.6062878431363));
#68319=CARTESIAN_POINT('Ctrl Pts',(39.5375702111042,-1.40235099011759,-12.6168565628882));
#68320=CARTESIAN_POINT('Ctrl Pts',(39.4407522542966,-1.39603971112165,-12.6274271884827));
#68321=CARTESIAN_POINT('Ctrl Pts',(39.3434597898127,-1.38972843212572,-12.6334434357768));
#68322=CARTESIAN_POINT('Ctrl Pts',(39.2461532310898,-1.38341715312978,-12.6348875433301));
#68323=CARTESIAN_POINT('Ctrl Pts',(39.1487426095192,-1.37709912464362,-12.6363331952598));
#68324=CARTESIAN_POINT('Ctrl Pts',(39.0513183016025,-1.37078109615747,-12.6331969391355));
#68325=CARTESIAN_POINT('Ctrl Pts',(38.9543401257753,-1.36446306767132,-12.6255131638321));
#68326=CARTESIAN_POINT('Ctrl Pts',(38.85730512387,-1.35814133702458,-12.6178248860845));
#68327=CARTESIAN_POINT('Ctrl Pts',(38.7607172082617,-1.35181960637785,-12.6055838379726));
#68328=CARTESIAN_POINT('Ctrl Pts',(38.6650283971823,-1.34549787573111,-12.5888759826531));
#68329=CARTESIAN_POINT('Ctrl Pts',(38.5691861560632,-1.33916600864969,-12.5721413375045));
#68330=CARTESIAN_POINT('Ctrl Pts',(38.4742463247096,-1.33283414156828,-12.5509256788029));
#68331=CARTESIAN_POINT('Ctrl Pts',(38.3806480632887,-1.32650227448686,-12.5253654871878));
#68332=CARTESIAN_POINT('Ctrl Pts',(38.3262846532383,-1.32282462191824,-12.5105197073982));
#68333=CARTESIAN_POINT('Ctrl Pts',(38.2723735049704,-1.31914696934963,-12.4942092345176));
#68334=CARTESIAN_POINT('Ctrl Pts',(38.2189975102117,-1.31546931678102,-12.4764682393563));
#68335=CARTESIAN_POINT('Ctrl Pts',(38.1270883661017,-1.30913669663139,-12.4459196811832));
#68336=CARTESIAN_POINT('Ctrl Pts',(38.0364478673732,-1.30280407648177,-12.4110208775835));
#68337=CARTESIAN_POINT('Ctrl Pts',(37.9475171640674,-1.29647145633214,-12.3718960990163));
#68338=CARTESIAN_POINT('Ctrl Pts',(37.8587061472744,-1.29014735887709,-12.3328239761477));
#68339=CARTESIAN_POINT('Ctrl Pts',(37.7716007492447,-1.28382326142203,-12.2895373570747));
#68340=CARTESIAN_POINT('Ctrl Pts',(37.6866261270882,-1.27749916396698,-12.242209998084));
#68341=CARTESIAN_POINT('Ctrl Pts',(37.6017404479898,-1.27118168595374,-12.1949321767075));
#68342=CARTESIAN_POINT('Ctrl Pts',(37.518981490894,-1.2648642079405,-12.1436222354299));
#68343=CARTESIAN_POINT('Ctrl Pts',(37.4387526839846,-1.25854672992727,-12.0885012277603));
#68344=CARTESIAN_POINT('Ctrl Pts',(37.3585808261239,-1.25223373626793,-12.0334193467969));
#68345=CARTESIAN_POINT('Ctrl Pts',(37.2809359073443,-1.2459207426086,-11.9745320245189));
#68346=CARTESIAN_POINT('Ctrl Pts',(37.2061942375429,-1.23960774894926,-11.9121047807947));
#68347=CARTESIAN_POINT('Ctrl Pts',(37.1314795771296,-1.23329703661568,-11.849700096396));
#68348=CARTESIAN_POINT('Ctrl Pts',(37.0596664163264,-1.2269863242821,-11.7837583124312));
#68349=CARTESIAN_POINT('Ctrl Pts',(36.9910989400906,-1.22067561194852,-11.7145859792279));
#68350=CARTESIAN_POINT('Ctrl Pts',(36.9225376704846,-1.21436547085158,-11.6454199074051));
#68351=CARTESIAN_POINT('Ctrl Pts',(36.8572218090311,-1.20805532975465,-11.5730241784787));
#68352=CARTESIAN_POINT('Ctrl Pts',(36.7954587750304,-1.20174518865771,-11.497742291918));
#68353=CARTESIAN_POINT('Ctrl Pts',(36.7336846033874,-1.19543390966177,-11.4224468298789));
#68354=CARTESIAN_POINT('Ctrl Pts',(36.6754648090073,-1.18912263066584,-11.3442645146203));
#68355=CARTESIAN_POINT('Ctrl Pts',(36.6210659356797,-1.1828113516699,-11.2635711790975));
#68356=CARTESIAN_POINT('Ctrl Pts',(36.5666088864003,-1.17649332318375,-11.1827915474565));
#68357=CARTESIAN_POINT('Ctrl Pts',(36.5159811609401,-1.17017529469761,-11.0994958975688));
#68358=CARTESIAN_POINT('Ctrl Pts',(36.4694053081403,-1.16385726621147,-11.014088070494));
#68359=CARTESIAN_POINT('Ctrl Pts',(36.4228021633954,-1.15753553556474,-10.9286301971917));
#68360=CARTESIAN_POINT('Ctrl Pts',(36.3802558101443,-1.15121380491802,-10.8410580753411));
#68361=CARTESIAN_POINT('Ctrl Pts',(36.3419413461397,-1.14489207427129,-10.751797205733));
#68362=CARTESIAN_POINT('Ctrl Pts',(36.3035654476824,-1.13856020718988,-10.6623932128213));
#68363=CARTESIAN_POINT('Ctrl Pts',(36.2694351413073,-1.13222834010846,-10.5712954744392));
#68364=CARTESIAN_POINT('Ctrl Pts',(36.2396761939009,-1.12589647302705,-10.4789463380835));
#68365=CARTESIAN_POINT('Ctrl Pts',(36.2223917076723,-1.12221882045838,-10.4253084404198));
#68366=CARTESIAN_POINT('Ctrl Pts',(36.2065809431792,-1.11854116788971,-10.3712486294749));
#68367=CARTESIAN_POINT('Ctrl Pts',(36.1922605966023,-1.11486351532104,-10.3168549956581));
#68368=CARTESIAN_POINT('Ctrl Pts',(36.160600384436,-1.10673275815172,-10.1965985494974));
#68369=CARTESIAN_POINT('Ctrl Pts',(36.1361386046844,-1.0986020009824,-10.0743742818528));
#68370=CARTESIAN_POINT('Ctrl Pts',(36.1190733990765,-1.09047124381308,-9.95093653590859));
#68371=CARTESIAN_POINT('Ctrl Pts',(36.1023366837152,-1.08249699659095,-9.82987485835468));
#68372=CARTESIAN_POINT('Ctrl Pts',(36.0927145179575,-1.07452274936882,-9.70764575813965));
#68373=CARTESIAN_POINT('Ctrl Pts',(36.0903484504941,-1.06654850214669,-9.58498244372551));
#68374=CARTESIAN_POINT('Ctrl Pts',(36.0899806582649,-1.06530894908788,-9.56591510327944));
#68375=CARTESIAN_POINT('Ctrl Pts',(36.0897881039816,-1.06406939602907,-9.54683731773078));
#68376=CARTESIAN_POINT('Ctrl Pts',(36.0897712174216,-1.06282984297026,-9.52775189410163));
#68377=CARTESIAN_POINT('',(36.0899362460626,0.207170205182039,-9.52357073843679));
#68378=CARTESIAN_POINT('Ctrl Pts',(36.0897712174209,-1.06282984291314,-9.52775189322205));
#68379=CARTESIAN_POINT('Ctrl Pts',(36.0896860844236,-1.05658067781646,-9.43153337126958));
#68380=CARTESIAN_POINT('Ctrl Pts',(36.0940701443256,-1.05033151271977,-9.3352083438086));
#68381=CARTESIAN_POINT('Ctrl Pts',(36.1029262969847,-1.04408234762309,-9.23922888356096));
#68382=CARTESIAN_POINT('Ctrl Pts',(36.1117776524504,-1.03783656756891,-9.14330141338673));
#68383=CARTESIAN_POINT('Ctrl Pts',(36.1250962497593,-1.03159078751473,-9.04771958335936));
#68384=CARTESIAN_POINT('Ctrl Pts',(36.1428329414513,-1.02534500746055,-8.95293337011782));
#68385=CARTESIAN_POINT('Ctrl Pts',(36.1605650823694,-1.01910082991111,-8.85817147655383));
#68386=CARTESIAN_POINT('Ctrl Pts',(36.1827129836568,-1.01285665236168,-8.76420523396972));
#68387=CARTESIAN_POINT('Ctrl Pts',(36.2091760613553,-1.00661247481225,-8.67147623294382));
#68388=CARTESIAN_POINT('Ctrl Pts',(36.2356398940563,-1.00036811911387,-8.57874458632138));
#68389=CARTESIAN_POINT('Ctrl Pts',(36.2664190235894,-0.994123763415482,
-8.48725068141378));
#68390=CARTESIAN_POINT('Ctrl Pts',(36.3013628189955,-0.987879407717097,
-8.39742155669849));
#68391=CARTESIAN_POINT('Ctrl Pts',(36.336340477737,-0.981629000738119,-8.30750538036965));
#68392=CARTESIAN_POINT('Ctrl Pts',(36.3754907006624,-0.975378593759137,
-8.2192576245062));
#68393=CARTESIAN_POINT('Ctrl Pts',(36.4186145503963,-0.969128186780159,
-8.13308562273654));
#68394=CARTESIAN_POINT('Ctrl Pts',(36.4617589066273,-0.96287480757228,-8.04687264396891));
#68395=CARTESIAN_POINT('Ctrl Pts',(36.5088804328319,-0.956621428364402,
-7.96273777518549));
#68396=CARTESIAN_POINT('Ctrl Pts',(36.559735136623,-0.950368049156523,-7.88106201329952));
#68397=CARTESIAN_POINT('Ctrl Pts',(36.6106765485517,-0.944104007830401,
-7.79924699284601));
#68398=CARTESIAN_POINT('Ctrl Pts',(36.6653635991613,-0.937839966504279,
-7.71989982409718));
#68399=CARTESIAN_POINT('Ctrl Pts',(36.7235100063757,-0.931575925178158,
-7.64337092805759));
#68400=CARTESIAN_POINT('Ctrl Pts',(36.7770958473711,-0.925803188072458,
-7.57284438220232));
#68401=CARTESIAN_POINT('Ctrl Pts',(36.8336190328546,-0.92003045096676,-7.50471118571648));
#68402=CARTESIAN_POINT('Ctrl Pts',(36.8928280636448,-0.914257713861061,
-7.43921757870213));
#68403=CARTESIAN_POINT('Ctrl Pts',(36.9577796272717,-0.907925093711437,
-7.36737191383699));
#68404=CARTESIAN_POINT('Ctrl Pts',(37.0262031313875,-0.901592473561813,
-7.29843824581509));
#68405=CARTESIAN_POINT('Ctrl Pts',(37.0978072860804,-0.895259853412189,
-7.23277042021453));
#68406=CARTESIAN_POINT('Ctrl Pts',(37.169315073026,-0.888935755957113,-7.16719097301123));
#68407=CARTESIAN_POINT('Ctrl Pts',(37.2439946829859,-0.882611658502038,
-7.10486892544389));
#68408=CARTESIAN_POINT('Ctrl Pts',(37.3215159596994,-0.876287561046962,
-7.04612356838108));
#68409=CARTESIAN_POINT('Ctrl Pts',(37.3989560947817,-0.869970083033735,
-6.9874397001675));
#68410=CARTESIAN_POINT('Ctrl Pts',(37.4792316367028,-0.863652605020507,
-6.93232534248509));
#68411=CARTESIAN_POINT('Ctrl Pts',(37.561977874681,-0.85733512700728,-6.88106086116467));
#68412=CARTESIAN_POINT('Ctrl Pts',(37.6446653766551,-0.851022133347939,
-6.82983276906089));
#68413=CARTESIAN_POINT('Ctrl Pts',(37.729819717368,-0.844709139688599,-6.78244935007139));
#68414=CARTESIAN_POINT('Ctrl Pts',(37.8170463918134,-0.838396146029258,
-6.73914825044412));
#68415=CARTESIAN_POINT('Ctrl Pts',(37.9042415451658,-0.83208543369568,-6.69586279853004));
#68416=CARTESIAN_POINT('Ctrl Pts',(37.9935071529134,-0.825774721362104,
-6.6566569289384));
#68417=CARTESIAN_POINT('Ctrl Pts',(38.0844240759997,-0.819464009028525,
-6.62172236761779));
#68418=CARTESIAN_POINT('Ctrl Pts',(38.1753327694161,-0.813153867931602,
-6.5867909685237));
#68419=CARTESIAN_POINT('Ctrl Pts',(38.2678920726935,-0.806843726834677,
-6.55613026564564));
#68420=CARTESIAN_POINT('Ctrl Pts',(38.3616638164926,-0.800533585737753,
-6.529883458641));
#68421=CARTESIAN_POINT('Ctrl Pts',(38.4554524700205,-0.794222306741826,
-6.50363191858602));
#68422=CARTESIAN_POINT('Ctrl Pts',(38.5504535771808,-0.7879110277459,-6.48179597310336));
#68423=CARTESIAN_POINT('Ctrl Pts',(38.646215817656,-0.781599748749973,-6.46446839057565));
#68424=CARTESIAN_POINT('Ctrl Pts',(38.7420804694343,-0.775281720263821,
-6.44712227735884));
#68425=CARTESIAN_POINT('Ctrl Pts',(38.8387074485619,-0.76896369177767,-6.43429423073547));
#68426=CARTESIAN_POINT('Ctrl Pts',(38.9356374987543,-0.762645663291519,
-6.42602547270309));
#68427=CARTESIAN_POINT('Ctrl Pts',(39.0326243468245,-0.756323932644797,
-6.41775186944565));
#68428=CARTESIAN_POINT('Ctrl Pts',(39.1299141827867,-0.750002201998074,
-6.4140428913081));
#68429=CARTESIAN_POINT('Ctrl Pts',(39.227047016857,-0.743680471351352,-6.41488760463884));
#68430=CARTESIAN_POINT('Ctrl Pts',(39.3243355963527,-0.737348604269936,
-6.41573367240589));
#68431=CARTESIAN_POINT('Ctrl Pts',(39.4214662349143,-0.731016737188519,
-6.42114798715704));
#68432=CARTESIAN_POINT('Ctrl Pts',(39.5179833718286,-0.724684870107102,
-6.431067675572));
#68433=CARTESIAN_POINT('Ctrl Pts',(39.5740421127861,-0.721007217538426,
-6.43682919379571));
#68434=CARTESIAN_POINT('Ctrl Pts',(39.6298940487152,-0.71732956496975,-6.44410962552948));
#68435=CARTESIAN_POINT('Ctrl Pts',(39.6854518178217,-0.713651912401074,
-6.45288880646003));
#68436=CARTESIAN_POINT('Ctrl Pts',(39.7811178008206,-0.707319292251471,
-6.4680058456636));
#68437=CARTESIAN_POINT('Ctrl Pts',(39.8762431598389,-0.700986672101865,
-6.48762197611831));
#68438=CARTESIAN_POINT('Ctrl Pts',(39.970372366564,-0.694654051952262,-6.51168669572269));
#68439=CARTESIAN_POINT('Ctrl Pts',(40.0643748904216,-0.688329954497225,
-6.53571902806079));
#68440=CARTESIAN_POINT('Ctrl Pts',(40.1573835065057,-0.682005857042191,
-6.56418794252481));
#68441=CARTESIAN_POINT('Ctrl Pts',(40.2489503768969,-0.675681759587154,
-6.59699150279447));
#68442=CARTESIAN_POINT('Ctrl Pts',(40.3404214041147,-0.669364281573921,
-6.62976072753093));
#68443=CARTESIAN_POINT('Ctrl Pts',(40.4304532762286,-0.66304680356069,-6.6668554314271));
#68444=CARTESIAN_POINT('Ctrl Pts',(40.5186118622718,-0.656729325547457,
-6.7081234656847));
#68445=CARTESIAN_POINT('Ctrl Pts',(40.6067078704477,-0.650416331888136,
-6.74936220653274));
#68446=CARTESIAN_POINT('Ctrl Pts',(40.692932841173,-0.644103338228813,-6.79476820350162));
#68447=CARTESIAN_POINT('Ctrl Pts',(40.7768721299827,-0.637790344569493,
-6.84414100732919));
#68448=CARTESIAN_POINT('Ctrl Pts',(40.8607810856617,-0.631479632235927,
-6.89349596931263));
#68449=CARTESIAN_POINT('Ctrl Pts',(40.9424056240902,-0.62516891990236,-6.94681466831479));
#68450=CARTESIAN_POINT('Ctrl Pts',(41.0213560881748,-0.618858207568794,
-7.0038509260719));
#68451=CARTESIAN_POINT('Ctrl Pts',(41.1002994057763,-0.612548066471879,
-7.06088202098856));
#68452=CARTESIAN_POINT('Ctrl Pts',(41.17656877593,-0.606237925374965,-7.12162974934534));
#68453=CARTESIAN_POINT('Ctrl Pts',(41.2498047742485,-0.59992778427805,-7.18580547188391));
#68454=CARTESIAN_POINT('Ctrl Pts',(41.3230539791133,-0.593616505282114,
-7.24999276714181));
#68455=CARTESIAN_POINT('Ctrl Pts',(41.3932683968505,-0.587305226286178,
-7.31760899610106));
#68456=CARTESIAN_POINT('Ctrl Pts',(41.4601236447158,-0.580993947290242,
-7.38832694042902));
#68457=CARTESIAN_POINT('Ctrl Pts',(41.5270503897912,-0.574675918804115,
-7.45912051286214));
#68458=CARTESIAN_POINT('Ctrl Pts',(41.5906104920292,-0.568357890317988,
-7.53302210471867));
#68459=CARTESIAN_POINT('Ctrl Pts',(41.6505183947253,-0.56203986183186,-7.60966967600554));
#68460=CARTESIAN_POINT('Ctrl Pts',(41.710461401517,-0.555718131185156,-7.68636216029295));
#68461=CARTESIAN_POINT('Ctrl Pts',(41.7667476945924,-0.549396400538453,
-7.76580347141102));
#68462=CARTESIAN_POINT('Ctrl Pts',(41.8191349904781,-0.543074669891748,
-7.84760244588428));
#68463=CARTESIAN_POINT('Ctrl Pts',(41.8716062855774,-0.53674280281035,-7.92953257905585));
#68464=CARTESIAN_POINT('Ctrl Pts',(41.9201658816691,-0.53041093572895,-8.01382754556607));
#68465=CARTESIAN_POINT('Ctrl Pts',(41.9646174096111,-0.524079068647551,
-8.10007149955682));
#68466=CARTESIAN_POINT('Ctrl Pts',(41.9904355883287,-0.520401416078733,
-8.15016340686659));
#68467=CARTESIAN_POINT('Ctrl Pts',(42.0148688134366,-0.516723763509916,
-8.20091240630828));
#68468=CARTESIAN_POINT('Ctrl Pts',(42.0378862165493,-0.513046110941098,
-8.25223432053687));
#68469=CARTESIAN_POINT('Ctrl Pts',(42.0775203222778,-0.506713490791419,
-8.3406065041737));
#68470=CARTESIAN_POINT('Ctrl Pts',(42.1130914569429,-0.50038087064174,-8.43098526761534));
#68471=CARTESIAN_POINT('Ctrl Pts',(42.1443929096834,-0.49404825049206,-8.5229615544771));
#68472=CARTESIAN_POINT('Ctrl Pts',(42.1756522356715,-0.487724153036946,
-8.61481405595751));
#68473=CARTESIAN_POINT('Ctrl Pts',(42.2026531610915,-0.481400055581832,
-8.70825939711112));
#68474=CARTESIAN_POINT('Ctrl Pts',(42.2252362488598,-0.475075958126719,
-8.80286684643024));
#68475=CARTESIAN_POINT('Ctrl Pts',(42.247795698878,-0.468758480113422,-8.89737526999737));
#68476=CARTESIAN_POINT('Ctrl Pts',(42.2659464032894,-0.462441002100126,
-8.99304296037945));
#68477=CARTESIAN_POINT('Ctrl Pts',(42.2795784644896,-0.456123524086829,
-9.08942321692722));
#68478=CARTESIAN_POINT('Ctrl Pts',(42.2932008492039,-0.449810530427428,
-9.18573505959558));
#68479=CARTESIAN_POINT('Ctrl Pts',(42.3023109063022,-0.443497536768026,
-9.28275803108793));
#68480=CARTESIAN_POINT('Ctrl Pts',(42.3068498357854,-0.437184543108625,
-9.38003534644477));
#68481=CARTESIAN_POINT('Ctrl Pts',(42.3113871250362,-0.430873830774989,
-9.47727750870977));
#68482=CARTESIAN_POINT('Ctrl Pts',(42.311356548589,-0.424563118441352,-9.57477339581393));
#68483=CARTESIAN_POINT('Ctrl Pts',(42.3067512576344,-0.418252406107716,
-9.67206215042368));
#68484=CARTESIAN_POINT('Ctrl Pts',(42.3021463835441,-0.411942265010724,
-9.76934209859467));
#68485=CARTESIAN_POINT('Ctrl Pts',(42.2929676391518,-0.405632123913731,
-9.86641451473711));
#68486=CARTESIAN_POINT('Ctrl Pts',(42.2792602574679,-0.399321982816739,
-9.9628206478441));
#68487=CARTESIAN_POINT('Ctrl Pts',(42.2655504039509,-0.393010703820751,
-10.0592441657354));
#68488=CARTESIAN_POINT('Ctrl Pts',(42.2473103527805,-0.386699424824764,
-10.1550007290107));
#68489=CARTESIAN_POINT('Ctrl Pts',(42.2246367967948,-0.380388145828777,
-10.2496398418352));
#68490=CARTESIAN_POINT('Ctrl Pts',(42.2019389929594,-0.374070117342578,
-10.3443801648528));
#68491=CARTESIAN_POINT('Ctrl Pts',(42.1747983205458,-0.367752088856378,
-10.4380002256121));
#68492=CARTESIAN_POINT('Ctrl Pts',(42.1433618544534,-0.361434060370179,
-10.5300630063079));
#68493=CARTESIAN_POINT('Ctrl Pts',(42.1119069676073,-0.35511232972338,-10.6221797328193));
#68494=CARTESIAN_POINT('Ctrl Pts',(42.0761514351891,-0.348790599076581,
-10.712736955624));
#68495=CARTESIAN_POINT('Ctrl Pts',(42.0362903735297,-0.342468868429782,
-10.8013179736739));
#68496=CARTESIAN_POINT('Ctrl Pts',(41.996365397561,-0.336137001348314,-10.8900410249347));
#68497=CARTESIAN_POINT('Ctrl Pts',(41.9523219452859,-0.329805134266847,
-10.9767811544218));
#68498=CARTESIAN_POINT('Ctrl Pts',(41.9044008992474,-0.323473267185379,
-11.0611466170421));
#68499=CARTESIAN_POINT('Ctrl Pts',(41.8765675673468,-0.319795614617291,
-11.1101474656498));
#68500=CARTESIAN_POINT('Ctrl Pts',(41.8474269568295,-0.316117962049202,
-11.1583477587084));
#68501=CARTESIAN_POINT('Ctrl Pts',(41.8170326830038,-0.312440309481113,
-11.2056756346749));
#68502=CARTESIAN_POINT('Ctrl Pts',(41.7646962027907,-0.30610768933152,-11.2871704076135));
#68503=CARTESIAN_POINT('Ctrl Pts',(41.7084585529873,-0.299775069181927,
-11.3663597582041));
#68504=CARTESIAN_POINT('Ctrl Pts',(41.648549277778,-0.293442449032334,-11.4428469926437));
#68505=CARTESIAN_POINT('Ctrl Pts',(41.5887206308779,-0.287118351577308,
-11.5192312874909));
#68506=CARTESIAN_POINT('Ctrl Pts',(41.5252304472576,-0.280794254122283,
-11.5929203527617));
#68507=CARTESIAN_POINT('Ctrl Pts',(41.4583522621891,-0.274470156667257,
-11.6635452328079));
#68508=CARTESIAN_POINT('Ctrl Pts',(41.391544078612,-0.268152678654027,-11.7340961896918));
#68509=CARTESIAN_POINT('Ctrl Pts',(41.3213552427646,-0.261835200640793,
-11.8015890217252));
#68510=CARTESIAN_POINT('Ctrl Pts',(41.2480997413983,-0.255517722627563,
-11.8656875276688));
#68511=CARTESIAN_POINT('Ctrl Pts',(41.1748962391992,-0.249204728968255,
-11.9297405343821));
#68512=CARTESIAN_POINT('Ctrl Pts',(41.0986307273081,-0.242891735308945,
-11.9904037178899));
#68513=CARTESIAN_POINT('Ctrl Pts',(41.0196535678084,-0.236578741649637,
-12.0473781528673));
#68514=CARTESIAN_POINT('Ctrl Pts',(40.9407049482752,-0.230268029316084,
-12.1043319990001));
#68515=CARTESIAN_POINT('Ctrl Pts',(40.8590469825193,-0.223957316982531,
-12.1575994897006));
#68516=CARTESIAN_POINT('Ctrl Pts',(40.7750618402567,-0.217646604648978,
-12.2069229765725));
#68517=CARTESIAN_POINT('Ctrl Pts',(40.6910843002089,-0.211336463552075,
-12.2562419987529));
#68518=CARTESIAN_POINT('Ctrl Pts',(40.6047803796756,-0.205026322455174,
-12.3016175056337));
#68519=CARTESIAN_POINT('Ctrl Pts',(40.5165589534812,-0.198716181358271,
-12.342836612529));
#68520=CARTESIAN_POINT('Ctrl Pts',(40.4283216184387,-0.192404902362335,
-12.3840631524088));
#68521=CARTESIAN_POINT('Ctrl Pts',(40.338166487181,-0.1860936233664,-12.4211316185863));
#68522=CARTESIAN_POINT('Ctrl Pts',(40.2465236507183,-0.179782344370464,
-12.4538767303161));
#68523=CARTESIAN_POINT('Ctrl Pts',(40.15478280838,-0.173464315884345,-12.4866568607498));
#68524=CARTESIAN_POINT('Ctrl Pts',(40.0615514969825,-0.167146287398224,
-12.5151042587068));
#68525=CARTESIAN_POINT('Ctrl Pts',(39.967276061071,-0.160828258912105,-12.5391031997938));
#68526=CARTESIAN_POINT('Ctrl Pts',(39.8729453827998,-0.154506528265406,
-12.563116203485));
#68527=CARTESIAN_POINT('Ctrl Pts',(39.7775697899156,-0.148184797618707,
-12.5826754719348));
#68528=CARTESIAN_POINT('Ctrl Pts',(39.6816048744415,-0.141863066972008,
-12.5977166152794));
#68529=CARTESIAN_POINT('Ctrl Pts',(39.5854860862143,-0.135531199890615,
-12.6127818760019));
#68530=CARTESIAN_POINT('Ctrl Pts',(39.488776522994,-0.129199332809222,-12.6233144983368));
#68531=CARTESIAN_POINT('Ctrl Pts',(39.3919358958253,-0.122867465727829,
-12.6293020575958));
#68532=CARTESIAN_POINT('Ctrl Pts',(39.3356892664025,-0.119189813158928,
-12.6327797305172));
#68533=CARTESIAN_POINT('Ctrl Pts',(39.2793984241823,-0.115512160590027,
-12.634725113714));
#68534=CARTESIAN_POINT('Ctrl Pts',(39.2231528518321,-0.111834508021126,
-12.6351438227761));
#68535=CARTESIAN_POINT('Ctrl Pts',(39.126302527308,-0.105501887871624,-12.6358648059014));
#68536=CARTESIAN_POINT('Ctrl Pts',(39.0292502677637,-0.0991692677221215,
-12.6320588343527));
#68537=CARTESIAN_POINT('Ctrl Pts',(38.9324537304411,-0.0928366475726188,
-12.6237012838519));
#68538=CARTESIAN_POINT('Ctrl Pts',(38.8357874657868,-0.0865125501176967,
-12.6153549812782));
#68539=CARTESIAN_POINT('Ctrl Pts',(38.7393766713302,-0.080188452662775,
-12.6024693121629));
#68540=CARTESIAN_POINT('Ctrl Pts',(38.6436798232554,-0.0738643552078528,
-12.5850716517505));
#68541=CARTESIAN_POINT('Ctrl Pts',(38.5480831412077,-0.067546877194739,
-12.567692201494));
#68542=CARTESIAN_POINT('Ctrl Pts',(38.4531993478962,-0.0612293991816249,
-12.5458102267209));
#68543=CARTESIAN_POINT('Ctrl Pts',(38.3594816031123,-0.054911921168511,
-12.5195048801752));
#68544=CARTESIAN_POINT('Ctrl Pts',(38.2658303822694,-0.0485989275093033,
-12.4932182060307));
#68545=CARTESIAN_POINT('Ctrl Pts',(38.1733439842851,-0.0422859338500956,
-12.4625145201786));
#68546=CARTESIAN_POINT('Ctrl Pts',(38.0824642382336,-0.0359729401908879,
-12.4275238111122));
#68547=CARTESIAN_POINT('Ctrl Pts',(37.991617333385,-0.0296622278574401,
-12.3925457466342));
#68548=CARTESIAN_POINT('Ctrl Pts',(37.9023763345141,-0.0233515155239927,
-12.3532838941925));
#68549=CARTESIAN_POINT('Ctrl Pts',(37.8151658928123,-0.0170408031905449,
-12.3099174401532));
#68550=CARTESIAN_POINT('Ctrl Pts',(37.7279633452747,-0.0107306620937389,
-12.2665549115832));
#68551=CARTESIAN_POINT('Ctrl Pts',(37.6427913809412,-0.00442052099693118,
-12.2190887150281));
#68552=CARTESIAN_POINT('Ctrl Pts',(37.5600517642171,0.00188962009987481,
-12.1677448679077));
#68553=CARTESIAN_POINT('Ctrl Pts',(37.4772972271731,0.00820089909564809,
-12.1163917620229));
#68554=CARTESIAN_POINT('Ctrl Pts',(37.3969762804557,0.014512178091419,-12.0611598473829));
#68555=CARTESIAN_POINT('Ctrl Pts',(37.3194624229793,0.0208234570871921,
-12.0023189286632));
#68556=CARTESIAN_POINT('Ctrl Pts',(37.2418656696231,0.0271414855732131,
-11.9434150835213));
#68557=CARTESIAN_POINT('Ctrl Pts',(37.1670823477209,0.0334595140592348,
-11.8808947936913));
#68558=CARTESIAN_POINT('Ctrl Pts',(37.0954533431046,0.0397775425452558,
-11.8150685626964));
#68559=CARTESIAN_POINT('Ctrl Pts',(37.0237823662056,0.0460992731918534,
-11.7492037596568));
#68560=CARTESIAN_POINT('Ctrl Pts',(36.9552696947197,0.0524210038384517,
-11.6800294685806));
#68561=CARTESIAN_POINT('Ctrl Pts',(36.8902182827396,0.0587427344850493,
-11.6078919970823));
#68562=CARTESIAN_POINT('Ctrl Pts',(36.825062565558,0.0650746015663302,-11.5356388584022));
#68563=CARTESIAN_POINT('Ctrl Pts',(36.7633794671254,0.0714064686476086,
-11.4604133898497));
#68564=CARTESIAN_POINT('Ctrl Pts',(36.7054306783924,0.0777383357288892,
-11.3825937533794));
#68565=CARTESIAN_POINT('Ctrl Pts',(36.6717730685476,0.0814159882988748,
-11.337394828262));
#68566=CARTESIAN_POINT('Ctrl Pts',(36.6393744022191,0.0850936408688613,
-11.2913213016371));
#68567=CARTESIAN_POINT('Ctrl Pts',(36.6082788899335,0.0887712934388469,
-11.2444511742227));
#68568=CARTESIAN_POINT('Ctrl Pts',(36.553808851527,0.0952134409389027,-11.1623487275114));
#68569=CARTESIAN_POINT('Ctrl Pts',(36.5031554741128,0.101655588438959,-11.0775225261828));
#68570=CARTESIAN_POINT('Ctrl Pts',(36.4565960757825,0.108097735939015,-10.990355097404));
#68571=CARTESIAN_POINT('Ctrl Pts',(36.410105389827,0.114530376115748,-10.9033163103443));
#68572=CARTESIAN_POINT('Ctrl Pts',(36.3676968630231,0.120963016292481,-10.8139435316009));
#68573=CARTESIAN_POINT('Ctrl Pts',(36.3296046919639,0.127395656469215,-10.7226482908202));
#68574=CARTESIAN_POINT('Ctrl Pts',(36.2902379643555,0.134043531520685,-10.6282983292447));
#68575=CARTESIAN_POINT('Ctrl Pts',(36.2554817982704,0.140691406572158,-10.5318953484093));
#68576=CARTESIAN_POINT('Ctrl Pts',(36.2255435723802,0.147339281623628,-10.4339222260958));
#68577=CARTESIAN_POINT('Ctrl Pts',(36.1966455897759,0.153756167457046,-10.3393533095983));
#68578=CARTESIAN_POINT('Ctrl Pts',(36.172236440122,0.160173053290463,-10.2433219900157));
#68579=CARTESIAN_POINT('Ctrl Pts',(36.1524536760506,0.166589939123881,-10.1462825897148));
#68580=CARTESIAN_POINT('Ctrl Pts',(36.1326843947812,0.173002451574465,-10.0493093259259));
#68581=CARTESIAN_POINT('Ctrl Pts',(36.1175353100499,0.179414964025047,-9.95132975601396));
#68582=CARTESIAN_POINT('Ctrl Pts',(36.1070935047393,0.185827476475631,-9.85281101945179));
#68583=CARTESIAN_POINT('Ctrl Pts',(36.0966567355883,0.192236896124194,-9.75433979920243));
#68584=CARTESIAN_POINT('Ctrl Pts',(36.09092277005,0.198646315772756,-9.65533034449738));
#68585=CARTESIAN_POINT('Ctrl Pts',(36.0899270638497,0.205055735421318,-9.55625675487976));
#68586=CARTESIAN_POINT('Ctrl Pts',(36.0898175717336,0.205760542643165,-9.54536219885355));
#68587=CARTESIAN_POINT('Ctrl Pts',(36.0897653235704,0.206465349865013,-9.53446687122886));
#68588=CARTESIAN_POINT('Ctrl Pts',(36.0897703280922,0.20717015708686,-9.52357140469285));
#68589=CARTESIAN_POINT('',(36.089648114499,1.47717011009206,-9.52360304152045));
#68590=CARTESIAN_POINT('Ctrl Pts',(36.0940691872287,0.207171403211074,-9.52355414230154));
#68591=CARTESIAN_POINT('Ctrl Pts',(36.0923009265865,0.234573300440328,-9.10053859340738));
#68592=CARTESIAN_POINT('Ctrl Pts',(36.3693104484986,0.328843798156245,-7.64746453123767));
#68593=CARTESIAN_POINT('Ctrl Pts',(38.573297397462,0.489982896358807,-5.90905004425038));
#68594=CARTESIAN_POINT('Ctrl Pts',(41.8853621052223,0.690588697818804,-7.02366423740838));
#68595=CARTESIAN_POINT('Ctrl Pts',(42.7624419786364,0.891194499278781,-10.4063951343764));
#68596=CARTESIAN_POINT('Ctrl Pts',(40.4092341470354,1.09180030073876,-12.9899102462532));
#68597=CARTESIAN_POINT('Ctrl Pts',(37.050354743051,1.28712498014314,-12.4462743804594));
#68598=CARTESIAN_POINT('Ctrl Pts',(36.0908975709741,1.41558105906088,-10.4677289734402));
#68599=CARTESIAN_POINT('Ctrl Pts',(36.0855589174695,1.47716853749195,-9.52362531105487));
#68600=CARTESIAN_POINT('',(36.0897712274935,2.74717015704593,-9.52776325396536));
#68601=CARTESIAN_POINT('Ctrl Pts',(36.0897703140206,1.47717015708686,-9.52360237602881));
#68602=CARTESIAN_POINT('Ctrl Pts',(36.0898066400594,1.48245073927748,-9.4427635192502));
#68603=CARTESIAN_POINT('Ctrl Pts',(36.0929943645843,1.4877313214681,-9.36199917881014));
#68604=CARTESIAN_POINT('Ctrl Pts',(36.0993176964666,1.49301190365872,-9.28148428088808));
#68605=CARTESIAN_POINT('Ctrl Pts',(36.1069008108343,1.49934452377502,-9.18492858989839));
#68606=CARTESIAN_POINT('Ctrl Pts',(36.1190115282862,1.50567714389132,-9.08855973115984));
#68607=CARTESIAN_POINT('Ctrl Pts',(36.1356351547736,1.51200976400762,-8.9928357882755));
#68608=CARTESIAN_POINT('Ctrl Pts',(36.1522364085168,1.51833386142944,-8.89724067451801));
#68609=CARTESIAN_POINT('Ctrl Pts',(36.1733384254317,1.52465795885125,-8.80228917874195));
#68610=CARTESIAN_POINT('Ctrl Pts',(36.1988746331224,1.53098205627306,-8.70843574338361));
#68611=CARTESIAN_POINT('Ctrl Pts',(36.2243841120284,1.53729953425319,-8.61468054454834));
#68612=CARTESIAN_POINT('Ctrl Pts',(36.254318440425,1.54361701223332,-8.52202154094052));
#68613=CARTESIAN_POINT('Ctrl Pts',(36.2885599146599,1.54993449021344,-8.43090344010476));
#68614=CARTESIAN_POINT('Ctrl Pts',(36.3227770831705,1.55624748383999,-8.33985001789291));
#68615=CARTESIAN_POINT('Ctrl Pts',(36.3612951659185,1.56256047746653,-8.25033573214745));
#68616=CARTESIAN_POINT('Ctrl Pts',(36.4039467817926,1.56887347109307,-8.16278964405193));
#68617=CARTESIAN_POINT('Ctrl Pts',(36.4465829846588,1.57518418339406,-8.07527519247295));
#68618=CARTESIAN_POINT('Ctrl Pts',(36.493349561246,1.58149489569505,-7.98972791802753));
#68619=CARTESIAN_POINT('Ctrl Pts',(36.5440315860174,1.58780560799605,-7.90655555028078));
#68620=CARTESIAN_POINT('Ctrl Pts',(36.5947090231266,1.59411574906064,-7.82339071117447));
#68621=CARTESIAN_POINT('Ctrl Pts',(36.6493009760121,1.60042589012524,-7.74260072468242));
#68622=CARTESIAN_POINT('Ctrl Pts',(36.707547822154,1.60673603118983,-7.664566503728));
#68623=CARTESIAN_POINT('Ctrl Pts',(36.7658051718718,1.61304731015373,-7.58651821096692));
#68624=CARTESIAN_POINT('Ctrl Pts',(36.8277184622553,1.61935858911762,-7.51122702116066));
#68625=CARTESIAN_POINT('Ctrl Pts',(36.8929868674292,1.62566986808151,-7.4390419325773));
#68626=CARTESIAN_POINT('Ctrl Pts',(36.9583250727981,1.63198789653623,-7.36677964686851));
#68627=CARTESIAN_POINT('Ctrl Pts',(37.0270252625657,1.63830592499096,-7.2976304190209));
#68628=CARTESIAN_POINT('Ctrl Pts',(37.0987488571929,1.64462395344569,-7.2319072657758));
#68629=CARTESIAN_POINT('Ctrl Pts',(37.1705144795331,1.6509456840613,-7.16614560088277));
#68630=CARTESIAN_POINT('Ctrl Pts',(37.2453066987127,1.65726741467692,-7.10381428805981));
#68631=CARTESIAN_POINT('Ctrl Pts',(37.3227545141559,1.66358914529253,-7.04518548298915));
#68632=CARTESIAN_POINT('Ctrl Pts',(37.400326511541,1.66992101234362,-6.98646267089164));
#68633=CARTESIAN_POINT('Ctrl Pts',(37.4805622473205,1.67625287939471,-6.93145446822313));
#68634=CARTESIAN_POINT('Ctrl Pts',(37.5630625206456,1.6825847464458,-6.88038918901383));
#68635=CARTESIAN_POINT('Ctrl Pts',(37.6109800410629,1.68626239933677,-6.85072963201479));
#68636=CARTESIAN_POINT('Ctrl Pts',(37.6596610351012,1.68994005222774,-6.82239935129324));
#68637=CARTESIAN_POINT('Ctrl Pts',(37.7090239996132,1.69361770511871,-6.79543570891425));
#68638=CARTESIAN_POINT('Ctrl Pts',(37.7940230226877,1.69995032525265,-6.74900650265803));
#68639=CARTESIAN_POINT('Ctrl Pts',(37.8813404693319,1.70628294538659,-6.70647075351165));
#68640=CARTESIAN_POINT('Ctrl Pts',(37.9705847167663,1.71261556552053,-6.66806655410885));
#68641=CARTESIAN_POINT('Ctrl Pts',(38.0597088557022,1.71893966295953,-6.62971404062263));
#68642=CARTESIAN_POINT('Ctrl Pts',(38.1507542430837,1.72526376039853,-6.59548219671587));
#68643=CARTESIAN_POINT('Ctrl Pts',(38.2433039474916,1.73158785783753,-6.56556368272354));
#68644=CARTESIAN_POINT('Ctrl Pts',(38.3357567799864,1.73790533583434,-6.53567648448427));
#68645=CARTESIAN_POINT('Ctrl Pts',(38.4297103852599,1.74422281383116,-6.51009377439101));
#68646=CARTESIAN_POINT('Ctrl Pts',(38.5247280343997,1.75054029182797,-6.488960075135));
#68647=CARTESIAN_POINT('Ctrl Pts',(38.6196782368767,1.75685328547043,-6.46784137727609));
#68648=CARTESIAN_POINT('Ctrl Pts',(38.7156905559805,1.7631662791129,-6.45116550652999));
#68649=CARTESIAN_POINT('Ctrl Pts',(38.8123142101335,1.76947927275536,-6.43902683400591));
#68650=CARTESIAN_POINT('Ctrl Pts',(38.908902947404,1.77578998507179,-6.426892548033));
#68651=CARTESIAN_POINT('Ctrl Pts',(39.0061021472945,1.78210069738822,-6.41929225682063));
#68652=CARTESIAN_POINT('Ctrl Pts',(39.1034529022483,1.78841140970466,-6.41626885839002));
#68653=CARTESIAN_POINT('Ctrl Pts',(39.2007948451471,1.79472155078419,-6.41324573363323));
#68654=CARTESIAN_POINT('Ctrl Pts',(39.2982878787266,1.80103169186372,-6.41479869131284));
#68655=CARTESIAN_POINT('Ctrl Pts',(39.3954711189734,1.80734183294325,-6.42091854253995));
#68656=CARTESIAN_POINT('Ctrl Pts',(39.4926718841358,1.81365311192156,-6.42703949735114));
#68657=CARTESIAN_POINT('Ctrl Pts',(39.5895623085709,1.81996439089987,-6.43772895384787));
#68658=CARTESIAN_POINT('Ctrl Pts',(39.6856857104737,1.82627566987818,-6.45292577505985));
#68659=CARTESIAN_POINT('Ctrl Pts',(39.781911909914,1.83259369834646,-6.46813884825383));
#68660=CARTESIAN_POINT('Ctrl Pts',(39.8773690165199,1.83891172681473,-6.48786884127477));
#68661=CARTESIAN_POINT('Ctrl Pts',(39.971609841885,1.84522975528301,-6.51200333475024));
#68662=CARTESIAN_POINT('Ctrl Pts',(40.065905889327,1.85155148591172,-6.53615197025862));
#68663=CARTESIAN_POINT('Ctrl Pts',(40.1589838184526,1.85787321654042,-6.56471011727024));
#68664=CARTESIAN_POINT('Ctrl Pts',(40.2504129351984,1.86419494716912,-6.59751587220905));
#68665=CARTESIAN_POINT('Ctrl Pts',(40.3419886518735,1.87052681423244,-6.63037422878645));
#68666=CARTESIAN_POINT('Ctrl Pts',(40.4319098730917,1.87685868129575,-6.66749362636479));
#68667=CARTESIAN_POINT('Ctrl Pts',(40.5197672021754,1.88319054835907,-6.7086645823052));
#68668=CARTESIAN_POINT('Ctrl Pts',(40.5707961868006,1.88686820109894,-6.73257735201492));
#68669=CARTESIAN_POINT('Ctrl Pts',(40.6211293892347,1.89054585383882,-6.75785604784021));
#68670=CARTESIAN_POINT('Ctrl Pts',(40.6706909720238,1.89422350657869,-6.78445284337091));
#68671=CARTESIAN_POINT('Ctrl Pts',(40.7560320055585,1.90055612688944,-6.83025037225457));
#68672=CARTESIAN_POINT('Ctrl Pts',(40.8393800241139,1.90688874720019,-6.88011754359707));
#68673=CARTESIAN_POINT('Ctrl Pts',(40.9203215848964,1.91322136751093,-6.93385656563757));
#68674=CARTESIAN_POINT('Ctrl Pts',(41.0011542112844,1.91954546512762,-6.98752326354975));
#68675=CARTESIAN_POINT('Ctrl Pts',(41.0795864557308,1.9258695627443,-7.04505121542693));
#68676=CARTESIAN_POINT('Ctrl Pts',(41.1552290854296,1.93219366036099,-7.10619660236922));
#68677=CARTESIAN_POINT('Ctrl Pts',(41.2307925398855,1.93851113853614,-7.16727798835221));
#68678=CARTESIAN_POINT('Ctrl Pts',(41.303571846174,1.94482861671129,-7.23196900843589));
#68679=CARTESIAN_POINT('Ctrl Pts',(41.3732072593789,1.95114609488644,-7.29998295272083));
#68680=CARTESIAN_POINT('Ctrl Pts',(41.4427932430732,1.95745908870744,-7.36794861846727));
#68681=CARTESIAN_POINT('Ctrl Pts',(41.5092394583548,1.96377208252843,-7.43923221443983));
#68682=CARTESIAN_POINT('Ctrl Pts',(41.5722204748629,1.97008507634943,-7.51350784949553));
#68683=CARTESIAN_POINT('Ctrl Pts',(41.6351787319272,1.97639578884446,-7.58775664357211));
#68684=CARTESIAN_POINT('Ctrl Pts',(41.6946739958512,1.98270650133949,-7.66499499510333));
#68685=CARTESIAN_POINT('Ctrl Pts',(41.7504194970726,1.98901721383451,-7.74486207223943));
#68686=CARTESIAN_POINT('Ctrl Pts',(41.8061599522876,1.99532735509248,-7.82472191991698));
#68687=CARTESIAN_POINT('Ctrl Pts',(41.8581510695283,2.00163749635045,-7.90720966138386));
#68688=CARTESIAN_POINT('Ctrl Pts',(41.906148615479,2.00794763760841,-7.99193433805305));
#68689=CARTESIAN_POINT('Ctrl Pts',(41.954154816756,2.01425891676477,-8.07667429299728));
#68690=CARTESIAN_POINT('Ctrl Pts',(41.9981658009022,2.02057019592113,-8.16365160380412));
#68691=CARTESIAN_POINT('Ctrl Pts',(42.0379831319713,2.0268814750775,-8.25245043493534));
#68692=CARTESIAN_POINT('Ctrl Pts',(42.0778430449963,2.03319950372217,-8.34134423044031));
#68693=CARTESIAN_POINT('Ctrl Pts',(42.1135001720061,2.03951753236684,-8.43206303564065));
#68694=CARTESIAN_POINT('Ctrl Pts',(42.14480420926,2.04583556101151,-8.52417093266402));
#68695=CARTESIAN_POINT('Ctrl Pts',(42.1761265896638,2.05215729181592,-8.6163328019258));
#68696=CARTESIAN_POINT('Ctrl Pts',(42.2030906799729,2.05847902262034,-8.70988496381116));
#68697=CARTESIAN_POINT('Ctrl Pts',(42.2255966297227,2.06480075342475,-8.80437826350402));
#68698=CARTESIAN_POINT('Ctrl Pts',(42.2481386661128,2.07113262066097,-8.89902307627427));
#68699=CARTESIAN_POINT('Ctrl Pts',(42.2662082068624,2.07746448789719,-8.99461161071951));
#68700=CARTESIAN_POINT('Ctrl Pts',(42.2797568848875,2.08379635513341,-9.09068653844481));
#68701=CARTESIAN_POINT('Ctrl Pts',(42.287626176362,2.08747400610183,-9.14648841138497));
#68702=CARTESIAN_POINT('Ctrl Pts',(42.2939713403462,2.09115165707025,-9.20245429005291));
#68703=CARTESIAN_POINT('Ctrl Pts',(42.2987909716045,2.09482930803867,-9.25849452688035));
#68704=CARTESIAN_POINT('Ctrl Pts',(42.3070899898936,2.10116192790374,-9.35499131790932));
#68705=CARTESIAN_POINT('Ctrl Pts',(42.3108917458408,2.10749454776881,-9.45204373863104));
#68706=CARTESIAN_POINT('Ctrl Pts',(42.3101358709359,2.11382716763389,-9.54919746304091));
#68707=CARTESIAN_POINT('Ctrl Pts',(42.3093810133178,2.12015126480478,-9.64622043406605));
#68708=CARTESIAN_POINT('Ctrl Pts',(42.3040807195195,2.12647536197567,-9.74334400419317));
#68709=CARTESIAN_POINT('Ctrl Pts',(42.2942263969418,2.13279945914657,-9.84010896110503));
#68710=CARTESIAN_POINT('Ctrl Pts',(42.2843823888969,2.13911693687639,-9.93677263400554));
#68711=CARTESIAN_POINT('Ctrl Pts',(42.2699938725908,2.14543441460622,-10.0330780071489));
#68712=CARTESIAN_POINT('Ctrl Pts',(42.2511042901921,2.15175189233604,-10.1285671157971));
#68713=CARTESIAN_POINT('Ctrl Pts',(42.2322281162346,2.15806488571424,-10.2239884431632));
#68714=CARTESIAN_POINT('Ctrl Pts',(42.2088573126661,2.16437787909245,-10.318594230155));
#68715=CARTESIAN_POINT('Ctrl Pts',(42.1810868882884,2.17069087247065,-10.4119338291975));
#68716=CARTESIAN_POINT('Ctrl Pts',(42.1533264992995,2.1770015845246,-10.5052396981411));
#68717=CARTESIAN_POINT('Ctrl Pts',(42.1211697732094,2.18331229657855,-10.5972798695859));
#68718=CARTESIAN_POINT('Ctrl Pts',(42.0847621102454,2.1896230086325,-10.687616970542));
#68719=CARTESIAN_POINT('Ctrl Pts',(42.0483577428405,2.19593314945165,-10.777945894339));
#68720=CARTESIAN_POINT('Ctrl Pts',(42.0077033672699,2.20224329027079,-10.8665716486195));
#68721=CARTESIAN_POINT('Ctrl Pts',(41.96299286245,2.20855343108994,-10.9530760116151));
#68722=CARTESIAN_POINT('Ctrl Pts',(41.9182742950308,2.21486470981027,-11.0395959738533));
#68723=CARTESIAN_POINT('Ctrl Pts',(41.8694983464578,2.2211759885306,-11.1239933965491));
#68724=CARTESIAN_POINT('Ctrl Pts',(41.8169047608535,2.22748726725093,-11.2058748095924));
#68725=CARTESIAN_POINT('Ctrl Pts',(41.7642549298878,2.23380529546644,-11.2878437893915));
#68726=CARTESIAN_POINT('Ctrl Pts',(41.7077795477114,2.24012332368196,-11.3672910191359));
#68727=CARTESIAN_POINT('Ctrl Pts',(41.6477614849951,2.24644135189747,-11.4438523563512));
#68728=CARTESIAN_POINT('Ctrl Pts',(41.5877082536086,2.25276308227597,-11.5204585560679));
#68729=CARTESIAN_POINT('Ctrl Pts',(41.5241084935469,2.25908481265448,-11.5941751649656));
#68730=CARTESIAN_POINT('Ctrl Pts',(41.4572837385655,2.26540654303299,-11.6646730536481));
#68731=CARTESIAN_POINT('Ctrl Pts',(41.3903518348838,2.2717384098526,-11.7352839806374));
#68732=CARTESIAN_POINT('Ctrl Pts',(41.3201849258317,2.27807027667222,-11.8026655791142));
#68733=CARTESIAN_POINT('Ctrl Pts',(41.2471395313558,2.28440214349183,-11.8665273630817));
#68734=CARTESIAN_POINT('Ctrl Pts',(41.2047135308746,2.28807979882744,-11.9036193672632));
#68735=CARTESIAN_POINT('Ctrl Pts',(41.1613170758136,2.29175745416305,-11.939524741118));
#68736=CARTESIAN_POINT('Ctrl Pts',(41.1170244675346,2.29543510949865,-11.9741933046973));
#68737=CARTESIAN_POINT('Ctrl Pts',(41.0407562374487,2.30176772964027,-12.0338897210192));
#68738=CARTESIAN_POINT('Ctrl Pts',(40.9615644445541,2.30810034978189,-12.0901239304866));
#68739=CARTESIAN_POINT('Ctrl Pts',(40.879796534497,2.3144329699235,-12.1425970384289));
#68740=CARTESIAN_POINT('Ctrl Pts',(40.7981386710133,2.32075706736781,-12.194999525932));
#68741=CARTESIAN_POINT('Ctrl Pts',(40.7139119462155,2.32708116481211,-12.2436507383664));
#68742=CARTESIAN_POINT('Ctrl Pts',(40.627496199149,2.33340526225642,-12.2882924663009));
#68743=CARTESIAN_POINT('Ctrl Pts',(40.5411709036052,2.33972274025621,-12.332887467656));
#68744=CARTESIAN_POINT('Ctrl Pts',(40.4526615274063,2.34604021825601,-12.3734811281637));
#68745=CARTESIAN_POINT('Ctrl Pts',(40.362375308086,2.3523576962558,-12.4098594932946));
#68746=CARTESIAN_POINT('Ctrl Pts',(40.272153176953,2.35867068989778,-12.4462120358415));
#68747=CARTESIAN_POINT('Ctrl Pts',(40.180157114639,2.36498368353976,-12.4783550686288));
#68748=CARTESIAN_POINT('Ctrl Pts',(40.0868164187175,2.37129667718173,-12.5061218177715));
#68749=CARTESIAN_POINT('Ctrl Pts',(39.9935094533476,2.37760738949555,-12.5338785328367));
#68750=CARTESIAN_POINT('Ctrl Pts',(39.8988592386145,2.38391810180936,-12.5572619820688));
#68751=CARTESIAN_POINT('Ctrl Pts',(39.803311501106,2.39022881412317,-12.5761548445684));
#68752=CARTESIAN_POINT('Ctrl Pts',(39.7077724124777,2.39653895519797,-12.5950459969061));
#68753=CARTESIAN_POINT('Ctrl Pts',(39.6113363916488,2.40284909627276,-12.6094472860701));
#68754=CARTESIAN_POINT('Ctrl Pts',(39.5144596276978,2.40915923734756,-12.6192924547379));
#68755=CARTESIAN_POINT('Ctrl Pts',(39.4175653941298,2.41547051631904,-12.6291393987678));
#68756=CARTESIAN_POINT('Ctrl Pts',(39.3202306946555,2.42178179529052,-12.6344285463271));
#68757=CARTESIAN_POINT('Ctrl Pts',(39.2229160625637,2.42809307426199,-12.6351455764926));
#68758=CARTESIAN_POINT('Ctrl Pts',(39.1254973590417,2.43441110272032,-12.6358633734735));
#68759=CARTESIAN_POINT('Ctrl Pts',(39.0280992037688,2.44072913117864,-12.6319992880725));
#68760=CARTESIAN_POINT('Ctrl Pts',(38.9311811454028,2.44704715963696,-12.6235911437802));
#68761=CARTESIAN_POINT('Ctrl Pts',(38.8342062962151,2.45336889025393,-12.6151780725895));
#68762=CARTESIAN_POINT('Ctrl Pts',(38.7377125373498,2.45969062087089,-12.6022156986011));
#68763=CARTESIAN_POINT('Ctrl Pts',(38.6421512321369,2.46601235148786,-12.5847933598682));
#68764=CARTESIAN_POINT('Ctrl Pts',(38.5464367013714,2.47234421853678,-12.5673430856914));
#68765=CARTESIAN_POINT('Ctrl Pts',(38.4516580355461,2.4786760855857,-12.5454186655204));
#68766=CARTESIAN_POINT('Ctrl Pts',(38.3582533628398,2.48500795263461,-12.5191598574107));
#68767=CARTESIAN_POINT('Ctrl Pts',(38.3040023889813,2.48868560540929,-12.503908308735));
#68768=CARTESIAN_POINT('Ctrl Pts',(38.2502146079462,2.49236325818397,-12.4871954868035));
#68769=CARTESIAN_POINT('Ctrl Pts',(38.1969726538517,2.49604091095864,-12.4690561808122));
#68770=CARTESIAN_POINT('Ctrl Pts',(38.1052943060448,2.50237353221427,-12.4378217599138));
#68771=CARTESIAN_POINT('Ctrl Pts',(38.0149170724324,2.50870615346988,-12.4022466924457));
#68772=CARTESIAN_POINT('Ctrl Pts',(37.9262811623457,2.5150387747255,-12.3624585416363));
#68773=CARTESIAN_POINT('Ctrl Pts',(37.8377645419445,2.52136287329097,-12.3227239392813));
#68774=CARTESIAN_POINT('Ctrl Pts',(37.7509849827616,2.52768697185644,-12.2787877008172));
#68775=CARTESIAN_POINT('Ctrl Pts',(37.666366331892,2.53401107042191,-12.230826754422));
#68776=CARTESIAN_POINT('Ctrl Pts',(37.5818362514309,2.54032854954844,-12.1829160087871));
#68777=CARTESIAN_POINT('Ctrl Pts',(37.4994629611205,2.54664602867496,-12.1309891447054));
#68778=CARTESIAN_POINT('Ctrl Pts',(37.4196482263398,2.55296350780148,-12.0752702239027));
#68779=CARTESIAN_POINT('Ctrl Pts',(37.33989014668,2.55927650257376,-12.0195908542206));
#68780=CARTESIAN_POINT('Ctrl Pts',(37.2626873695045,2.56558949734605,-11.9601250287466));
#68781=CARTESIAN_POINT('Ctrl Pts',(37.1884142104197,2.57190249211833,-11.8971410717027));
#68782=CARTESIAN_POINT('Ctrl Pts',(37.1141678914201,2.57821320556423,-11.834179875166));
#68783=CARTESIAN_POINT('Ctrl Pts',(37.0428494201068,2.58452391901013,-11.7677033557909));
#68784=CARTESIAN_POINT('Ctrl Pts',(36.9748006814745,2.59083463245603,-11.6980206270843));
#68785=CARTESIAN_POINT('Ctrl Pts',(36.9067581025372,2.59714477466328,-11.6283442059795));
#68786=CARTESIAN_POINT('Ctrl Pts',(36.8419849732057,2.60345491687054,-11.55546246559));
#68787=CARTESIAN_POINT('Ctrl Pts',(36.7807861377721,2.60976505907779,-11.4797211928315));
#68788=CARTESIAN_POINT('Ctrl Pts',(36.7195762664718,2.6160763391807,-11.4039662617968));
#68789=CARTESIAN_POINT('Ctrl Pts',(36.6619422440296,2.6223876192836,-11.3253511144098));
#68790=CARTESIAN_POINT('Ctrl Pts',(36.6081477987834,2.62869889938651,-11.2442535647626));
#68791=CARTESIAN_POINT('Ctrl Pts',(36.5542958240918,2.63501692896779,-11.1630692868846));
#68792=CARTESIAN_POINT('Ctrl Pts',(36.5042918664585,2.64133495854907,-11.0793976716945));
#68793=CARTESIAN_POINT('Ctrl Pts',(36.4583554512351,2.64765298813035,-10.9936442118933));
#68794=CARTESIAN_POINT('Ctrl Pts',(36.4123921187981,2.65397471986712,-10.9078405034127));
#68795=CARTESIAN_POINT('Ctrl Pts',(36.3705012629379,2.6602964516039,-10.8199529157724));
#68796=CARTESIAN_POINT('Ctrl Pts',(36.3328547974104,2.66661818334068,-10.7304082462666));
#68797=CARTESIAN_POINT('Ctrl Pts',(36.2951479686393,2.6729500514934,-10.640719998695));
#68798=CARTESIAN_POINT('Ctrl Pts',(36.2616992699725,2.67928191964612,-10.5493697740765));
#68799=CARTESIAN_POINT('Ctrl Pts',(36.2326311598061,2.68561378779884,-10.456800847363));
#68800=CARTESIAN_POINT('Ctrl Pts',(36.2157479766986,2.68929142933876,-10.4030354621756));
#68801=CARTESIAN_POINT('Ctrl Pts',(36.2003416177388,2.69296907087869,-10.3488591891142));
#68802=CARTESIAN_POINT('Ctrl Pts',(36.1864281203344,2.69664671241861,-10.2943602400623));
#68803=CARTESIAN_POINT('Ctrl Pts',(36.1545708458623,2.70506728652316,-10.1695758003257));
#68804=CARTESIAN_POINT('Ctrl Pts',(36.1304509100632,2.71348786062771,-10.042742164824));
#68805=CARTESIAN_POINT('Ctrl Pts',(36.1142797500045,2.72190843473227,-9.91469371520203));
#68806=CARTESIAN_POINT('Ctrl Pts',(36.0981085899458,2.73032900883682,-9.78664526558008));
#68807=CARTESIAN_POINT('Ctrl Pts',(36.0898863856997,2.73874958294137,-9.65738158475599));
#68808=CARTESIAN_POINT('Ctrl Pts',(36.0897712274935,2.74717015704592,-9.52776325396536));
#68809=CARTESIAN_POINT('',(36.0897702810346,4.01717015712308,-9.52367781839343));
#68810=CARTESIAN_POINT('Ctrl Pts',(36.0897712274929,2.74717015708686,-9.52776325333526));
#68811=CARTESIAN_POINT('Ctrl Pts',(36.0896857067451,2.75342358861985,-9.43150385974016));
#68812=CARTESIAN_POINT('Ctrl Pts',(36.0940731888462,2.75967702015284,-9.33513286548138));
#68813=CARTESIAN_POINT('Ctrl Pts',(36.1029378738701,2.76593045168583,-9.23910344564557));
#68814=CARTESIAN_POINT('Ctrl Pts',(36.1117861814384,2.77217233003931,-9.1432514396215));
#68815=CARTESIAN_POINT('Ctrl Pts',(36.1250951477522,2.7784142083928,-9.04774019554694));
#68816=CARTESIAN_POINT('Ctrl Pts',(36.1428168738931,2.78465608674629,-8.95301924302696));
#68817=CARTESIAN_POINT('Ctrl Pts',(36.1605334922914,2.79089616607027,-8.85832559090906));
#68818=CARTESIAN_POINT('Ctrl Pts',(36.1826602619927,2.79713624539425,-8.76442221820453));
#68819=CARTESIAN_POINT('Ctrl Pts',(36.2090978226404,2.80337632471823,-8.67175043605885));
#68820=CARTESIAN_POINT('Ctrl Pts',(36.2355353226703,2.80961638973452,-8.57907886639747));
#68821=CARTESIAN_POINT('Ctrl Pts',(36.2662834698003,2.81585645475081,-8.48763931238116));
#68822=CARTESIAN_POINT('Ctrl Pts',(36.3011928119984,2.8220965197671,-8.3978586869028));
#68823=CARTESIAN_POINT('Ctrl Pts',(36.3362304586393,2.8283595192764,-8.30774808519484));
#68824=CARTESIAN_POINT('Ctrl Pts',(36.3754597886764,2.83462251878569,-8.21930905567815));
#68825=CARTESIAN_POINT('Ctrl Pts',(36.4186812940064,2.84088551829498,-8.1329522606642));
#68826=CARTESIAN_POINT('Ctrl Pts',(36.4618047166418,2.84713430516028,-8.04679143538992));
#68827=CARTESIAN_POINT('Ctrl Pts',(36.5089019591111,2.85338309202559,-7.96270377705377));
#68828=CARTESIAN_POINT('Ctrl Pts',(36.5597299468514,2.85963187889089,-7.88107034841914));
#68829=CARTESIAN_POINT('Ctrl Pts',(36.6107313442735,2.86590198472218,-7.7991584112795));
#68830=CARTESIAN_POINT('Ctrl Pts',(36.6654887176831,2.87217209055346,-7.7197178436163));
#68831=CARTESIAN_POINT('Ctrl Pts',(36.7237151099566,2.87844219638475,-7.64310101327331));
#68832=CARTESIAN_POINT('Ctrl Pts',(36.7819415022302,2.88471230221603,-7.56648418293031));
#68833=CARTESIAN_POINT('Ctrl Pts',(36.8436365754505,2.89098240804732,-7.4926913920379));
#68834=CARTESIAN_POINT('Ctrl Pts',(36.9084766575112,2.8972525138786,-7.4220374649726));
#68835=CARTESIAN_POINT('Ctrl Pts',(36.9739632171509,2.90358513478866,-7.35067909432449));
#68836=CARTESIAN_POINT('Ctrl Pts',(37.0428998635996,2.90991775569873,-7.28225858062534));
#68837=CARTESIAN_POINT('Ctrl Pts',(37.1149926712673,2.91625037660879,-7.21712758324237));
#68838=CARTESIAN_POINT('Ctrl Pts',(37.1869884533318,2.9225744748051,-7.15208424195867));
#68839=CARTESIAN_POINT('Ctrl Pts',(37.2621316323609,2.92889857300141,-7.09032190846517));
#68840=CARTESIAN_POINT('Ctrl Pts',(37.3400896756765,2.93522267119771,-7.03215739799427));
#68841=CARTESIAN_POINT('Ctrl Pts',(37.4179661199614,2.94154014993231,-6.97405376857516));
#68842=CARTESIAN_POINT('Ctrl Pts',(37.4986512224208,2.94785762866692,-6.91954073561128));
#68843=CARTESIAN_POINT('Ctrl Pts',(37.5817781876478,2.95417510740152,-6.86889593221058));
#68844=CARTESIAN_POINT('Ctrl Pts',(37.6648461461997,2.96048810174993,-6.81828707841358));
#68845=CARTESIAN_POINT('Ctrl Pts',(37.7503521491603,2.96680109609834,-6.77154122221721));
#68846=CARTESIAN_POINT('Ctrl Pts',(37.8378999269094,2.97311409044675,-6.7288930557315));
#68847=CARTESIAN_POINT('Ctrl Pts',(37.9254160672524,2.97942480344924,-6.68626030114313));
#68848=CARTESIAN_POINT('Ctrl Pts',(38.0149721235363,2.98573551645172,-6.64772248523414));
#68849=CARTESIAN_POINT('Ctrl Pts',(38.1061475358688,2.99204622945421,-6.61346819704573));
#68850=CARTESIAN_POINT('Ctrl Pts',(38.1973146948333,2.99835637119921,-6.57921700961925));
#68851=CARTESIAN_POINT('Ctrl Pts',(38.2901005089509,3.00466651294421,-6.54924873257616));
#68852=CARTESIAN_POINT('Ctrl Pts',(38.3840657511376,3.0109766546892,-6.52370328783818));
#68853=CARTESIAN_POINT('Ctrl Pts',(38.4780479376236,3.01728793431165,-6.49815323661327));
#68854=CARTESIAN_POINT('Ctrl Pts',(38.5732095525892,3.02359921393409,-6.47702771641294));
#68855=CARTESIAN_POINT('Ctrl Pts',(38.6690985951302,3.02991049355653,-6.4604161210358));
#68856=CARTESIAN_POINT('Ctrl Pts',(38.7650901840176,3.03622852263282,-6.44378676076741));
#68857=CARTESIAN_POINT('Ctrl Pts',(38.861810321972,3.0425465517091,-6.43168103756005));
#68858=CARTESIAN_POINT('Ctrl Pts',(38.9587994574682,3.04886458078539,-6.42413674097319));
#68859=CARTESIAN_POINT('Ctrl Pts',(39.0558454251575,3.05518631200261,-6.41658802369614));
#68860=CARTESIAN_POINT('Ctrl Pts',(39.1531602673442,3.06150804321983,-6.41360606877045));
#68861=CARTESIAN_POINT('Ctrl Pts',(39.250284088696,3.06782977443705,-6.41517650608206));
#68862=CARTESIAN_POINT('Ctrl Pts',(39.3475636404491,3.07416164205258,-6.41674946146625));
#68863=CARTESIAN_POINT('Ctrl Pts',(39.4446511236004,3.08049350966811,-6.42288935713051));
#68864=CARTESIAN_POINT('Ctrl Pts',(39.5410914598249,3.08682537728365,-6.43352991783286));
#68865=CARTESIAN_POINT('Ctrl Pts',(39.597105489185,3.09050302330196,-6.43971011901137));
#68866=CARTESIAN_POINT('Ctrl Pts',(39.6529013713708,3.09418066932027,-6.44740764080296));
#68867=CARTESIAN_POINT('Ctrl Pts',(39.7083918981512,3.09785831533858,-6.4566016668636));
#68868=CARTESIAN_POINT('Ctrl Pts',(39.8039423757478,3.10419094279536,-6.47243308227991));
#68869=CARTESIAN_POINT('Ctrl Pts',(39.8989186247315,3.11052357025214,-6.49275943423228));
#68870=CARTESIAN_POINT('Ctrl Pts',(39.992865506002,3.11685619770893,-6.5175268176936));
#68871=CARTESIAN_POINT('Ctrl Pts',(40.0866859504796,3.12318030250806,-6.54226086839825));
#68872=CARTESIAN_POINT('Ctrl Pts',(40.1794793614124,3.12950440730719,-6.57142396073292));
#68873=CARTESIAN_POINT('Ctrl Pts',(40.2707986742641,3.13582851210632,-6.60491081435956));
#68874=CARTESIAN_POINT('Ctrl Pts',(40.3620224035563,3.14214599749026,-6.63836261743045));
#68875=CARTESIAN_POINT('Ctrl Pts',(40.4517746937712,3.14846348287419,-6.67612903478748));
#68876=CARTESIAN_POINT('Ctrl Pts',(40.5396225621817,3.15478096825812,-6.71805467744851));
#68877=CARTESIAN_POINT('Ctrl Pts',(40.6274080734803,3.16109396929713,-6.75995056000221));
#68878=CARTESIAN_POINT('Ctrl Pts',(40.7132914569184,3.16740697033614,-6.80599961059708));
#68879=CARTESIAN_POINT('Ctrl Pts',(40.7968595766655,3.17371997137514,-6.85599828675372));
#68880=CARTESIAN_POINT('Ctrl Pts',(40.8803974974827,3.18003069109112,-6.9059788949375));
#68881=CARTESIAN_POINT('Ctrl Pts',(40.9616214421778,3.1863414108071,-6.95990606837964));
#68882=CARTESIAN_POINT('Ctrl Pts',(41.0401436033027,3.19265213052307,-7.0175307235932));
#68883=CARTESIAN_POINT('Ctrl Pts',(41.1186586566432,3.19896227899604,-7.07515016265347));
#68884=CARTESIAN_POINT('Ctrl Pts',(41.1944720602269,3.205272427469,-7.13646615913693));
#68885=CARTESIAN_POINT('Ctrl Pts',(41.2672265557435,3.21158257594197,-7.20118739565153));
#68886=CARTESIAN_POINT('Ctrl Pts',(41.3399941707842,3.21789386229851,-7.26592030308511));
#68887=CARTESIAN_POINT('Ctrl Pts',(41.4097014554993,3.22420514865504,-7.33405937945335));
#68888=CARTESIAN_POINT('Ctrl Pts',(41.4760264805007,3.23051643501158,-7.40527499119348));
#68889=CARTESIAN_POINT('Ctrl Pts',(41.5424224348733,3.23683447078997,-7.4765667624008));
#68890=CARTESIAN_POINT('Ctrl Pts',(41.6054286097377,3.24315250656836,-7.55094131696089));
#68891=CARTESIAN_POINT('Ctrl Pts',(41.6647621608396,3.24947054234675,-7.62803449072118));
#68892=CARTESIAN_POINT('Ctrl Pts',(41.724130479183,3.25579228025778,-7.7051728381976));
#68893=CARTESIAN_POINT('Ctrl Pts',(41.7798216384679,3.2621140181688,-7.78503261844524));
#68894=CARTESIAN_POINT('Ctrl Pts',(41.8315962840512,3.26843575607983,-7.8672208679477));
#68895=CARTESIAN_POINT('Ctrl Pts',(41.8834539454656,3.27476763030993,-7.94954089866794));
#68896=CARTESIAN_POINT('Ctrl Pts',(41.9313823382706,3.28109950454002,-8.03419647344177));
#68897=CARTESIAN_POINT('Ctrl Pts',(41.9751882052804,3.28743137877011,-8.1207702900976));
#68898=CARTESIAN_POINT('Ctrl Pts',(42.0006308381811,3.29110895811293,-8.17105272910263));
#68899=CARTESIAN_POINT('Ctrl Pts',(42.0246837016427,3.29478653745574,-8.22198186775086));
#68900=CARTESIAN_POINT('Ctrl Pts',(42.0473165588172,3.29846411679856,-8.2734733056041));
#68901=CARTESIAN_POINT('Ctrl Pts',(42.0862891694655,3.30479671841183,-8.36213890110126));
#68902=CARTESIAN_POINT('Ctrl Pts',(42.1211839554828,3.31112932002509,-8.45278065774558));
#68903=CARTESIAN_POINT('Ctrl Pts',(42.1517972678665,3.31746192163836,-8.54498798868783));
#68904=CARTESIAN_POINT('Ctrl Pts',(42.1823693794774,3.32378600055154,-8.63707122285675));
#68905=CARTESIAN_POINT('Ctrl Pts',(42.2086713334622,3.33011007946473,-8.7307154319889));
#68906=CARTESIAN_POINT('Ctrl Pts',(42.2305469151543,3.33643415837791,-8.82548870777606));
#68907=CARTESIAN_POINT('Ctrl Pts',(42.2523995996431,3.34275161786848,-8.92016278423733));
#68908=CARTESIAN_POINT('Ctrl Pts',(42.269835024806,3.34906907735905,-9.01596315401371));
#68909=CARTESIAN_POINT('Ctrl Pts',(42.2827466333479,3.35538653684961,-9.11244231011624));
#68910=CARTESIAN_POINT('Ctrl Pts',(42.2956490769913,3.36169951209061,-9.20885298352962));
#68911=CARTESIAN_POINT('Ctrl Pts',(42.3040340300051,3.36801248733161,-9.30594105316998));
#68912=CARTESIAN_POINT('Ctrl Pts',(42.3078461066003,3.3743254625726,-9.40324930969573));
#68913=CARTESIAN_POINT('Ctrl Pts',(42.3116568056648,3.38063615655918,-9.50052240294554));
#68914=CARTESIAN_POINT('Ctrl Pts',(42.3108978946503,3.38694685054575,-9.59801508844345));
#68915=CARTESIAN_POINT('Ctrl Pts',(42.3055659679321,3.39325754453233,-9.6952664726896));
#68916=CARTESIAN_POINT('Ctrl Pts',(42.3002345237747,3.39956766737561,-9.79250905529271));
#68917=CARTESIAN_POINT('Ctrl Pts',(42.2903309109435,3.40587779021889,-9.88950994341774));
#68918=CARTESIAN_POINT('Ctrl Pts',(42.2759037884449,3.41218791306218,-9.98581073894882));
#68919=CARTESIAN_POINT('Ctrl Pts',(42.2614740640517,3.41849917391991,-10.0821289020811));
#68920=CARTESIAN_POINT('Ctrl Pts',(42.2425192745294,3.42481043477765,-10.177746289373));
#68921=CARTESIAN_POINT('Ctrl Pts',(42.2191394755936,3.43112169563538,-10.2722131421572));
#68922=CARTESIAN_POINT('Ctrl Pts',(42.1957346723996,3.43743970626871,-10.3667810254758));
#68923=CARTESIAN_POINT('Ctrl Pts',(42.1678955169209,3.44375771690205,-10.4601954925031));
#68924=CARTESIAN_POINT('Ctrl Pts',(42.1357723448205,3.45007572753538,-10.5520206386862));
#68925=CARTESIAN_POINT('Ctrl Pts',(42.1036303488395,3.45639744046426,-10.6438995935521));
#68926=CARTESIAN_POINT('Ctrl Pts',(42.0671995009236,3.46271915339315,-10.7341869676802));
#68927=CARTESIAN_POINT('Ctrl Pts',(42.0266780249898,3.46904086632204,-10.8224675317479));
#68928=CARTESIAN_POINT('Ctrl Pts',(41.9860915731618,3.47537271607198,-10.9108896530629));
#68929=CARTESIAN_POINT('Ctrl Pts',(41.9414015963321,3.48170456582192,-10.9972981505316));
#68930=CARTESIAN_POINT('Ctrl Pts',(41.8928518968493,3.48803641557186,-11.0813030921177));
#68931=CARTESIAN_POINT('Ctrl Pts',(41.8646519626102,3.49171424980076,-11.1300970878319));
#68932=CARTESIAN_POINT('Ctrl Pts',(41.8351506388072,3.49539208402966,-11.1780807039365));
#68933=CARTESIAN_POINT('Ctrl Pts',(41.8044020846547,3.49906991825855,-11.2251824708973));
#68934=CARTESIAN_POINT('Ctrl Pts',(41.7514580799431,3.50540255008824,-11.3062840459346));
#68935=CARTESIAN_POINT('Ctrl Pts',(41.6946302290773,3.51173518191792,-11.3850511066296));
#68936=CARTESIAN_POINT('Ctrl Pts',(41.6341510345655,3.51806781374761,-11.4610886843902));
#68937=CARTESIAN_POINT('Ctrl Pts',(41.5737532364699,3.5243919227532,-11.5370239263577));
#68938=CARTESIAN_POINT('Ctrl Pts',(41.5097141318353,3.53071603175879,-11.6102366472761));
#68939=CARTESIAN_POINT('Ctrl Pts',(41.4423100057695,3.53704014076438,-11.6803599446325));
#68940=CARTESIAN_POINT('Ctrl Pts',(41.3749764330928,3.54335763018524,-11.750409842383));
#68941=CARTESIAN_POINT('Ctrl Pts',(41.3042851428335,3.54967511960611,-11.8173764318364));
#68942=CARTESIAN_POINT('Ctrl Pts',(41.2305526257222,3.55599260902697,-11.880925866209));
#68943=CARTESIAN_POINT('Ctrl Pts',(41.1568724492895,3.56230561383648,-11.9444301885924));
#68944=CARTESIAN_POINT('Ctrl Pts',(41.0801556683079,3.56861861864599,-12.0045218937258));
#68945=CARTESIAN_POINT('Ctrl Pts',(41.0007548693125,3.5749316234555,-12.060904681479));
#68946=CARTESIAN_POINT('Ctrl Pts',(40.9213827653735,3.58124234677628,-12.1172670927714));
#68947=CARTESIAN_POINT('Ctrl Pts',(40.8393289270005,3.58755307009705,-12.1699229971051));
#68948=CARTESIAN_POINT('Ctrl Pts',(40.7549774391038,3.59386379341783,-12.2186176077495));
#68949=CARTESIAN_POINT('Ctrl Pts',(40.6706335889134,3.6001739453266,-12.2673078092821));
#68950=CARTESIAN_POINT('Ctrl Pts',(40.5839928816742,3.60648409723538,-12.3120372118093));
#68951=CARTESIAN_POINT('Ctrl Pts',(40.4954657722599,3.61279424914416,-12.3525959905551));
#68952=CARTESIAN_POINT('Ctrl Pts',(40.4069227015372,3.6191055387641,-12.3931620819893));
#68953=CARTESIAN_POINT('Ctrl Pts',(40.3164929507085,3.62541682838404,-12.4295558740468));
#68954=CARTESIAN_POINT('Ctrl Pts',(40.2246078346454,3.63172811800398,-12.4616153030459));
#68955=CARTESIAN_POINT('Ctrl Pts',(40.1326244588472,3.6380461567654,-12.4937090156279));
#68956=CARTESIAN_POINT('Ctrl Pts',(40.0391830242623,3.64436419552681,-12.5214589671988));
#68957=CARTESIAN_POINT('Ctrl Pts',(39.9447307286541,3.65068223428822,-12.5447527704596));
#68958=CARTESIAN_POINT('Ctrl Pts',(39.8502230898586,3.6570039750285,-12.5680602224444));
#68959=CARTESIAN_POINT('Ctrl Pts',(39.7547038394558,3.66332571576878,-12.5869062422387));
#68960=CARTESIAN_POINT('Ctrl Pts',(39.6586290390159,3.66964745650906,-12.6012298447079));
#68961=CARTESIAN_POINT('Ctrl Pts',(39.5624001957111,3.67597933330011,-12.6155764131239));
#68962=CARTESIAN_POINT('Ctrl Pts',(39.4656144585077,3.68231121009117,-12.6253860410088));
#68963=CARTESIAN_POINT('Ctrl Pts',(39.3687316197421,3.68864308688222,-12.6306497377198));
#68964=CARTESIAN_POINT('Ctrl Pts',(39.3124622163455,3.69232063116099,-12.6337068846549));
#68965=CARTESIAN_POINT('Ctrl Pts',(39.2561600520151,3.69599817543976,-12.6352315439811));
#68966=CARTESIAN_POINT('Ctrl Pts',(39.199914556952,3.69967571971853,-12.6352299988264));
#68967=CARTESIAN_POINT('Ctrl Pts',(39.1030608108006,3.7060083858216,-12.6352273380973));
#68968=CARTESIAN_POINT('Ctrl Pts',(39.0060389757696,3.71234105192467,-12.6306962713217));
#68969=CARTESIAN_POINT('Ctrl Pts',(38.9093068864271,3.71867371802774,-12.6216155987822));
#68970=CARTESIAN_POINT('Ctrl Pts',(38.8127049775187,3.7249978617343,-12.6125471468605));
#68971=CARTESIAN_POINT('Ctrl Pts',(38.7163924709999,3.73132200544085,-12.5989412990248));
#68972=CARTESIAN_POINT('Ctrl Pts',(38.6208276312334,3.73764614914741,-12.5808288597625));
#68973=CARTESIAN_POINT('Ctrl Pts',(38.5253628150799,3.74396367364438,-12.5627353780124));
#68974=CARTESIAN_POINT('Ctrl Pts',(38.4306445373297,3.75028119814135,-12.540144763181));
#68975=CARTESIAN_POINT('Ctrl Pts',(38.3371253587336,3.75659872263832,-12.5131395560381));
#68976=CARTESIAN_POINT('Ctrl Pts',(38.2436725604007,3.76291176293274,-12.4861535172924));
#68977=CARTESIAN_POINT('Ctrl Pts',(38.1514175880817,3.76922480322716,-12.4547592367898));
#68978=CARTESIAN_POINT('Ctrl Pts',(38.0608012918966,3.77553784352159,-12.4190900048816));
#68979=CARTESIAN_POINT('Ctrl Pts',(37.9702177403851,3.78184860256581,-12.3834336622374));
#68980=CARTESIAN_POINT('Ctrl Pts',(37.8812720949134,3.78815936161003,-12.3435055976874));
#68981=CARTESIAN_POINT('Ctrl Pts',(37.7943876603095,3.79447012065425,-12.2994881696288));
#68982=CARTESIAN_POINT('Ctrl Pts',(37.7075110900579,3.80078030847957,-12.2554747258115));
#68983=CARTESIAN_POINT('Ctrl Pts',(37.6226957497321,3.80709049630489,-12.2073728522452));
#68984=CARTESIAN_POINT('Ctrl Pts',(37.5403417079127,3.8134006841302,-12.1554115659733));
#68985=CARTESIAN_POINT('Ctrl Pts',(37.4579728159357,3.81971200981447,-12.1034409099938));
#68986=CARTESIAN_POINT('Ctrl Pts',(37.3780664737735,3.82602333549874,-12.0476096924764));
#68987=CARTESIAN_POINT('Ctrl Pts',(37.3009941580418,3.832334661183,-11.9881905052409));
#68988=CARTESIAN_POINT('Ctrl Pts',(37.2238394234699,3.83865273601109,-11.9287077768952));
#68989=CARTESIAN_POINT('Ctrl Pts',(37.1495251127038,3.84497081083918,-11.8656296861786));
#68990=CARTESIAN_POINT('Ctrl Pts',(37.0783897860474,3.85128888566726,-11.7992692789008));
#68991=CARTESIAN_POINT('Ctrl Pts',(37.0072127781336,3.857610662528,-11.732869988197));
#68992=CARTESIAN_POINT('Ctrl Pts',(36.9392187687496,3.86393243938874,-11.6631848640705));
#68993=CARTESIAN_POINT('Ctrl Pts',(36.8747081200652,3.87025421624949,-11.5905624720664));
#68994=CARTESIAN_POINT('Ctrl Pts',(36.8100940407202,3.87658612888733,-11.517823643751));
#68995=CARTESIAN_POINT('Ctrl Pts',(36.7489747487376,3.88291804152518,-11.4421384838086));
#68996=CARTESIAN_POINT('Ctrl Pts',(36.691609106351,3.88924995416303,-11.3638871029943));
#68997=CARTESIAN_POINT('Ctrl Pts',(36.6582946370077,3.89292714316819,-11.31844346951));
#68998=CARTESIAN_POINT('Ctrl Pts',(36.6262452941534,3.89660433217334,-11.2721348868709));
#68999=CARTESIAN_POINT('Ctrl Pts',(36.5955046880318,3.9002815211785,-11.2250396533127));
#69000=CARTESIAN_POINT('Ctrl Pts',(36.5415325528662,3.90673766395039,-11.1423532449447));
#69001=CARTESIAN_POINT('Ctrl Pts',(36.4914152766448,3.91319380672228,-11.0569619124821));
#69002=CARTESIAN_POINT('Ctrl Pts',(36.4454280277222,3.91964994949417,-10.9692520217889));
#69003=CARTESIAN_POINT('Ctrl Pts',(36.3995096965043,3.92609641692012,-10.8816735754525));
#69004=CARTESIAN_POINT('Ctrl Pts',(36.3577092741141,3.93254288434608,-10.7917838452957));
#69005=CARTESIAN_POINT('Ctrl Pts',(36.3202585619524,3.93898935177203,-10.6999978310158));
#69006=CARTESIAN_POINT('Ctrl Pts',(36.2824093203582,3.9455044188816,-10.6072350815531));
#69007=CARTESIAN_POINT('Ctrl Pts',(36.2490031659417,3.95201948599117,-10.5125357975657));
#69008=CARTESIAN_POINT('Ctrl Pts',(36.2202319394877,3.95853455310074,-10.4163545638243));
#69009=CARTESIAN_POINT('Ctrl Pts',(36.1918352140922,3.96496481675109,-10.3214252744139));
#69010=CARTESIAN_POINT('Ctrl Pts',(36.1679536071212,3.97139508040143,-10.2250527921383));
#69011=CARTESIAN_POINT('Ctrl Pts',(36.1487230800705,3.97782534405178,-10.1276937952272));
#69012=CARTESIAN_POINT('Ctrl Pts',(36.1291121296098,3.98438281289096,-10.0284088166985));
#69013=CARTESIAN_POINT('Ctrl Pts',(36.1143383994277,3.99094028173014,-9.92809828583084));
#69014=CARTESIAN_POINT('Ctrl Pts',(36.1044921442325,3.99749775056932,-9.82726109207431));
#69015=CARTESIAN_POINT('Ctrl Pts',(36.0946458890374,4.0040552194085,-9.72642389831778));
#69016=CARTESIAN_POINT('Ctrl Pts',(36.0897271825286,4.01061268824768,-9.62506049549556));
#69017=CARTESIAN_POINT('Ctrl Pts',(36.0897702810343,4.01717015708686,-9.5236778189534));
#69018=CARTESIAN_POINT('Ctrl Pts',(36.0897702810346,4.01717015712308,-9.52367781839343));
#69019=CARTESIAN_POINT('Ctrl Pts',(36.0898161331557,4.0241465875827,-9.41581772632917));
#69020=CARTESIAN_POINT('Ctrl Pts',(36.0954771164379,4.03112301804231,-9.30813600171421));
#69021=CARTESIAN_POINT('Ctrl Pts',(36.1066715293551,4.03809944850193,-9.20119508095537));
#69022=CARTESIAN_POINT('Ctrl Pts',(36.1177674248493,4.045014482267,-9.09519530324727));
#69023=CARTESIAN_POINT('Ctrl Pts',(36.1342995664637,4.05192951603208,-8.98992360536198));
#69024=CARTESIAN_POINT('Ctrl Pts',(36.15613770959,4.05884454979716,-8.88591236131493));
#69025=CARTESIAN_POINT('Ctrl Pts',(36.1782666950712,4.06585167860405,-8.78051588616198));
#69026=CARTESIAN_POINT('Ctrl Pts',(36.2058439016662,4.07285880741093,-8.67641397761243));
#69027=CARTESIAN_POINT('Ctrl Pts',(36.2386833095558,4.07986593621782,-8.57414033012391));
#69028=CARTESIAN_POINT('Ctrl Pts',(36.2715227174455,4.08687306502472,-8.47186668263539));
#69029=CARTESIAN_POINT('Ctrl Pts',(36.3096241442889,4.09388019383161,-8.37142155394688));
#69030=CARTESIAN_POINT('Ctrl Pts',(36.3527533462547,4.10088732263849,-8.27331427840847));
#69031=CARTESIAN_POINT('Ctrl Pts',(36.3917317158068,4.10722007269381,-8.18464902453411));
#69032=CARTESIAN_POINT('Ctrl Pts',(36.4349233715946,4.11355282274913,-8.09765223533168));
#69033=CARTESIAN_POINT('Ctrl Pts',(36.4821634778366,4.11988557280445,-8.01275157738719));
#69034=CARTESIAN_POINT('Ctrl Pts',(36.5293400015044,4.12620979932791,-7.92796519103984));
#69035=CARTESIAN_POINT('Ctrl Pts',(36.5805539346683,4.13253402585137,-7.84526970742359));
#69036=CARTESIAN_POINT('Ctrl Pts',(36.6355926609841,4.13885825237482,-7.7650722592954));
#69037=CARTESIAN_POINT('Ctrl Pts',(36.6905737706915,4.14517585846012,-7.68495876487191));
#69038=CARTESIAN_POINT('Ctrl Pts',(36.7493714673799,4.15149346454541,-7.60733846576996));
#69039=CARTESIAN_POINT('Ctrl Pts',(36.8117280675142,4.15781107063071,-7.53259245398925));
#69040=CARTESIAN_POINT('Ctrl Pts',(36.8740403860956,4.164124190368,-7.4578995219062));
#69041=CARTESIAN_POINT('Ctrl Pts',(36.9399063043555,4.17043731010529,-7.38607715408355));
#69042=CARTESIAN_POINT('Ctrl Pts',(37.0090263921805,4.17675042984257,-7.31747529963123));
#69043=CARTESIAN_POINT('Ctrl Pts',(37.0781214885987,4.18306126697653,-7.24889824921049));
#69044=CARTESIAN_POINT('Ctrl Pts',(37.150468106614,4.18937210411049,-7.1835397061674));
#69045=CARTESIAN_POINT('Ctrl Pts',(37.2257289566207,4.19568294124446,-7.12171381226167));
#69046=CARTESIAN_POINT('Ctrl Pts',(37.3009829773001,4.20199320571983,-7.05989352856711));
#69047=CARTESIAN_POINT('Ctrl Pts',(37.379150366166,4.20830347019521,-7.00160553407963));
#69048=CARTESIAN_POINT('Ctrl Pts',(37.4598604697883,4.21461373467058,-6.94712392301442));
#69049=CARTESIAN_POINT('Ctrl Pts',(37.5405851074183,4.22092513547745,-6.89263250108144));
#69050=CARTESIAN_POINT('Ctrl Pts',(37.6238530067577,4.22723653628432,-6.84194906857085));
#69051=CARTESIAN_POINT('Ctrl Pts',(37.709265128746,4.23354793709118,-6.79530401023717));
#69052=CARTESIAN_POINT('Ctrl Pts',(37.7947685493868,4.23986608427522,-6.74860909210754));
#69053=CARTESIAN_POINT('Ctrl Pts',(37.8824203841084,4.24618423145925,-6.7059613761455));
#69054=CARTESIAN_POINT('Ctrl Pts',(37.9717978053915,4.25250237864328,-6.66754483463716));
#69055=CARTESIAN_POINT('Ctrl Pts',(38.0612275755798,4.25882422640497,-6.62910579232423));
#69056=CARTESIAN_POINT('Ctrl Pts',(38.1523845356437,4.26514607416666,-6.5949030128498));
#69057=CARTESIAN_POINT('Ctrl Pts',(38.2448287117249,4.27146792192835,-6.56507120643841));
#69058=CARTESIAN_POINT('Ctrl Pts',(38.3374210594344,4.27779990249144,-6.53519158492911));
#69059=CARTESIAN_POINT('Ctrl Pts',(38.4313043212246,4.28413188305452,-6.50969704056112));
#69060=CARTESIAN_POINT('Ctrl Pts',(38.5260263442078,4.29046386361761,-6.48867159809778));
#69061=CARTESIAN_POINT('Ctrl Pts',(38.5810230314921,4.2941402837779,-6.4764639863117));
#69062=CARTESIAN_POINT('Ctrl Pts',(38.636302319507,4.29781670393818,-6.46576198716194));
#69063=CARTESIAN_POINT('Ctrl Pts',(38.691775037217,4.30149312409847,-6.45657401260773));
#69064=CARTESIAN_POINT('Ctrl Pts',(38.787330651996,4.30782601354583,-6.44074708734889));
#69065=CARTESIAN_POINT('Ctrl Pts',(38.8837921438038,4.31415890299318,-6.42936056874551));
#69066=CARTESIAN_POINT('Ctrl Pts',(38.9807112641447,4.32049179244054,-6.42251017677302));
#69067=CARTESIAN_POINT('Ctrl Pts',(39.0774999881135,4.32681616152776,-6.41566900141597));
#69068=CARTESIAN_POINT('Ctrl Pts',(39.1747446843783,4.33314053061498,-6.41335185329256));
#69069=CARTESIAN_POINT('Ctrl Pts',(39.2719881846059,4.33946489970221,-6.41560321699254));
#69070=CARTESIAN_POINT('Ctrl Pts',(39.3691299341042,4.3457826512863,-6.41785222497828));
#69071=CARTESIAN_POINT('Ctrl Pts',(39.466270055195,4.3521004028704,-6.4246602313055));
#69072=CARTESIAN_POINT('Ctrl Pts',(39.5629485540092,4.3584181544545,-6.43601974754732));
#69073=CARTESIAN_POINT('Ctrl Pts',(39.659558456741,4.36473142341822,-6.44737120389659));
#69074=CARTESIAN_POINT('Ctrl Pts',(39.7557069553029,4.37104469238195,-6.4632676989785));
#69075=CARTESIAN_POINT('Ctrl Pts',(39.8509373172772,4.37735796134568,-6.48364976336563));
#69076=CARTESIAN_POINT('Ctrl Pts',(39.9461332819041,4.38366894994734,-6.504024465721));
#69077=CARTESIAN_POINT('Ctrl Pts',(40.0404113417497,4.389979938549,-6.52888142660613));
#69078=CARTESIAN_POINT('Ctrl Pts',(40.1333240564461,4.39629092715066,-6.55810990116603));
#69079=CARTESIAN_POINT('Ctrl Pts',(40.2262283702829,4.40260134513366,-6.58733573298422));
#69080=CARTESIAN_POINT('Ctrl Pts',(40.3177671673656,4.40891176311666,-6.6209321611959));
#69081=CARTESIAN_POINT('Ctrl Pts',(40.4075083070617,4.41522218109967,-6.65873861253428));
#69082=CARTESIAN_POINT('Ctrl Pts',(40.4972656328219,4.42153373725442,-6.69655188279255));
#69083=CARTESIAN_POINT('Ctrl Pts',(40.5852242542767,4.42784529340916,-6.73857651452453));
#69084=CARTESIAN_POINT('Ctrl Pts',(40.6709731177269,4.43415684956391,-6.78460427313412));
#69085=CARTESIAN_POINT('Ctrl Pts',(40.7568136623554,4.44047515392361,-6.83068124381455));
#69086=CARTESIAN_POINT('Ctrl Pts',(40.8404393461987,4.44679345828331,-6.88076967916138));
#69087=CARTESIAN_POINT('Ctrl Pts',(40.9214649784174,4.45311176264302,-6.93461605529556));
#69088=CARTESIAN_POINT('Ctrl Pts',(41.0025380828147,4.4594337688396,-6.98849397953026));
#69089=CARTESIAN_POINT('Ctrl Pts',(41.0810077499224,4.46575577503618,-7.04613397008788));
#69090=CARTESIAN_POINT('Ctrl Pts',(41.1565206683713,4.47207778123276,-7.10724121816591));
#69091=CARTESIAN_POINT('Ctrl Pts',(41.2321546223702,4.47840992062922,-7.16844641172832));
#69092=CARTESIAN_POINT('Ctrl Pts',(41.3048220379171,4.48474206002569,-7.2331296695793));
#69093=CARTESIAN_POINT('Ctrl Pts',(41.3742053900307,4.49107419942216,-7.30095827942425));
#69094=CARTESIAN_POINT('Ctrl Pts',(41.4144725839746,4.49474910813426,-7.34032316601978));
#69095=CARTESIAN_POINT('Ctrl Pts',(41.4536343775838,4.49842401684636,-7.38074680055014));
#69096=CARTESIAN_POINT('Ctrl Pts',(41.4916350544945,4.50209892555846,-7.42215920005528));
#69097=CARTESIAN_POINT('Ctrl Pts',(41.5571069112291,4.50843047321161,-7.49350915768401));
#69098=CARTESIAN_POINT('Ctrl Pts',(41.6193573245284,4.51476202086475,-7.56804390007884));
#69099=CARTESIAN_POINT('Ctrl Pts',(41.67806115532,4.5210935685179,-7.64544059327879));
#69100=CARTESIAN_POINT('Ctrl Pts',(41.7366859502706,4.5274165916985,-7.72273308352204));
#69101=CARTESIAN_POINT('Ctrl Pts',(41.7917733909051,4.53373961487911,-7.8028795206477));
#69102=CARTESIAN_POINT('Ctrl Pts',(41.8430363558471,4.54006263805971,-7.8855215845976));
#69103=CARTESIAN_POINT('Ctrl Pts',(41.8942456519932,4.54637904147026,-7.96807712799477));
#69104=CARTESIAN_POINT('Ctrl Pts',(41.9416382030586,4.5526954448808,-8.05312273418323));
#69105=CARTESIAN_POINT('Ctrl Pts',(41.984968857296,4.55901184829135,-8.14026929809751));
#69106=CARTESIAN_POINT('Ctrl Pts',(42.0282687756684,4.56532377126821,-8.22735404607401));
#69107=CARTESIAN_POINT('Ctrl Pts',(42.0675123309939,4.57163569424508,-8.31653639843586));
#69108=CARTESIAN_POINT('Ctrl Pts',(42.1024996774301,4.57794761722194,-8.40740155895853));
#69109=CARTESIAN_POINT('Ctrl Pts',(42.137474393984,4.58425726169381,-8.49823391858623));
#69110=CARTESIAN_POINT('Ctrl Pts',(42.1681957974673,4.59056690616567,-8.59074747149895));
#69111=CARTESIAN_POINT('Ctrl Pts',(42.1945120558889,4.59687655063754,-8.68450716836111));
#69112=CARTESIAN_POINT('Ctrl Pts',(42.2208259489294,4.60318562798039,-8.77825843783179));
#69113=CARTESIAN_POINT('Ctrl Pts',(42.2427353661126,4.60949470532325,-8.87325520730227));
#69114=CARTESIAN_POINT('Ctrl Pts',(42.2601385630211,4.6158037826661,-8.96904799846442));
#69115=CARTESIAN_POINT('Ctrl Pts',(42.2775449136437,4.6221140033062,-9.06485814868369));
#69116=CARTESIAN_POINT('Ctrl Pts',(42.2904433439776,4.6284242239463,-9.16146417666143));
#69117=CARTESIAN_POINT('Ctrl Pts',(42.2987835467469,4.6347344445864,-9.25840820847109));
#69118=CARTESIAN_POINT('Ctrl Pts',(42.3071326896345,4.64105142934484,-9.35545615755111));
#69119=CARTESIAN_POINT('Ctrl Pts',(42.3109138125849,4.64736841410328,-9.45284239722024));
#69120=CARTESIAN_POINT('Ctrl Pts',(42.3101286699969,4.65368539886173,-9.55010595474015));
#69121=CARTESIAN_POINT('Ctrl Pts',(42.3093430664287,4.66000609250672,-9.64742661854001));
#69122=CARTESIAN_POINT('Ctrl Pts',(42.30398588289,4.66632678615171,-9.74462402014482));
#69123=CARTESIAN_POINT('Ctrl Pts',(42.2941108707343,4.67264747979671,-9.84124132004542));
#69124=CARTESIAN_POINT('Ctrl Pts',(42.2842199896438,4.67897833066205,-9.93801388189351));
#69125=CARTESIAN_POINT('Ctrl Pts',(42.2697968477625,4.68530918152739,-10.0342040482199));
#69126=CARTESIAN_POINT('Ctrl Pts',(42.2509464970116,4.69164003239273,-10.1293642322908));
#69127=CARTESIAN_POINT('Ctrl Pts',(42.2399646464367,4.69532826393463,-10.184802719137));
#69128=CARTESIAN_POINT('Ctrl Pts',(42.2274811480986,4.69901649547654,-10.2398918777559));
#69129=CARTESIAN_POINT('Ctrl Pts',(42.2135244854079,4.70270472701844,-10.2945458587682));
#69130=CARTESIAN_POINT('Ctrl Pts',(42.1895563876361,4.70903861185608,-10.3884043971266));
#69131=CARTESIAN_POINT('Ctrl Pts',(42.1611576037167,4.71537249669373,-10.4813048909988));
#69132=CARTESIAN_POINT('Ctrl Pts',(42.1284209443368,4.72170638153138,-10.5727983707133));
#69133=CARTESIAN_POINT('Ctrl Pts',(42.0957283609005,4.72803173856088,-10.6641686655481));
#69134=CARTESIAN_POINT('Ctrl Pts',(42.0587096562478,4.73435709559038,-10.7541353033115));
#69135=CARTESIAN_POINT('Ctrl Pts',(42.0175081333417,4.74068245261988,-10.8422617702846));
#69136=CARTESIAN_POINT('Ctrl Pts',(41.9763497712833,4.74700118349209,-10.9302959199659));
#69137=CARTESIAN_POINT('Ctrl Pts',(41.9310174863046,4.7533199143643,-11.0164933373018));
#69138=CARTESIAN_POINT('Ctrl Pts',(41.8817032966851,4.75963864523652,-11.1004358385692));
#69139=CARTESIAN_POINT('Ctrl Pts',(41.8324242224,4.76595287670706,-11.1843185665945));
#69140=CARTESIAN_POINT('Ctrl Pts',(41.7791691013338,4.7722671081776,-11.2659491949411));
#69141=CARTESIAN_POINT('Ctrl Pts',(41.7221762247401,4.77858133964815,-11.3449334450072));
#69142=CARTESIAN_POINT('Ctrl Pts',(41.6652040276702,4.78489328003764,-11.4238890361114));
#69143=CARTESIAN_POINT('Ctrl Pts',(41.6044970254573,4.79120522042714,-11.5001998028149));
#69144=CARTESIAN_POINT('Ctrl Pts',(41.5403367113354,4.79751716081663,-11.573500605437));
#69145=CARTESIAN_POINT('Ctrl Pts',(41.4761823176237,4.80382851877014,-11.6467946442079));
#69146=CARTESIAN_POINT('Ctrl Pts',(41.4085755336306,4.81013987672365,-11.7170789423427));
#69147=CARTESIAN_POINT('Ctrl Pts',(41.3378373137875,4.81645123467716,-11.7840224152668));
#69148=CARTESIAN_POINT('Ctrl Pts',(41.267086482095,4.82276371787663,-11.8509778234785));
#69149=CARTESIAN_POINT('Ctrl Pts',(41.1932034232146,4.82907620107611,-11.9145909230486));
#69150=CARTESIAN_POINT('Ctrl Pts',(41.1165442418502,4.83538868427558,-11.9745691094417));
#69151=CARTESIAN_POINT('Ctrl Pts',(41.0398034158875,4.8417078904813,-12.0346111746142));
#69152=CARTESIAN_POINT('Ctrl Pts',(40.9602809094415,4.84802709668702,-12.0910103279271));
#69153=CARTESIAN_POINT('Ctrl Pts',(40.8783638840763,4.85434630289274,-12.1435158631424));
#69154=CARTESIAN_POINT('Ctrl Pts',(40.7963990384143,4.86066919803022,-12.1960520492543));
#69155=CARTESIAN_POINT('Ctrl Pts',(40.7120372688379,4.8669920931677,-12.2446898728526));
#69156=CARTESIAN_POINT('Ctrl Pts',(40.6256907113392,4.87331498830518,-12.2892244207917));
#69157=CARTESIAN_POINT('Ctrl Pts',(40.5392061685772,4.87964798768277,-12.3338301367251));
#69158=CARTESIAN_POINT('Ctrl Pts',(40.4507309016318,4.88598098706036,-12.3743193015679));
#69159=CARTESIAN_POINT('Ctrl Pts',(40.3606973525431,4.89231398643795,-12.4105350125582));
#69160=CARTESIAN_POINT('Ctrl Pts',(40.3085863043348,4.89597950045144,-12.4314965172464));
#69161=CARTESIAN_POINT('Ctrl Pts',(40.2559535325021,4.89964501446493,-12.4510273184645));
#69162=CARTESIAN_POINT('Ctrl Pts',(40.2028848447455,4.90331052847842,-12.4691047265815));
#69163=CARTESIAN_POINT('Ctrl Pts',(40.1111819264513,4.90964455229351,-12.500342564742));
#69164=CARTESIAN_POINT('Ctrl Pts',(40.0178595226294,4.9159785761086,-12.5273458107243));
#69165=CARTESIAN_POINT('Ctrl Pts',(39.9233444150091,4.92231259992369,-12.5499468607192));
#69166=CARTESIAN_POINT('Ctrl Pts',(39.828956215711,4.92863811885151,-12.5725175635939));
#69167=CARTESIAN_POINT('Ctrl Pts',(39.7333789172025,4.93496363777933,-12.5906977181596));
#69168=CARTESIAN_POINT('Ctrl Pts',(39.6370564555585,4.94128915670716,-12.6043688164224));
#69169=CARTESIAN_POINT('Ctrl Pts',(39.5408345538429,4.9476080718406,-12.618025642161));
#69170=CARTESIAN_POINT('Ctrl Pts',(39.4438694660887,4.95392698697405,-12.6271827092045));
#69171=CARTESIAN_POINT('Ctrl Pts',(39.3466163926442,4.96024590210749,-12.631772326114));
#69172=CARTESIAN_POINT('Ctrl Pts',(39.2494320730791,4.96656035003066,-12.6363586983552));
#69173=CARTESIAN_POINT('Ctrl Pts',(39.151960607948,4.97287479795382,-12.636384019408));
#69174=CARTESIAN_POINT('Ctrl Pts',(39.0546624609442,4.97918924587698,-12.6318324146373));
#69175=CARTESIAN_POINT('Ctrl Pts',(38.9573993122324,4.98550142248359,-12.6272824470858));
#69176=CARTESIAN_POINT('Ctrl Pts',(38.8603097939336,4.9918135990902,-12.6181588454324));
#69177=CARTESIAN_POINT('Ctrl Pts',(38.763853569696,4.99812577569682,-12.6044978396214));
#69178=CARTESIAN_POINT('Ctrl Pts',(38.6674059501631,5.0044373892043,-12.5908380524869));
#69179=CARTESIAN_POINT('Ctrl Pts',(38.5715919450938,5.01074900271178,-12.5726417274938));
#69180=CARTESIAN_POINT('Ctrl Pts',(38.4768642573544,5.01706061621927,-12.5499967521649));
#69181=CARTESIAN_POINT('Ctrl Pts',(38.3821193973506,5.02337337389799,-12.527347671748));
#69182=CARTESIAN_POINT('Ctrl Pts',(38.2884616708947,5.02968613157671,-12.5002484409021));
#69183=CARTESIAN_POINT('Ctrl Pts',(38.1963307592554,5.03599888925543,-12.4688374119647));
#69184=CARTESIAN_POINT('Ctrl Pts',(38.1041013369121,5.04231839683157,-12.4373927968778));
#69185=CARTESIAN_POINT('Ctrl Pts',(38.0134024030467,5.04863790440772,-12.4016273205991));
#69186=CARTESIAN_POINT('Ctrl Pts',(37.9246555201598,5.05495741198386,-12.3617282405336));
#69187=CARTESIAN_POINT('Ctrl Pts',(37.8358566132894,5.06128062409527,-12.3218057713754));
#69188=CARTESIAN_POINT('Ctrl Pts',(37.7490124256655,5.06760383620668,-12.277745070888));
#69189=CARTESIAN_POINT('Ctrl Pts',(37.6645198138637,5.07392704831809,-12.2297793349704));
#69190=CARTESIAN_POINT('Ctrl Pts',(37.5798919025376,5.08026038590169,-12.1817367906655));
#69191=CARTESIAN_POINT('Ctrl Pts',(37.4976234556511,5.08659372348529,-12.1297769575985));
#69192=CARTESIAN_POINT('Ctrl Pts',(37.4180822176767,5.09292706106889,-12.0741762728262));
#69193=CARTESIAN_POINT('Ctrl Pts',(37.3720769827445,5.09659015069206,-12.0420178273395));
#69194=CARTESIAN_POINT('Ctrl Pts',(37.3269834651792,5.10025324031523,-12.0086421846129));
#69195=CARTESIAN_POINT('Ctrl Pts',(37.282867422968,5.1039163299384,-11.9741086817417));
#69196=CARTESIAN_POINT('Ctrl Pts',(37.2075507939534,5.11017009950536,-11.9151517378737));
#69197=CARTESIAN_POINT('Ctrl Pts',(37.1348090320424,5.11642386907233,-11.852601735732));
#69198=CARTESIAN_POINT('Ctrl Pts',(37.0650108769628,5.12267763863929,-11.7867144155293));
#69199=CARTESIAN_POINT('Ctrl Pts',(36.9953073460977,5.12892293007339,-11.7209164176863));
#69200=CARTESIAN_POINT('Ctrl Pts',(36.9285398189936,5.13516822150749,-11.6517903943124));
#69201=CARTESIAN_POINT('Ctrl Pts',(36.865045801067,5.14141351294159,-11.5796336758131));
#69202=CARTESIAN_POINT('Ctrl Pts',(36.8016225896781,5.14765183982254,-11.5075574242235));
#69203=CARTESIAN_POINT('Ctrl Pts',(36.741465925958,5.15389016670348,-11.4324575313063));
#69204=CARTESIAN_POINT('Ctrl Pts',(36.6848771847878,5.16012849358443,-11.3546687889613));
#69205=CARTESIAN_POINT('Ctrl Pts',(36.6283229200577,5.16636301979234,-11.2769274390632));
#69206=CARTESIAN_POINT('Ctrl Pts',(36.5753325256378,5.17259754600025,-11.1965008544694));
#69207=CARTESIAN_POINT('Ctrl Pts',(36.5261671199786,5.17883207220816,-11.1137568670557));
#69208=CARTESIAN_POINT('Ctrl Pts',(36.4770175409623,5.18506459148419,-11.0310395154344));
#69209=CARTESIAN_POINT('Ctrl Pts',(36.4316907342995,5.19129711076023,-10.9460066287224));
#69210=CARTESIAN_POINT('Ctrl Pts',(36.3904038200082,5.19752963003626,-10.8590539562835));
#69211=CARTESIAN_POINT('Ctrl Pts',(36.3491183334319,5.20376193378974,-10.7721042906964));
#69212=CARTESIAN_POINT('Ctrl Pts',(36.3118726529036,5.20999423754321,-10.6832353778791));
#69213=CARTESIAN_POINT('Ctrl Pts',(36.2788368271283,5.21622654129669,-10.5928653334379));
#69214=CARTESIAN_POINT('Ctrl Pts',(36.2457731565261,5.22246409805704,-10.5024191190146));
#69215=CARTESIAN_POINT('Ctrl Pts',(36.2169265823318,5.22870165481739,-10.4104696687024));
#69216=CARTESIAN_POINT('Ctrl Pts',(36.192417926031,5.23493921157774,-10.3174523463531));
#69217=CARTESIAN_POINT('Ctrl Pts',(36.1678988187396,5.24117942815947,-10.2243953595211));
#69218=CARTESIAN_POINT('Ctrl Pts',(36.1477214069243,5.24741964474119,-10.1302700334956));
#69219=CARTESIAN_POINT('Ctrl Pts',(36.1319553452258,5.25365986132292,-10.0355219380313));
#69220=CARTESIAN_POINT('Ctrl Pts',(36.1161650415883,5.25990967287845,-9.94062815764062));
#69221=CARTESIAN_POINT('Ctrl Pts',(36.1047996883591,5.26615948443398,-9.84511014177736));
#69222=CARTESIAN_POINT('Ctrl Pts',(36.0978770168524,5.27240929598951,-9.7494184714492));
#69223=CARTESIAN_POINT('Ctrl Pts',(36.0924270076094,5.27732958300767,-9.67408332268855));
#69224=CARTESIAN_POINT('Ctrl Pts',(36.0897295006916,5.28224987002584,-9.59864067588427));
#69225=CARTESIAN_POINT('Ctrl Pts',(36.0897704597331,5.287170157044,-9.52330892006468));
#69226=CARTESIAN_POINT('Origin',(39.2,8.05522481984854,-9.525));
#69227=CARTESIAN_POINT('',(37.4444040758239,-12.75,-7.88069592367579));
#69228=CARTESIAN_POINT('Ctrl Pts',(36.9580196848654,-11.5570870138823,-8.65357747851634));
#69229=CARTESIAN_POINT('Ctrl Pts',(36.9542985205578,-11.557947724717,-8.663151223653));
#69230=CARTESIAN_POINT('Ctrl Pts',(36.9506385991756,-11.5588049799687,-8.67274901000278));
#69231=CARTESIAN_POINT('Ctrl Pts',(36.9352241227137,-11.5624633818171,-8.71396307409524));
#69232=CARTESIAN_POINT('Ctrl Pts',(36.9240730287327,-11.5652325766466,-8.7458033405071));
#69233=CARTESIAN_POINT('Ctrl Pts',(36.8979053716304,-11.5720812690608,-8.82588294209961));
#69234=CARTESIAN_POINT('Ctrl Pts',(36.8837311827434,-11.5761258191705,-8.87438192035425));
#69235=CARTESIAN_POINT('Ctrl Pts',(36.8423114898232,-11.5892702188433,-9.03469727488616));
#69236=CARTESIAN_POINT('Ctrl Pts',(36.8215583821953,-11.5982148740058,-9.14802569727867));
#69237=CARTESIAN_POINT('Ctrl Pts',(36.7956053791119,-11.616882243002,-9.38433838841497));
#69238=CARTESIAN_POINT('Ctrl Pts',(36.7915623109317,-11.6265924990067,-9.50709725972053));
#69239=CARTESIAN_POINT('Ctrl Pts',(36.7982888662892,-11.6392030548517,-9.6616087596262));
#69240=CARTESIAN_POINT('Ctrl Pts',(36.8003201963094,-11.6418316248682,-9.69356739931507));
#69241=CARTESIAN_POINT('Ctrl Pts',(36.8047004161722,-11.6461782353672,-9.74594032721957));
#69242=CARTESIAN_POINT('Ctrl Pts',(36.8066740602457,-11.6478845913681,-9.76638271696718));
#69243=CARTESIAN_POINT('Ctrl Pts',(36.8110469375735,-11.6512389786805,-9.80632190538292));
#69244=CARTESIAN_POINT('Ctrl Pts',(36.813423732069,-11.6528861841482,-9.82581957615525));
#69245=CARTESIAN_POINT('Ctrl Pts',(36.8196798901244,-11.6568445914328,-9.87238566856782));
#69246=CARTESIAN_POINT('Ctrl Pts',(36.8237824919044,-11.6591625577661,-9.89942068546272));
#69247=CARTESIAN_POINT('Ctrl Pts',(36.8403323400121,-11.6676229754151,-9.99720995508508));
#69248=CARTESIAN_POINT('Ctrl Pts',(36.8554854622904,-11.6738473742196,-10.0674601710637));
#69249=CARTESIAN_POINT('Ctrl Pts',(36.9045075744349,-11.6907706574786,-10.2538200777191));
#69250=CARTESIAN_POINT('Ctrl Pts',(36.9440231356249,-11.7016071449136,-10.3682238871745));
#69251=CARTESIAN_POINT('Ctrl Pts',(37.0387193834495,-11.7230626201159,-10.5873618517877));
#69252=CARTESIAN_POINT('Ctrl Pts',(37.0933714377716,-11.7336507598302,-10.6919912608123));
#69253=CARTESIAN_POINT('Ctrl Pts',(37.1689967801852,-11.7461543447625,-10.8140062125811));
#69254=CARTESIAN_POINT('Ctrl Pts',(37.1828608603123,-11.7483726700347,-10.835595645731));
#69255=CARTESIAN_POINT('Ctrl Pts',(37.2042927663781,-11.7516887121019,-10.8678238101491));
#69256=CARTESIAN_POINT('Ctrl Pts',(37.2116055136549,-11.7528012424656,-10.8786286560699));
#69257=CARTESIAN_POINT('Ctrl Pts',(37.2251723074942,-11.7548302060971,-10.8983268760363));
#69258=CARTESIAN_POINT('Ctrl Pts',(37.2313990079435,-11.7557482382746,-10.9072377754715));
#69259=CARTESIAN_POINT('Ctrl Pts',(37.2460845102195,-11.7578832488629,-10.927953339875));
#69260=CARTESIAN_POINT('Ctrl Pts',(37.2545901159273,-11.7590970984721,-10.9397240829371));
#69261=CARTESIAN_POINT('Ctrl Pts',(37.2832570807654,-11.7631162780797,-10.9786482515421));
#69262=CARTESIAN_POINT('Ctrl Pts',(37.3038856051206,-11.7658927168098,-11.0054550667182));
#69263=CARTESIAN_POINT('Ctrl Pts',(37.356826811098,-11.7727628157233,-11.0713294528352));
#69264=CARTESIAN_POINT('Ctrl Pts',(37.3898228482146,-11.7768212967455,-11.1098285859429));
#69265=CARTESIAN_POINT('Ctrl Pts',(37.551333793215,-11.7958314022693,-11.2866445501831));
#69266=CARTESIAN_POINT('Ctrl Pts',(37.6946177563593,-11.8103250271822,-11.4105552888389));
#69267=CARTESIAN_POINT('Ctrl Pts',(37.9014668303761,-11.8303116032354,-11.5506831630786));
#69268=CARTESIAN_POINT('Ctrl Pts',(37.9532960784354,-11.8352462138195,-11.582986596297));
#69269=CARTESIAN_POINT('Ctrl Pts',(38.0271003349675,-11.8422149766932,-11.6251746770269));
#69270=CARTESIAN_POINT('Ctrl Pts',(38.0480824477401,-11.8441897623893,-11.6367559441532));
#69271=CARTESIAN_POINT('Ctrl Pts',(38.0865951250313,-11.8478054532929,-11.6572686209035));
#69272=CARTESIAN_POINT('Ctrl Pts',(38.1040691245242,-11.8494426482533,-11.6663022568855));
#69273=CARTESIAN_POINT('Ctrl Pts',(38.139724365488,-11.8527779100226,-11.6841844092006));
#69274=CARTESIAN_POINT('Ctrl Pts',(38.1579102718375,-11.8544762643177,-11.6930199904905));
#69275=CARTESIAN_POINT('Ctrl Pts',(38.2036633044304,-11.8587435547332,-11.7145403418167));
#69276=CARTESIAN_POINT('Ctrl Pts',(38.2313623233122,-11.861322076058,-11.7269342837391));
#69277=CARTESIAN_POINT('Ctrl Pts',(38.3527240647931,-11.8726045705189,-11.77850467994));
#69278=CARTESIAN_POINT('Ctrl Pts',(38.4485660379483,-11.8814821245231,-11.8122474505715));
#69279=CARTESIAN_POINT('Ctrl Pts',(38.6374174237369,-11.8989100996508,-11.8655833436182));
#69280=CARTESIAN_POINT('Ctrl Pts',(38.7300329845701,-11.9074273574035,-11.8859232634944));
#69281=CARTESIAN_POINT('Ctrl Pts',(38.9293821509118,-11.9255604574588,-11.9175069451102));
#69282=CARTESIAN_POINT('Ctrl Pts',(39.0361764765007,-11.9351562801561,-11.9271844909143));
#69283=CARTESIAN_POINT('Ctrl Pts',(39.1690701439768,-11.9467353044458,-11.9303195787957));
#69284=CARTESIAN_POINT('Ctrl Pts',(39.1948794316064,-11.948966857592,-11.930513016968));
#69285=CARTESIAN_POINT('Ctrl Pts',(39.2337790608165,-11.9522997847906,-11.9301784337741));
#69286=CARTESIAN_POINT('Ctrl Pts',(39.2468690871447,-11.9534161388058,-11.9299589677455));
#69287=CARTESIAN_POINT('Ctrl Pts',(39.2708594388396,-11.9554518212718,-11.9293607920759));
#69288=CARTESIAN_POINT('Ctrl Pts',(39.2817594849541,-11.9563727568259,-11.9290148242498));
#69289=CARTESIAN_POINT('Ctrl Pts',(39.3072141849367,-11.958514509633,-11.9280335564926));
#69290=CARTESIAN_POINT('Ctrl Pts',(39.3217659933897,-11.9597321884348,-11.9273401572075));
#69291=CARTESIAN_POINT('Ctrl Pts',(39.370164713456,-11.9637625725864,-11.9245930216666));
#69292=CARTESIAN_POINT('Ctrl Pts',(39.4039764097716,-11.9665463685107,-11.9219557087851));
#69293=CARTESIAN_POINT('Ctrl Pts',(39.4883340751097,-11.9734380490757,-11.9135776308246));
#69294=CARTESIAN_POINT('Ctrl Pts',(39.5387764133877,-11.9775106941544,-11.9069468858319));
#69295=CARTESIAN_POINT('Ctrl Pts',(39.7027259655225,-11.9907012891413,-11.8800809894981));
#69296=CARTESIAN_POINT('Ctrl Pts',(39.8149949525048,-11.9996664520673,-11.8532876252156));
#69297=CARTESIAN_POINT('Ctrl Pts',(40.039942156662,-12.0182052933104,-11.7821892860208));
#69298=CARTESIAN_POINT('Ctrl Pts',(40.1520570783395,-12.0277635842373,-11.7372358215556));
#69299=CARTESIAN_POINT('Ctrl Pts',(40.2890355860524,-12.040209152254,-11.6699657473404));
#69300=CARTESIAN_POINT('Ctrl Pts',(40.3174678003802,-12.0428358696885,-11.6552915496957));
#69301=CARTESIAN_POINT('Ctrl Pts',(40.3636886544239,-12.047183785104,-11.6302565078068));
#69302=CARTESIAN_POINT('Ctrl Pts',(40.3816526497544,-12.0488934035409,-11.6202262905939));
#69303=CARTESIAN_POINT('Ctrl Pts',(40.4165784399783,-12.0522577458837,-11.6001334235476));
#69304=CARTESIAN_POINT('Ctrl Pts',(40.433549542327,-12.0539116748263,-11.5900901441492));
#69305=CARTESIAN_POINT('Ctrl Pts',(40.4739117351212,-12.0578926762898,-11.5655292629567));
#69306=CARTESIAN_POINT('Ctrl Pts',(40.4971802652047,-12.060226624361,-11.5508168738512));
#69307=CARTESIAN_POINT('Ctrl Pts',(40.5811334762645,-12.0687951380098,-11.4956949233973));
#69308=CARTESIAN_POINT('Ctrl Pts',(40.6402187445438,-12.0751140828492,-11.4529356275011));
#69309=CARTESIAN_POINT('Ctrl Pts',(40.7916473972912,-12.0921134150615,-11.3324994366157));
#69310=CARTESIAN_POINT('Ctrl Pts',(40.8802411136818,-12.1029264986396,-11.2504505332821));
#69311=CARTESIAN_POINT('Ctrl Pts',(41.0419365771646,-12.1242778842078,-11.0763907470312));
#69312=CARTESIAN_POINT('Ctrl Pts',(41.1152197595652,-12.134785735661,-10.9849598283339));
#69313=CARTESIAN_POINT('Ctrl Pts',(41.1961239216403,-12.1472166947,-10.8673867156619));
#69314=CARTESIAN_POINT('Ctrl Pts',(41.2103466305909,-12.1494378545524,-10.8459918208529));
#69315=CARTESIAN_POINT('Ctrl Pts',(41.2312801438623,-12.1527579369728,-10.8133805766081));
#69316=CARTESIAN_POINT('Ctrl Pts',(41.2382462108354,-12.1538716991374,-10.8023315707104));
#69317=CARTESIAN_POINT('Ctrl Pts',(41.250820859159,-12.1558979985074,-10.7820218529997));
#69318=CARTESIAN_POINT('Ctrl Pts',(41.2564572447194,-12.156812192493,-10.7727795271475));
#69319=CARTESIAN_POINT('Ctrl Pts',(41.2694441309307,-12.1589328417281,-10.751157085998));
#69320=CARTESIAN_POINT('Ctrl Pts',(41.2767461628105,-12.1601362415648,-10.7387485810905));
#69321=CARTESIAN_POINT('Ctrl Pts',(41.3006340515201,-12.1641129604191,-10.697308565048));
#69322=CARTESIAN_POINT('Ctrl Pts',(41.316726997804,-12.1668578200936,-10.6679951637524));
#69323=CARTESIAN_POINT('Ctrl Pts',(41.3553199040437,-12.1736356949638,-10.5940851516062));
#69324=CARTESIAN_POINT('Ctrl Pts',(41.3770526974665,-12.1776343025331,-10.5491041302539));
#69325=CARTESIAN_POINT('Ctrl Pts',(41.4797329462882,-12.1976687799414,-10.3185142802863));
#69326=CARTESIAN_POINT('Ctrl Pts',(41.5384117329997,-12.2131619472121,-10.1238994860267));
#69327=CARTESIAN_POINT('Ctrl Pts',(41.5810553100192,-12.233789200857,-9.87053374643876));
#69328=CARTESIAN_POINT('Ctrl Pts',(41.5882662592702,-12.2382042405221,-9.81654993145718));
#69329=CARTESIAN_POINT('Ctrl Pts',(41.5960536419447,-12.2446847965724,-9.73802254120953));
#69330=CARTESIAN_POINT('Ctrl Pts',(41.598096524861,-12.2467050853659,-9.7136388749689));
#69331=CARTESIAN_POINT('Ctrl Pts',(41.6010772989839,-12.2503306552236,-9.67008289410366));
#69332=CARTESIAN_POINT('Ctrl Pts',(41.602158361476,-12.2519313497961,-9.6509222097963));
#69333=CARTESIAN_POINT('Ctrl Pts',(41.6039573638322,-12.2553278036847,-9.61042599211918));
#69334=CARTESIAN_POINT('Ctrl Pts',(41.6046207670379,-12.2571251179227,-9.58908986309842));
#69335=CARTESIAN_POINT('Ctrl Pts',(41.6056458849351,-12.2620061855472,-9.53141740654411));
#69336=CARTESIAN_POINT('Ctrl Pts',(41.6054682928594,-12.2651062661373,-9.49507863599632));
#69337=CARTESIAN_POINT('Ctrl Pts',(41.6009106761434,-12.2793409981676,-9.32964044030008));
#69338=CARTESIAN_POINT('Ctrl Pts',(41.5869597132131,-12.2907587977928,-9.20104068670405));
#69339=CARTESIAN_POINT('Ctrl Pts',(41.5355817193552,-12.3153184634751,-8.93175332990722));
#69340=CARTESIAN_POINT('Ctrl Pts',(41.4955760701008,-12.328453828886,-8.79204859779349));
#69341=CARTESIAN_POINT('Ctrl Pts',(41.4298817969084,-12.3444564890413,-8.62231109335828));
#69342=CARTESIAN_POINT('Ctrl Pts',(41.4157415344472,-12.3476791858735,-8.58813822961163));
#69343=CARTESIAN_POINT('Ctrl Pts',(41.3952154240443,-12.3520573452491,-8.54160032733227));
#69344=CARTESIAN_POINT('Ctrl Pts',(41.3895029488942,-12.3532466731366,-8.52894651786372));
#69345=CARTESIAN_POINT('Ctrl Pts',(41.3790550832277,-12.3553697599223,-8.50632753749832));
#69346=CARTESIAN_POINT('Ctrl Pts',(41.3743601148742,-12.3563057991912,-8.49634419965886));
#69347=CARTESIAN_POINT('Ctrl Pts',(41.3644268802704,-12.3582487602414,-8.47559418640268));
#69348=CARTESIAN_POINT('Ctrl Pts',(41.3591766728751,-12.3592549599153,-8.46483378841859));
#69349=CARTESIAN_POINT('Ctrl Pts',(41.3447819967961,-12.3619597428809,-8.43588217296116));
#69350=CARTESIAN_POINT('Ctrl Pts',(41.3354862753539,-12.3636495283759,-8.4177665526253));
#69351=CARTESIAN_POINT('Ctrl Pts',(41.2761571438391,-12.3741028293089,-8.30567261891157));
#69352=CARTESIAN_POINT('Ctrl Pts',(41.2201527380048,-12.3825522531078,-8.21497037392307));
#69353=CARTESIAN_POINT('Ctrl Pts',(41.0492926771049,-12.4056986323015,-7.97541328310945));
#69354=CARTESIAN_POINT('Ctrl Pts',(40.9227637462089,-12.4202092474583,-7.83586401618057));
#69355=CARTESIAN_POINT('Ctrl Pts',(40.7532744278501,-12.4384258546061,-7.68799838300081));
#69356=CARTESIAN_POINT('Ctrl Pts',(40.724684921271,-12.4414604690287,-7.66420124951601));
#69357=CARTESIAN_POINT('Ctrl Pts',(40.6769628977446,-12.4464743624698,-7.62631699612608));
#69358=CARTESIAN_POINT('Ctrl Pts',(40.6581523369864,-12.4484380790744,-7.61183293190663));
#69359=CARTESIAN_POINT('Ctrl Pts',(40.6236715780633,-12.4520173563612,-7.58608679145969));
#69360=CARTESIAN_POINT('Ctrl Pts',(40.6080741642415,-12.4536291199562,-7.57473019949258));
#69361=CARTESIAN_POINT('Ctrl Pts',(40.5739516915968,-12.4571406310443,-7.55050808214353));
#69362=CARTESIAN_POINT('Ctrl Pts',(40.5553790834878,-12.4590428391348,-7.53771314334845));
#69363=CARTESIAN_POINT('Ctrl Pts',(40.5020877305708,-12.4644773917166,-7.50209449756052));
#69364=CARTESIAN_POINT('Ctrl Pts',(40.4669555296242,-12.4680323829678,-7.47990773785733));
#69365=CARTESIAN_POINT('Ctrl Pts',(40.3852718029824,-12.4762415433406,-7.43123530336788));
#69366=CARTESIAN_POINT('Ctrl Pts',(40.338376337735,-12.4809144674893,-7.40537307695799));
#69367=CARTESIAN_POINT('Ctrl Pts',(40.1897859182684,-12.4955986458467,-7.32978110848318));
#69368=CARTESIAN_POINT('Ctrl Pts',(40.0854237972828,-12.5057474472962,-7.28565134676141));
#69369=CARTESIAN_POINT('Ctrl Pts',(39.8697500032924,-12.5262173819618,-7.21189339745932));
#69370=CARTESIAN_POINT('Ctrl Pts',(39.7586152099203,-12.5365129999654,-7.18256924199442));
#69371=CARTESIAN_POINT('Ctrl Pts',(39.620464619881,-12.5487532419623,-7.15651373448423));
#69372=CARTESIAN_POINT('Ctrl Pts',(39.595051947083,-12.5509817951602,-7.15214269141626));
#69373=CARTESIAN_POINT('Ctrl Pts',(39.5565743628291,-12.5543169193844,-7.14615979900953));
#69374=CARTESIAN_POINT('Ctrl Pts',(39.5435594968635,-12.5554382780791,-7.14424531398136));
#69375=CARTESIAN_POINT('Ctrl Pts',(39.5206185163224,-12.5574023128386,-7.14106274794722));
#69376=CARTESIAN_POINT('Ctrl Pts',(39.5106996979998,-12.558247301484,-7.13974974928353));
#69377=CARTESIAN_POINT('Ctrl Pts',(39.4865116585258,-12.5602981459257,-7.13670131409115));
#69378=CARTESIAN_POINT('Ctrl Pts',(39.4722345493033,-12.561500471632,-7.13503181508051));
#69379=CARTESIAN_POINT('Ctrl Pts',(39.4264324052607,-12.565333948092,-7.13009169993544));
#69380=CARTESIAN_POINT('Ctrl Pts',(39.3948557097709,-12.5679409247018,-7.12731592313843));
#69381=CARTESIAN_POINT('Ctrl Pts',(39.3172598772165,-12.574280245338,-7.1220380347081));
#69382=CARTESIAN_POINT('Ctrl Pts',(39.2712048696586,-12.5779852351098,-7.12023253672798));
#69383=CARTESIAN_POINT('Ctrl Pts',(39.0438074194755,-12.5961208970095,-7.11785732402667));
#69384=CARTESIAN_POINT('Ctrl Pts',(38.8628584655863,-12.6101013178022,-7.13647084063742));
#69385=CARTESIAN_POINT('Ctrl Pts',(38.6215062701294,-12.6298519186568,-7.18929492595988));
#69386=CARTESIAN_POINT('Ctrl Pts',(38.5579062998381,-12.6351596976618,-7.20597272850991));
#69387=CARTESIAN_POINT('Ctrl Pts',(38.4715313540076,-12.6425645278997,-7.2324484318039));
#69388=CARTESIAN_POINT('Ctrl Pts',(38.4481020751502,-12.6445932590993,-7.24002545235607));
#69389=CARTESIAN_POINT('Ctrl Pts',(38.4075512877431,-12.6481424746626,-7.25383075134866));
#69390=CARTESIAN_POINT('Ctrl Pts',(38.3903762332926,-12.6496577159095,-7.25989646229953));
#69391=CARTESIAN_POINT('Ctrl Pts',(38.3543861507293,-12.6528593266299,-7.27306869023705));
#69392=CARTESIAN_POINT('Ctrl Pts',(38.3355881555246,-12.6545469494113,-7.28021726720911));
#69393=CARTESIAN_POINT('Ctrl Pts',(38.2902116694931,-12.6586596465065,-7.29812768702052));
#69394=CARTESIAN_POINT('Ctrl Pts',(38.2637323861268,-12.661092416769,-7.30913043956218));
#69395=CARTESIAN_POINT('Ctrl Pts',(38.1634397132502,-12.6704378217172,-7.35292291351868));
#69396=CARTESIAN_POINT('Ctrl Pts',(38.0911066283019,-12.6774549325123,-7.3889455844176));
#69397=CARTESIAN_POINT('Ctrl Pts',(37.9220293917355,-12.6945533234796,-7.48405211883646));
#69398=CARTESIAN_POINT('Ctrl Pts',(37.827381440119,-12.7047153723466,-7.54646748654571));
#69399=CARTESIAN_POINT('Ctrl Pts',(37.6505455582212,-12.7247361284071,-7.68189478509101));
#69400=CARTESIAN_POINT('Ctrl Pts',(37.568241289525,-12.734570146411,-7.75434644945453));
#69401=CARTESIAN_POINT('Ctrl Pts',(37.4771610585272,-12.7458843881036,-7.84628790424061));
#69402=CARTESIAN_POINT('Ctrl Pts',(37.4633423278758,-12.7476136262563,-7.86058763598447));
#69403=CARTESIAN_POINT('Ctrl Pts',(37.4479329618307,-12.7495548577216,-7.87693425832693));
#69404=CARTESIAN_POINT('Ctrl Pts',(37.4461670091522,-12.7497775229632,-7.87881366928609));
#69405=CARTESIAN_POINT('Ctrl Pts',(37.4444040758239,-12.75,-7.88069592367579));
#69406=CARTESIAN_POINT('',(40.3181783974771,-12.75,-7.39532161681262));
#69407=CARTESIAN_POINT('Origin',(39.2,-12.75,-9.525));
#69408=CARTESIAN_POINT('',(36.7946210610025,-11.8952248199035,-9.52725925364505));
#69409=CARTESIAN_POINT('Ctrl Pts',(36.7946210610025,-11.8952248199035,-9.52725925364505));
#69410=CARTESIAN_POINT('Ctrl Pts',(36.7947186589564,-11.9039501489463,-9.63116970366884));
#69411=CARTESIAN_POINT('Ctrl Pts',(36.8015536899245,-11.912675477989,-9.73478128463119));
#69412=CARTESIAN_POINT('Ctrl Pts',(36.8149857633701,-11.9214008070318,-9.83734601882026));
#69413=CARTESIAN_POINT('Ctrl Pts',(36.8284178368158,-11.9301261360746,-9.93991075300932));
#69414=CARTESIAN_POINT('Ctrl Pts',(36.8484467666642,-11.9388514651173,-10.0414289472041));
#69415=CARTESIAN_POINT('Ctrl Pts',(36.8748810013598,-11.9475767941601,-10.1411773986139));
#69416=CARTESIAN_POINT('Ctrl Pts',(36.8953762218173,-11.9543417920635,-10.2185152343967));
#69417=CARTESIAN_POINT('Ctrl Pts',(36.9197715899412,-11.961106789967,-10.2949704447773));
#69418=CARTESIAN_POINT('Ctrl Pts',(36.9479738992011,-11.9678717878704,-10.3701221129046));
#69419=CARTESIAN_POINT('Ctrl Pts',(36.9761359648038,-11.9746271323709,-10.445166542368));
#69420=CARTESIAN_POINT('Ctrl Pts',(37.0080940195322,-11.9813824768713,-10.5189106928252));
#69421=CARTESIAN_POINT('Ctrl Pts',(37.0437045982079,-11.9881378213718,-10.5909470364939));
#69422=CARTESIAN_POINT('Ctrl Pts',(37.0792739104633,-11.9948853376118,-10.6628999026641));
#69423=CARTESIAN_POINT('Ctrl Pts',(37.1184871288128,-12.0016328538518,-10.7331484813702));
#69424=CARTESIAN_POINT('Ctrl Pts',(37.1611526010783,-12.0083803700919,-10.8013049119667));
#69425=CARTESIAN_POINT('Ctrl Pts',(37.2037909501032,-12.0151235968093,-10.8694180142423));
#69426=CARTESIAN_POINT('Ctrl Pts',(37.2498769501429,-12.0218668235267,-10.9354412162069));
#69427=CARTESIAN_POINT('Ctrl Pts',(37.2991734512255,-12.0286100502441,-10.9990119999084));
#69428=CARTESIAN_POINT('Ctrl Pts',(37.3484536494874,-12.0353510469125,-11.0625617601484));
#69429=CARTESIAN_POINT('Ctrl Pts',(37.4009419555341,-12.0420920435809,-11.1236603462121));
#69430=CARTESIAN_POINT('Ctrl Pts',(37.456359245328,-12.0488330402492,-11.1819761202404));
#69431=CARTESIAN_POINT('Ctrl Pts',(37.5117751102101,-12.0555738635903,-11.2402903948299));
#69432=CARTESIAN_POINT('Ctrl Pts',(37.5701194881866,-12.0623146869315,-11.2958216638355));
#69433=CARTESIAN_POINT('Ctrl Pts',(37.6310754912959,-12.0690555102726,-11.3482742060336));
#69434=CARTESIAN_POINT('Ctrl Pts',(37.6920891892273,-12.0758027137992,-11.400776394533));
#69435=CARTESIAN_POINT('Ctrl Pts',(37.7557190975019,-12.0825499173258,-11.4501937312609));
#69436=CARTESIAN_POINT('Ctrl Pts',(37.8216146789238,-12.0892971208523,-11.4962703647754));
#69437=CARTESIAN_POINT('Ctrl Pts',(37.8875405388679,-12.096047424668,-11.5423681701551));
#69438=CARTESIAN_POINT('Ctrl Pts',(37.9557337525196,-12.1027977284837,-11.5851219661566));
#69439=CARTESIAN_POINT('Ctrl Pts',(38.0258162750942,-12.1095480322993,-11.6243202529786));
#69440=CARTESIAN_POINT('Ctrl Pts',(38.0960202739729,-12.116310036635,-11.6635864834596));
#69441=CARTESIAN_POINT('Ctrl Pts',(38.1681197084572,-12.1230720409707,-11.6992846828844));
#69442=CARTESIAN_POINT('Ctrl Pts',(38.2417136926401,-12.1298340453064,-11.7312502798927));
#69443=CARTESIAN_POINT('Ctrl Pts',(38.3082789127791,-12.1359502287443,-11.7601629284652));
#69444=CARTESIAN_POINT('Ctrl Pts',(38.3760663357046,-12.1420664121822,-11.7860224535644));
#69445=CARTESIAN_POINT('Ctrl Pts',(38.444769163389,-12.1481825956201,-11.8087423952434));
#69446=CARTESIAN_POINT('Ctrl Pts',(38.5207016312425,-12.1549423887456,-11.8338531701462));
#69447=CARTESIAN_POINT('Ctrl Pts',(38.5980250033347,-12.161702181871,-11.8552181838809));
#69448=CARTESIAN_POINT('Ctrl Pts',(38.6763360263255,-12.1684619749965,-11.8726858791319));
#69449=CARTESIAN_POINT('Ctrl Pts',(38.7545372919926,-12.17521229389,-11.8901290924211));
#69450=CARTESIAN_POINT('Ctrl Pts',(38.8337230087439,-12.1819626127834,-11.9036857361839));
#69451=CARTESIAN_POINT('Ctrl Pts',(38.9134737198311,-12.1887129316769,-11.9132536789823));
#69452=CARTESIAN_POINT('Ctrl Pts',(38.993135366358,-12.1954557119017,-11.9228109364263));
#69453=CARTESIAN_POINT('Ctrl Pts',(39.0733602935979,-12.2021984921265,-11.928388291076));
#69454=CARTESIAN_POINT('Ctrl Pts',(39.1537192200424,-12.2089412723513,-11.9299347254773));
#69455=CARTESIAN_POINT('Ctrl Pts',(39.2340291491899,-12.2156799412966,-11.9314802169702));
#69456=CARTESIAN_POINT('Ctrl Pts',(39.314472451482,-12.222418610242,-11.9289996585284));
#69457=CARTESIAN_POINT('Ctrl Pts',(39.3946162739486,-12.2291572791873,-11.9224939938015));
#69458=CARTESIAN_POINT('Ctrl Pts',(39.4747357506959,-12.235893901091,-11.9159903053353));
#69459=CARTESIAN_POINT('Ctrl Pts',(39.5545554650489,-12.2426305229946,-11.9054639766861));
#69460=CARTESIAN_POINT('Ctrl Pts',(39.6336455636557,-12.2493671448983,-11.8909679772815));
#69461=CARTESIAN_POINT('Ctrl Pts',(39.7127358338636,-12.2561037814183,-11.8764719464251));
#69462=CARTESIAN_POINT('Ctrl Pts',(39.7910960279766,-12.2628404179384,-11.8580063129897));
#69463=CARTESIAN_POINT('Ctrl Pts',(39.8683058174271,-12.2695770544585,-11.8356752863164));
#69464=CARTESIAN_POINT('Ctrl Pts',(39.945592404757,-12.2763203916754,-11.8133220477512));
#69465=CARTESIAN_POINT('Ctrl Pts',(40.0217258539102,-12.2830637288924,-11.7870958654182));
#69466=CARTESIAN_POINT('Ctrl Pts',(40.0963009027855,-12.2898070661094,-11.7571508990357));
#69467=CARTESIAN_POINT('Ctrl Pts',(40.1709121142176,-12.2965536732715,-11.7271914118911));
#69468=CARTESIAN_POINT('Ctrl Pts',(40.2439629968681,-12.3033002804336,-11.6935097428903));
#69469=CARTESIAN_POINT('Ctrl Pts',(40.315070495802,-12.3100468875956,-11.6563072828177));
#69470=CARTESIAN_POINT('Ctrl Pts',(40.3863047468538,-12.3168055208697,-11.61903850779));
#69471=CARTESIAN_POINT('Ctrl Pts',(40.4555882903888,-12.3235641541437,-11.5782366376932));
#69472=CARTESIAN_POINT('Ctrl Pts',(40.5225649641608,-12.3303227874178,-11.5341477944577));
#69473=CARTESIAN_POINT('Ctrl Pts',(40.5835617694908,-12.3364779906385,-11.4939953288812));
#69474=CARTESIAN_POINT('Ctrl Pts',(40.6426454031471,-12.3426331938593,-11.4511173257771));
#69475=CARTESIAN_POINT('Ctrl Pts',(40.6995715373854,-12.34878839708,-11.4057280900395));
#69476=CARTESIAN_POINT('Ctrl Pts',(40.7614038109521,-12.3554740822138,-11.3564270145552));
#69477=CARTESIAN_POINT('Ctrl Pts',(40.8209297575957,-12.3621597673477,-11.3039715293003));
#69478=CARTESIAN_POINT('Ctrl Pts',(40.8778053802409,-12.3688454524815,-11.2486072784816));
#69479=CARTESIAN_POINT('Ctrl Pts',(40.9345989025398,-12.3755214867836,-11.1933229463338));
#69480=CARTESIAN_POINT('Ctrl Pts',(40.9887493562766,-12.3821975210857,-11.1351385120028));
#69481=CARTESIAN_POINT('Ctrl Pts',(41.039944698374,-12.3888735553877,-11.0743406505108));
#69482=CARTESIAN_POINT('Ctrl Pts',(41.0912345614128,-12.3955619155191,-11.0134305391371));
#69483=CARTESIAN_POINT('Ctrl Pts',(41.139558021386,-12.4022502756504,-10.9498976508583));
#69484=CARTESIAN_POINT('Ctrl Pts',(41.1846376443065,-12.4089386357818,-10.8840681974064));
#69485=CARTESIAN_POINT('Ctrl Pts',(41.2295564640133,-12.4156031379095,-10.8184735637464));
#69486=CARTESIAN_POINT('Ctrl Pts',(41.2712542670028,-12.4222676400373,-10.7505991077033));
#69487=CARTESIAN_POINT('Ctrl Pts',(41.3094974475735,-12.4289321421651,-10.6807999234647));
#69488=CARTESIAN_POINT('Ctrl Pts',(41.3477297928876,-12.4355947560716,-10.6110205150935));
#69489=CARTESIAN_POINT('Ctrl Pts',(41.3825092293477,-12.442257369978,-10.5393178783685));
#69490=CARTESIAN_POINT('Ctrl Pts',(41.4136472332856,-12.4489199838844,-10.4660732548356));
#69491=CARTESIAN_POINT('Ctrl Pts',(41.4447864767208,-12.4555828630067,-10.3928257156854));
#69492=CARTESIAN_POINT('Ctrl Pts',(41.4722838147315,-12.462245742129,-10.3180365069909));
#69493=CARTESIAN_POINT('Ctrl Pts',(41.4959988032221,-12.4689086212512,-10.2421069934135));
#69494=CARTESIAN_POINT('Ctrl Pts',(41.5198712976804,-12.4756157526919,-10.1656731847775));
#69495=CARTESIAN_POINT('Ctrl Pts',(41.5399108594295,-12.4823228841327,-10.0880843317876));
#69496=CARTESIAN_POINT('Ctrl Pts',(41.5560257516827,-12.4890300155734,-10.0097634493319));
#69497=CARTESIAN_POINT('Ctrl Pts',(41.5720613477695,-12.4957041433923,-9.93182795857612));
#69498=CARTESIAN_POINT('Ctrl Pts',(41.58421080047,-12.5023782712112,-9.85316811001779));
#69499=CARTESIAN_POINT('Ctrl Pts',(41.5924357484883,-12.50905239903,-9.7742070098437));
#69500=CARTESIAN_POINT('Ctrl Pts',(41.600721705169,-12.5157760322817,-9.69466021464805));
#69501=CARTESIAN_POINT('Ctrl Pts',(41.6050246821397,-12.5224996655334,-9.61480817148));
#69502=CARTESIAN_POINT('Ctrl Pts',(41.6053588685275,-12.529223298785,-9.53508255900005));
#69503=CARTESIAN_POINT('Ctrl Pts',(41.6056930549153,-12.5359469320367,-9.45535694652009));
#69504=CARTESIAN_POINT('Ctrl Pts',(41.6020585501418,-12.5426705652883,-9.37575824569389));
#69505=CARTESIAN_POINT('Ctrl Pts',(41.5945222031575,-12.54939419854,-9.29670991483252));
#69506=CARTESIAN_POINT('Ctrl Pts',(41.5867483123806,-12.5563297590485,-9.21517000013748));
#69507=CARTESIAN_POINT('Ctrl Pts',(41.574793301892,-12.5632653195569,-9.1339033638181));
#69508=CARTESIAN_POINT('Ctrl Pts',(41.5586876183147,-12.5702008800654,-9.05335854337322));
#69509=CARTESIAN_POINT('Ctrl Pts',(41.5426074010974,-12.5771254740426,-8.97294108066456));
#69510=CARTESIAN_POINT('Ctrl Pts',(41.5223896476239,-12.5840500680199,-8.89324358831412));
#69511=CARTESIAN_POINT('Ctrl Pts',(41.4981164888731,-12.5909746619971,-8.81470882874016));
#69512=CARTESIAN_POINT('Ctrl Pts',(41.473881501497,-12.5978883665275,-8.73629757100507));
#69513=CARTESIAN_POINT('Ctrl Pts',(41.4456039330987,-12.6048020710579,-8.65904581993135));
#69514=CARTESIAN_POINT('Ctrl Pts',(41.4134164805572,-12.6117157755884,-8.58338413989683));
#69515=CARTESIAN_POINT('Ctrl Pts',(41.3812588456174,-12.6186230754464,-8.50779255083449));
#69516=CARTESIAN_POINT('Ctrl Pts',(41.3451986982026,-12.6255303753044,-8.43378850320112));
#69517=CARTESIAN_POINT('Ctrl Pts',(41.3054176952937,-12.6324376751625,-8.36178494131817));
#69518=CARTESIAN_POINT('Ctrl Pts',(41.2656638151787,-12.639340265605,-8.28983047165588));
#69519=CARTESIAN_POINT('Ctrl Pts',(41.2221943354176,-12.6462428560476,-8.21987415539018));
#69520=CARTESIAN_POINT('Ctrl Pts',(41.1752374670053,-12.6531454464902,-8.15230560817845));
#69521=CARTESIAN_POINT('Ctrl Pts',(41.1283011405467,-12.6600450172958,-8.08476661979401));
#69522=CARTESIAN_POINT('Ctrl Pts',(41.0778807094616,-12.6669445881015,-8.01961367923981));
#69523=CARTESIAN_POINT('Ctrl Pts',(41.0242478569796,-12.6738441589071,-7.95720769847997));
#69524=CARTESIAN_POINT('Ctrl Pts',(40.9706098995415,-12.6807443864373,-7.8947957777081));
#69525=CARTESIAN_POINT('Ctrl Pts',(40.913759186687,-12.6876446139674,-7.83513167569318));
#69526=CARTESIAN_POINT('Ctrl Pts',(40.854007437666,-12.6945448414975,-7.77854291763422));
#69527=CARTESIAN_POINT('Ctrl Pts',(40.7942556066665,-12.7014450784946,-7.72195408193639));
#69528=CARTESIAN_POINT('Ctrl Pts',(40.7316030523931,-12.7083453154917,-7.66844089369298));
#69529=CARTESIAN_POINT('Ctrl Pts',(40.6663969572748,-12.7152455524888,-7.61829265274002));
#69530=CARTESIAN_POINT('Ctrl Pts',(40.6011444758808,-12.7221506981727,-7.56810873735922));
#69531=CARTESIAN_POINT('Ctrl Pts',(40.5333351737933,-12.7290558438566,-7.52129481301359));
#69532=CARTESIAN_POINT('Ctrl Pts',(40.4633474192269,-12.7359609895405,-7.47809837981088));
#69533=CARTESIAN_POINT('Ctrl Pts',(40.4159161815491,-12.7406406596937,-7.44882382595842));
#69534=CARTESIAN_POINT('Ctrl Pts',(40.3674850379813,-12.7453203298468,-7.42120985453868));
#69535=CARTESIAN_POINT('Ctrl Pts',(40.3181783974771,-12.75,-7.39532161681263));
#69536=CARTESIAN_POINT('Ctrl Pts',(36.7946210320027,-11.8956214580413,-9.52722816428394));
#69537=CARTESIAN_POINT('Ctrl Pts',(36.7945104667753,-11.8862658381917,-9.40786924872099));
#69538=CARTESIAN_POINT('Ctrl Pts',(36.8032839374915,-11.8768622465317,-9.28867798243652));
#69539=CARTESIAN_POINT('Ctrl Pts',(36.8251651662405,-11.8648356185918,-9.14177147686941));
#69540=CARTESIAN_POINT('Ctrl Pts',(36.8299891894927,-11.8624587560463,-9.11298882687568));
#69541=CARTESIAN_POINT('Ctrl Pts',(36.8390759405276,-11.8583923497813,-9.06423179043359));
#69542=CARTESIAN_POINT('Ctrl Pts',(36.8430716794022,-11.8567109743571,-9.0442104438046));
#69543=CARTESIAN_POINT('Ctrl Pts',(36.8515198883864,-11.8533529365506,-9.00451870099323));
#69544=CARTESIAN_POINT('Ctrl Pts',(36.8559658566946,-11.8516766043042,-8.98484863204398));
#69545=CARTESIAN_POINT('Ctrl Pts',(36.8651906959268,-11.8483656869082,-8.94629648569365));
#69546=CARTESIAN_POINT('Ctrl Pts',(36.8699526424761,-11.8467317600666,-8.92741192479448));
#69547=CARTESIAN_POINT('Ctrl Pts',(36.8809762653888,-11.8431062195011,-8.88583171043609));
#69548=CARTESIAN_POINT('Ctrl Pts',(36.8873428245448,-11.8411113778412,-8.86316626886844));
#69549=CARTESIAN_POINT('Ctrl Pts',(36.9107217626599,-11.8341110687762,-8.78439540198754));
#69550=CARTESIAN_POINT('Ctrl Pts',(36.9294502714909,-11.829051585831,-8.7288262188455));
#69551=CARTESIAN_POINT('Ctrl Pts',(36.9527678797602,-11.8232961015687,-8.66718071860874));
#69552=CARTESIAN_POINT('Ctrl Pts',(36.9553784964742,-11.8226584942794,-8.66037268072647));
#69553=CARTESIAN_POINT('Ctrl Pts',(36.9580196917093,-11.8220201063326,-8.65357746090844));
#69554=CARTESIAN_POINT('Origin',(39.2,-12.75,-9.525));
#69555=CARTESIAN_POINT('',(41.1084785589541,-12.75,-11.9808583515571));
#69556=CARTESIAN_POINT('',(36.08977,-12.75,-9.525));
#69557=CARTESIAN_POINT('Origin',(39.2,-12.75,-9.525));
#69558=CARTESIAN_POINT('Ctrl Pts',(41.1084785589541,-12.75,-11.9808583515571));
#69559=CARTESIAN_POINT('Ctrl Pts',(41.1177983966318,-12.75,-11.9717669582536));
#69560=CARTESIAN_POINT('Ctrl Pts',(41.1270543353679,-12.75,-11.9626123445009));
#69561=CARTESIAN_POINT('Ctrl Pts',(41.1362455536515,-12.75,-11.9533945855071));
#69562=CARTESIAN_POINT('Ctrl Pts',(41.2078661956446,-12.75,-11.8815671305931));
#69563=CARTESIAN_POINT('Ctrl Pts',(41.2755608385581,-12.75,-11.8059075492844));
#69564=CARTESIAN_POINT('Ctrl Pts',(41.3392177633947,-12.75,-11.7268202136986));
#69565=CARTESIAN_POINT('Ctrl Pts',(41.3943876820438,-12.75,-11.6582771308897));
#69566=CARTESIAN_POINT('Ctrl Pts',(41.4465241253691,-12.75,-11.5871584953386));
#69567=CARTESIAN_POINT('Ctrl Pts',(41.4955251476878,-12.75,-11.5137175255415));
#69568=CARTESIAN_POINT('Ctrl Pts',(41.5101767234174,-12.75,-11.4917582708215));
#69569=CARTESIAN_POINT('Ctrl Pts',(41.5245486734672,-12.75,-11.4695899646366));
#69570=CARTESIAN_POINT('Ctrl Pts',(41.5386355217927,-12.75,-11.4472228736974));
#69571=CARTESIAN_POINT('Ctrl Pts',(41.5519504183468,-12.75,-11.4260814874063));
#69572=CARTESIAN_POINT('Ctrl Pts',(41.5650061724716,-12.75,-11.404769422587));
#69573=CARTESIAN_POINT('Ctrl Pts',(41.5777948568304,-12.75,-11.3833028614934));
#69574=CARTESIAN_POINT('Ctrl Pts',(41.6294048341385,-12.75,-11.2966724701383));
#69575=CARTESIAN_POINT('Ctrl Pts',(41.6766999371217,-12.75,-11.2074785188293));
#69576=CARTESIAN_POINT('Ctrl Pts',(41.7195470841769,-12.75,-11.1161137346045));
#69577=CARTESIAN_POINT('Ctrl Pts',(41.7620308413559,-12.75,-11.025523821985));
#69578=CARTESIAN_POINT('Ctrl Pts',(41.8001418510265,-12.75,-10.9327987519571));
#69579=CARTESIAN_POINT('Ctrl Pts',(41.8336996271297,-12.75,-10.8383186854066));
#69580=CARTESIAN_POINT('Ctrl Pts',(41.8380607202485,-12.75,-10.8260402684213));
#69581=CARTESIAN_POINT('Ctrl Pts',(41.8423448419313,-12.75,-10.813732219562));
#69582=CARTESIAN_POINT('Ctrl Pts',(41.8465515312897,-12.75,-10.8013953832721));
#69583=CARTESIAN_POINT('Ctrl Pts',(41.8519573108627,-12.75,-10.7855420097684));
#69584=CARTESIAN_POINT('Ctrl Pts',(41.857235428307,-12.75,-10.7696402235551));
#69585=CARTESIAN_POINT('Ctrl Pts',(41.8623800097954,-12.75,-10.7537076086219));
#69586=CARTESIAN_POINT('Ctrl Pts',(41.8924329745631,-12.75,-10.6606344759834));
#69587=CARTESIAN_POINT('Ctrl Pts',(41.9179769286029,-12.75,-10.5663842906978));
#69588=CARTESIAN_POINT('Ctrl Pts',(41.9388991726743,-12.75,-10.4713165340972));
#69589=CARTESIAN_POINT('Ctrl Pts',(41.9595829880513,-12.7499999999999,-10.3773321642029));
#69590=CARTESIAN_POINT('Ctrl Pts',(41.9757498406875,-12.75,-10.282547834876));
#69591=CARTESIAN_POINT('Ctrl Pts',(41.9872405753498,-12.75,-10.1873132752954));
#69592=CARTESIAN_POINT('Ctrl Pts',(41.998401906114,-12.75,-10.0948087966098));
#69593=CARTESIAN_POINT('Ctrl Pts',(42.0051512351925,-12.75,-10.0018788103257));
#69594=CARTESIAN_POINT('Ctrl Pts',(42.0072961959229,-12.75,-9.90885796114165));
#69595=CARTESIAN_POINT('Ctrl Pts',(42.0085525980484,-12.75,-9.85437137265856));
#69596=CARTESIAN_POINT('Ctrl Pts',(42.0082283810938,-12.75,-9.79985393080354));
#69597=CARTESIAN_POINT('Ctrl Pts',(42.0062774111146,-12.75,-9.74537669181848));
#69598=CARTESIAN_POINT('Ctrl Pts',(42.0056087070014,-12.75,-9.7267043625824));
#69599=CARTESIAN_POINT('Ctrl Pts',(42.0047488424704,-12.7499999999999,-9.70803678557931));
#69600=CARTESIAN_POINT('Ctrl Pts',(42.0036958084692,-12.75,-9.68937691893248));
#69601=CARTESIAN_POINT('Ctrl Pts',(42.0029149036918,-12.75,-9.67553920904492));
#69602=CARTESIAN_POINT('Ctrl Pts',(42.0020282962605,-12.75,-9.66171521265807));
#69603=CARTESIAN_POINT('Ctrl Pts',(42.0010356525435,-12.75,-9.64790697816443));
#69604=CARTESIAN_POINT('Ctrl Pts',(41.9945063923453,-12.75,-9.55708128276281));
#69605=CARTESIAN_POINT('Ctrl Pts',(41.9833925950157,-12.7499999999999,-9.46692217583271));
#69606=CARTESIAN_POINT('Ctrl Pts',(41.9675554099829,-12.75,-9.37773775964327));
#69607=CARTESIAN_POINT('Ctrl Pts',(41.9607505630484,-12.75,-9.33941742052689));
#69608=CARTESIAN_POINT('Ctrl Pts',(41.9530730683015,-12.75,-9.30127722046684));
#69609=CARTESIAN_POINT('Ctrl Pts',(41.9445091332559,-12.75,-9.26334269611395));
#69610=CARTESIAN_POINT('Ctrl Pts',(41.9237890194308,-12.75,-9.1715615629886));
#69611=CARTESIAN_POINT('Ctrl Pts',(41.897882700181,-12.7499999999999,-9.08098197605832));
#69612=CARTESIAN_POINT('Ctrl Pts',(41.8670374313203,-12.75,-8.99192525440121));
#69613=CARTESIAN_POINT('Ctrl Pts',(41.8361921624596,-12.75,-8.90286853274409));
#69614=CARTESIAN_POINT('Ctrl Pts',(41.8004070957505,-12.75,-8.81533391622066));
#69615=CARTESIAN_POINT('Ctrl Pts',(41.7598933162349,-12.75,-8.72968369143849));
#69616=CARTESIAN_POINT('Ctrl Pts',(41.7520217401559,-12.75,-8.71304238399647));
#69617=CARTESIAN_POINT('Ctrl Pts',(41.7439715676172,-12.75,-8.69647235644754));
#69618=CARTESIAN_POINT('Ctrl Pts',(41.7357442304968,-12.75,-8.67997648296463));
#69619=CARTESIAN_POINT('Ctrl Pts',(41.729514813746,-12.75,-8.66748645501395));
#69620=CARTESIAN_POINT('Ctrl Pts',(41.7231878371419,-12.7499999999999,-8.65504700546118));
#69621=CARTESIAN_POINT('Ctrl Pts',(41.7167654750851,-12.75,-8.64266142135632));
#69622=CARTESIAN_POINT('Ctrl Pts',(41.6752249123853,-12.75,-8.56255006535911));
#69623=CARTESIAN_POINT('Ctrl Pts',(41.6296810084744,-12.75,-8.48465727580426));
#69624=CARTESIAN_POINT('Ctrl Pts',(41.580378827968,-12.75,-8.40925152491517));
#69625=CARTESIAN_POINT('Ctrl Pts',(41.5314354814769,-12.7499999999999,-8.33439459657495));
#69626=CARTESIAN_POINT('Ctrl Pts',(41.4787875447868,-12.75,-8.26198804712867));
#69627=CARTESIAN_POINT('Ctrl Pts',(41.4226420462153,-12.75,-8.19233310842445));
#69628=CARTESIAN_POINT('Ctrl Pts',(41.3670515962938,-12.75,-8.12336677131231));
#69629=CARTESIAN_POINT('Ctrl Pts',(41.3080316361269,-12.75,-8.05709740682041));
#69630=CARTESIAN_POINT('Ctrl Pts',(41.2457626467438,-12.75,-7.99386341792389));
#69631=CARTESIAN_POINT('Ctrl Pts',(41.2267639300686,-12.75,-7.97457027295411));
#69632=CARTESIAN_POINT('Ctrl Pts',(41.2074626579876,-12.75,-7.95556004729628));
#69633=CARTESIAN_POINT('Ctrl Pts',(41.1878637361297,-12.75,-7.93684332516778));
#69634=CARTESIAN_POINT('Ctrl Pts',(41.1712853455817,-12.75,-7.9210111721812));
#69635=CARTESIAN_POINT('Ctrl Pts',(41.1544939793358,-12.75,-7.90538903367538));
#69636=CARTESIAN_POINT('Ctrl Pts',(41.1374925744962,-12.75,-7.88998358950291));
#69637=CARTESIAN_POINT('Ctrl Pts',(41.1276172064111,-12.75,-7.88103524475422));
#69638=CARTESIAN_POINT('Ctrl Pts',(41.1176718130391,-12.75,-7.87216086334629));
#69639=CARTESIAN_POINT('Ctrl Pts',(41.1076664155748,-12.75,-7.86336977076331));
#69640=CARTESIAN_POINT('Ctrl Pts',(41.0432046529541,-12.75,-7.80673140879069));
#69641=CARTESIAN_POINT('Ctrl Pts',(40.9761510753172,-12.75,-7.75345252931226));
#69642=CARTESIAN_POINT('Ctrl Pts',(40.9066975736398,-12.75,-7.70379730514819));
#69643=CARTESIAN_POINT('Ctrl Pts',(40.8383344183618,-12.75,-7.65492161540032));
#69644=CARTESIAN_POINT('Ctrl Pts',(40.7676453780882,-12.75,-7.60955634955628));
#69645=CARTESIAN_POINT('Ctrl Pts',(40.694798190339,-12.75,-7.56800068927081));
#69646=CARTESIAN_POINT('Ctrl Pts',(40.6241249698281,-12.75,-7.52768516806028));
#69647=CARTESIAN_POINT('Ctrl Pts',(40.5514198830853,-12.75,-7.49095512491116));
#69648=CARTESIAN_POINT('Ctrl Pts',(40.4768312911088,-12.75,-7.45813193578272));
#69649=CARTESIAN_POINT('Ctrl Pts',(40.4248450302792,-12.75,-7.4352550476947));
#69650=CARTESIAN_POINT('Ctrl Pts',(40.3719437125909,-12.75,-7.41427698771476));
#69651=CARTESIAN_POINT('Ctrl Pts',(40.3181783974771,-12.75,-7.39532161681262));
#69652=CARTESIAN_POINT('',(37.423659425391,-12.7512312321065,-7.90004131257367));
#69653=CARTESIAN_POINT('Ctrl Pts',(37.4444040758239,-12.75,-7.88069592367579));
#69654=CARTESIAN_POINT('Ctrl Pts',(37.4379608436199,-12.7504104107022,-7.88757525479146));
#69655=CARTESIAN_POINT('Ctrl Pts',(37.4315580470395,-12.7508208214043,-7.89449245820598));
#69656=CARTESIAN_POINT('Ctrl Pts',(37.4251961284841,-12.7512312321065,-7.90144705597498));
#69657=CARTESIAN_POINT('Ctrl Pts',(37.4219896448371,-12.75,-7.89867535481033));
#69658=CARTESIAN_POINT('Ctrl Pts',(37.4041800318868,-12.75,-7.91315252990336));
#69659=CARTESIAN_POINT('Ctrl Pts',(37.3866079915316,-12.75,-7.92789833873796));
#69660=CARTESIAN_POINT('Ctrl Pts',(37.3692807783977,-12.75,-7.94290979008526));
#69661=CARTESIAN_POINT('Ctrl Pts',(37.3073978200408,-12.75,-7.99652216337458));
#69662=CARTESIAN_POINT('Ctrl Pts',(37.2486361525171,-12.75,-8.05351884266802));
#69663=CARTESIAN_POINT('Ctrl Pts',(37.1930196554172,-12.75,-8.11352008911787));
#69664=CARTESIAN_POINT('Ctrl Pts',(37.1575846699701,-12.75,-8.15174873359617));
#69665=CARTESIAN_POINT('Ctrl Pts',(37.1234267578552,-12.75,-8.19119811603227));
#69666=CARTESIAN_POINT('Ctrl Pts',(37.0905565908903,-12.75,-8.23178001255319));
#69667=CARTESIAN_POINT('Ctrl Pts',(37.0738455802734,-12.75,-8.25241162371415));
#69668=CARTESIAN_POINT('Ctrl Pts',(37.0574674682131,-12.75,-8.27333606608347));
#69669=CARTESIAN_POINT('Ctrl Pts',(37.0414240687244,-12.75,-8.29454242346543));
#69670=CARTESIAN_POINT('Ctrl Pts',(37.0265574148782,-12.75,-8.314193344379));
#69671=CARTESIAN_POINT('Ctrl Pts',(37.0119749045712,-12.75,-8.33409122869043));
#69672=CARTESIAN_POINT('Ctrl Pts',(36.9976972145749,-12.75,-8.35420012550333));
#69673=CARTESIAN_POINT('Ctrl Pts',(36.9478117565662,-12.75,-8.42445949714009));
#69674=CARTESIAN_POINT('Ctrl Pts',(36.9016057374712,-12.75,-8.49734007805571));
#69675=CARTESIAN_POINT('Ctrl Pts',(36.8591144753857,-12.75,-8.57244354508648));
#69676=CARTESIAN_POINT('Ctrl Pts',(36.8225527531614,-12.75,-8.63706652790425));
#69677=CARTESIAN_POINT('Ctrl Pts',(36.7887415597637,-12.75,-8.70333641037004));
#69678=CARTESIAN_POINT('Ctrl Pts',(36.7577206548755,-12.75,-8.77102495961378));
#69679=CARTESIAN_POINT('Ctrl Pts',(36.748069517199,-12.75,-8.79208403284934));
#69680=CARTESIAN_POINT('Ctrl Pts',(36.7386885924217,-12.75,-8.81328057411961));
#69681=CARTESIAN_POINT('Ctrl Pts',(36.7295794455984,-12.75,-8.83460808988947));
#69682=CARTESIAN_POINT('Ctrl Pts',(36.7220483554448,-12.75,-8.85224085475003));
#69683=CARTESIAN_POINT('Ctrl Pts',(36.7147022785046,-12.75,-8.86996535756085));
#69684=CARTESIAN_POINT('Ctrl Pts',(36.7075507171553,-12.75,-8.88775585391959));
#69685=CARTESIAN_POINT('Ctrl Pts',(36.6740987028843,-12.75,-8.97097235854196));
#69686=CARTESIAN_POINT('Ctrl Pts',(36.644855758403,-12.75,-9.05573011267507));
#69687=CARTESIAN_POINT('Ctrl Pts',(36.6198544411057,-12.75,-9.14161810772437));
#69688=CARTESIAN_POINT('Ctrl Pts',(36.5943080999463,-12.75,-9.22937844438731));
#69689=CARTESIAN_POINT('Ctrl Pts',(36.5731897292325,-12.75,-9.31831956866093));
#69690=CARTESIAN_POINT('Ctrl Pts',(36.5565704314595,-12.75,-9.4080440570504));
#69691=CARTESIAN_POINT('Ctrl Pts',(36.5401253552976,-12.75,-9.49682795546161));
#69692=CARTESIAN_POINT('Ctrl Pts',(36.5280851134617,-12.75,-9.58637983259742));
#69693=CARTESIAN_POINT('Ctrl Pts',(36.5205611019666,-12.75,-9.67634142246066));
#69694=CARTESIAN_POINT('Ctrl Pts',(36.5158634381635,-12.75,-9.73250950575603));
#69695=CARTESIAN_POINT('Ctrl Pts',(36.5129271579462,-12.75,-9.78883778500213));
#69696=CARTESIAN_POINT('Ctrl Pts',(36.5117889942815,-12.75,-9.84524193459141));
#69697=CARTESIAN_POINT('Ctrl Pts',(36.5115191770569,-12.75,-9.85861330776889));
#69698=CARTESIAN_POINT('Ctrl Pts',(36.5113505718752,-12.75,-9.87198485331457));
#69699=CARTESIAN_POINT('Ctrl Pts',(36.5112834643196,-12.75,-9.88534723852641));
#69700=CARTESIAN_POINT('Ctrl Pts',(36.5108085549604,-12.75,-9.97991068595048));
#69701=CARTESIAN_POINT('Ctrl Pts',(36.5154106260062,-12.75,-10.074134730613));
#69702=CARTESIAN_POINT('Ctrl Pts',(36.5251526597289,-12.75,-10.1676019130765));
#69703=CARTESIAN_POINT('Ctrl Pts',(36.529414730784,-12.75,-10.2084931462955));
#69704=CARTESIAN_POINT('Ctrl Pts',(36.5346611529582,-12.75,-10.2492398965073));
#69705=CARTESIAN_POINT('Ctrl Pts',(36.5408999787326,-12.75,-10.2898086508596));
#69706=CARTESIAN_POINT('Ctrl Pts',(36.5547918865281,-12.75,-10.3801425398342));
#69707=CARTESIAN_POINT('Ctrl Pts',(36.5736003964838,-12.75,-10.4695937030868));
#69708=CARTESIAN_POINT('Ctrl Pts',(36.5970362254893,-12.75,-10.5579348213263));
#69709=CARTESIAN_POINT('Ctrl Pts',(36.6204720544947,-12.75,-10.6462759395658));
#69710=CARTESIAN_POINT('Ctrl Pts',(36.6485355160504,-12.75,-10.7335076916399));
#69711=CARTESIAN_POINT('Ctrl Pts',(36.6809898727762,-12.75,-10.8194022563315));
#69712=CARTESIAN_POINT('Ctrl Pts',(36.6899298075195,-12.75,-10.8430629256718));
#69713=CARTESIAN_POINT('Ctrl Pts',(36.699203211383,-12.75,-10.8666220939594));
#69714=CARTESIAN_POINT('Ctrl Pts',(36.7088057864774,-12.75,-10.8900748849566));
#69715=CARTESIAN_POINT('Ctrl Pts',(36.7144182844112,-12.75,-10.903782535219));
#69716=CARTESIAN_POINT('Ctrl Pts',(36.7201400708447,-12.75,-10.9174460470224));
#69717=CARTESIAN_POINT('Ctrl Pts',(36.725968063952,-12.75,-10.9310603421251));
#69718=CARTESIAN_POINT('Ctrl Pts',(36.7632844244424,-12.75,-11.0182320210414));
#69719=CARTESIAN_POINT('Ctrl Pts',(36.8049729222028,-12.75,-11.1034402117559));
#69720=CARTESIAN_POINT('Ctrl Pts',(36.8507031457334,-12.75,-11.186447825772));
#69721=CARTESIAN_POINT('Ctrl Pts',(36.897242032023,-12.75,-11.2709232910466));
#69722=CARTESIAN_POINT('Ctrl Pts',(36.9479670801348,-12.75,-11.3531203940572));
#69723=CARTESIAN_POINT('Ctrl Pts',(37.0025849524151,-12.75,-11.4327882625403));
#69724=CARTESIAN_POINT('Ctrl Pts',(37.0579909527395,-12.75,-11.5136057269111));
#69725=CARTESIAN_POINT('Ctrl Pts',(37.1174032465806,-12.75,-11.5918212706129));
#69726=CARTESIAN_POINT('Ctrl Pts',(37.1805674478662,-12.75,-11.667160078329));
#69727=CARTESIAN_POINT('Ctrl Pts',(37.2181975830789,-12.75,-11.71204324733));
#69728=CARTESIAN_POINT('Ctrl Pts',(37.2571603082924,-12.75,-11.755905103373));
#69729=CARTESIAN_POINT('Ctrl Pts',(37.2974096407888,-12.75,-11.7986835008897));
#69730=CARTESIAN_POINT('Ctrl Pts',(37.3076886400212,-12.75,-11.8096083805825));
#69731=CARTESIAN_POINT('Ctrl Pts',(37.3180531561345,-12.75,-11.8204642006903));
#69732=CARTESIAN_POINT('Ctrl Pts',(37.3284973899992,-12.75,-11.831244642987));
#69733=CARTESIAN_POINT('Ctrl Pts',(37.399176916415,-12.75,-11.9041994011775));
#69734=CARTESIAN_POINT('Ctrl Pts',(37.4733055554982,-12.75,-11.9735015455736));
#69735=CARTESIAN_POINT('Ctrl Pts',(37.5505563567699,-12.75,-12.0388871187713));
#69736=CARTESIAN_POINT('Ctrl Pts',(37.6282447166439,-12.75,-12.1046430443735));
#69737=CARTESIAN_POINT('Ctrl Pts',(37.7090911707722,-12.75,-12.1664387621244));
#69738=CARTESIAN_POINT('Ctrl Pts',(37.7928131421831,-12.75,-12.2239879195989));
#69739=CARTESIAN_POINT('Ctrl Pts',(37.8752801154996,-12.75,-12.2806744112551));
#69740=CARTESIAN_POINT('Ctrl Pts',(37.9605376456359,-12.75,-12.333241449453));
#69741=CARTESIAN_POINT('Ctrl Pts',(38.0483558365738,-12.75,-12.3813862473665));
#69742=CARTESIAN_POINT('Ctrl Pts',(38.1254402939299,-12.75,-12.4236464622724));
#69743=CARTESIAN_POINT('Ctrl Pts',(38.2044985066156,-12.75,-12.462499334437));
#69744=CARTESIAN_POINT('Ctrl Pts',(38.2853957334118,-12.75,-12.4977141955524));
#69745=CARTESIAN_POINT('Origin',(39.2,-12.75,-9.525));
#69746=CARTESIAN_POINT('Ctrl Pts',(38.1090601293427,6.10939317307034,-7.3859991646148));
#69747=CARTESIAN_POINT('Ctrl Pts',(37.4014250801391,6.04252457258368,-7.74690939722429));
#69748=CARTESIAN_POINT('Ctrl Pts',(36.3842966957365,5.90878737161036,-9.2198489270829));
#69749=CARTESIAN_POINT('Ctrl Pts',(37.4068122137656,5.70818157015037,-11.7207065033657));
#69750=CARTESIAN_POINT('Ctrl Pts',(40.0578012994608,5.5075757686904,-12.224479871604));
#69751=CARTESIAN_POINT('Ctrl Pts',(41.9297097031944,5.3069699672304,-10.2834563771707));
#69752=CARTESIAN_POINT('Ctrl Pts',(41.3270630938264,5.10636416577043,-7.6531776804645));
#69753=CARTESIAN_POINT('Ctrl Pts',(38.7953478358015,4.90575836431044,-6.72097002802451));
#69754=CARTESIAN_POINT('Ctrl Pts',(36.6307235789104,4.70515256285046,-8.33095570597218));
#69755=CARTESIAN_POINT('Ctrl Pts',(36.795736350814,4.50454676139048,-11.0238574475027));
#69756=CARTESIAN_POINT('Ctrl Pts',(39.1408882915444,4.3039409599305,-12.3575487902617));
#69757=CARTESIAN_POINT('Ctrl Pts',(41.5396181212764,4.10333515847052,-11.12284467284));
#69758=CARTESIAN_POINT('Ctrl Pts',(41.8168821219755,3.90272935701054,-8.43924848869504));
#69759=CARTESIAN_POINT('Ctrl Pts',(39.7212505068437,3.70212355555055,-6.74018448494738));
#69760=CARTESIAN_POINT('Ctrl Pts',(37.1529716231046,3.50151775409057,-7.5662788780741));
#69761=CARTESIAN_POINT('Ctrl Pts',(36.4408591567146,3.30091195263059,-10.1684711251898));
#69762=CARTESIAN_POINT('Ctrl Pts',(38.2306320743938,3.10030615117061,-12.1871862476963));
#69763=CARTESIAN_POINT('Ctrl Pts',(40.8993907810134,2.89970034971063,-11.7919324649524));
#69764=CARTESIAN_POINT('Ctrl Pts',(42.0272063778795,2.69909454825064,-9.34110954729177));
#69765=CARTESIAN_POINT('Ctrl Pts',(40.5914180124664,2.49848874679066,-7.05703178483132));
#69766=CARTESIAN_POINT('Ctrl Pts',(37.8939444502983,2.29788294533068,-7.01081417098301));
#69767=CARTESIAN_POINT('Ctrl Pts',(36.3807526568316,2.0972771438707,-9.24436527970491));
#69768=CARTESIAN_POINT('Ctrl Pts',(37.4239477837834,1.89667134241071,-11.7323853104763));
#69769=CARTESIAN_POINT('Ctrl Pts',(40.0775999080307,1.69606554095074,-12.218831810624));
#69770=CARTESIAN_POINT('Ctrl Pts',(41.9354776177662,1.49545973949075,-10.262613459155));
#69771=CARTESIAN_POINT('Ctrl Pts',(41.3129276391037,1.29485393803077,-7.63755511343507));
#69772=CARTESIAN_POINT('Ctrl Pts',(38.7744547594159,1.09424813657079,-6.72396043203959));
#69773=CARTESIAN_POINT('Ctrl Pts',(36.6218502152785,0.893642335110802,-8.35024253613623));
#69774=CARTESIAN_POINT('Ctrl Pts',(36.8070144268541,0.693036533650818,-11.0417502950991));
#69775=CARTESIAN_POINT('Ctrl Pts',(39.1620474870164,0.492430732190839,-12.3579262289002));
#69776=CARTESIAN_POINT('Ctrl Pts',(41.5514944511869,0.291824930730855,-11.1053117595593));
#69777=CARTESIAN_POINT('Ctrl Pts',(41.8086951473945,0.0912191292708744,
-8.41973033186413));
#69778=CARTESIAN_POINT('Ctrl Pts',(39.7004297080759,-0.109386672189109,
-6.7363656534607));
#69779=CARTESIAN_POINT('Ctrl Pts',(37.1383935286702,-0.30999247364909,-7.5816291736382));
#69780=CARTESIAN_POINT('Ctrl Pts',(36.4457441565455,-0.510598275109072,
-10.1890678882323));
#69781=CARTESIAN_POINT('Ctrl Pts',(38.2505498560931,-0.711204076569056,
-12.1943549474788));
#69782=CARTESIAN_POINT('Ctrl Pts',(40.9162810513022,-0.911809878029036,
-11.7791718577627));
#69783=CARTESIAN_POINT('Ctrl Pts',(42.0257534747706,-1.11241567948902,-9.31999094846492));
#69784=CARTESIAN_POINT('Ctrl Pts',(40.572939477521,-1.313021480949,-7.04670449654313));
#69785=CARTESIAN_POINT('Ctrl Pts',(37.8751958672925,-1.51362728240898,-7.02064271292006));
#69786=CARTESIAN_POINT('Ctrl Pts',(36.378734559167,-1.71423308386896,-9.26543743769494));
#69787=CARTESIAN_POINT('Ctrl Pts',(37.4404900922592,-1.91483888532894,-11.7455936809672));
#69788=CARTESIAN_POINT('Ctrl Pts',(40.0977026898037,-2.11544468678892,-12.2121995259207));
#69789=CARTESIAN_POINT('Ctrl Pts',(41.9409124267084,-2.3160504882489,-10.242154432814));
#69790=CARTESIAN_POINT('Ctrl Pts',(41.2987663977842,-2.51665628970889,-7.6218208127131));
#69791=CARTESIAN_POINT('Ctrl Pts',(38.7535383451392,-2.71726209116887,-6.72721812820788));
#69792=CARTESIAN_POINT('Ctrl Pts',(36.6131448422295,-2.91786789262886,-8.36953827233206));
#69793=CARTESIAN_POINT('Ctrl Pts',(36.8184137979523,-3.11847369408883,-11.0595874278143));
#69794=CARTESIAN_POINT('Ctrl Pts',(39.1832150836397,-3.31907949554882,-12.3581307202409));
#69795=CARTESIAN_POINT('Ctrl Pts',(41.5632362969134,-3.5196852970088,-11.0876981846604));
#69796=CARTESIAN_POINT('Ctrl Pts',(41.8003641804634,-3.72029109846878,-8.4002700144691));
#69797=CARTESIAN_POINT('Ctrl Pts',(39.6795801343239,-3.92089689992876,-6.73270447370779));
#69798=CARTESIAN_POINT('Ctrl Pts',(37.1239309533467,-4.12150270138875,-7.59708695089287));
#69799=CARTESIAN_POINT('Ctrl Pts',(36.4507826961788,-4.32210850284872,-10.2096280944859));
#69800=CARTESIAN_POINT('Ctrl Pts',(38.2705207534323,-4.52271430430871,-12.2013743649926));
#69801=CARTESIAN_POINT('Ctrl Pts',(40.9330754516574,-4.72332010576869,-11.7662855441136));
#69802=CARTESIAN_POINT('Ctrl Pts',(42.0241428508277,-4.92392590722868,-9.29888372568953));
#69803=CARTESIAN_POINT('Ctrl Pts',(40.5543842821803,-5.12453170868865,-7.03651559627705));
#69804=CARTESIAN_POINT('Ctrl Pts',(37.8565212501926,-5.32513751014864,-7.03061104472332));
#69805=CARTESIAN_POINT('Ctrl Pts',(36.3768739570832,-5.52574331160863,-9.28652409515082));
#69806=CARTESIAN_POINT('Ctrl Pts',(37.457130628819,-5.72634911306861,-11.7586780802944));
#69807=CARTESIAN_POINT('Ctrl Pts',(40.1177553555661,-5.92695491452858,-12.2054172284784));
#69808=CARTESIAN_POINT('Ctrl Pts',(41.9461942224683,-6.12756071598857,-10.2216553695093));
#69809=CARTESIAN_POINT('Ctrl Pts',(41.2844879908318,-6.32816651744855,-7.60619275917001));
#69810=CARTESIAN_POINT('Ctrl Pts',(38.7326468550866,-6.52877231890854,-6.73063201253607));
#69811=CARTESIAN_POINT('Ctrl Pts',(36.6045838824426,-6.72937812036851,-8.38889851330806));
#69812=CARTESIAN_POINT('Ctrl Pts',(36.8299461230947,-6.9299839218285,-11.077338890813));
#69813=CARTESIAN_POINT('Ctrl Pts',(39.2043836172943,-7.13058972328848,-12.3581770498033));
#69814=CARTESIAN_POINT('Ctrl Pts',(41.5748462129954,-7.33119552474845,-11.0699973707383));
#69815=CARTESIAN_POINT('Ctrl Pts',(41.7918880461159,-7.53180132620844,-8.38087248623012));
#69816=CARTESIAN_POINT('Ctrl Pts',(39.6587037874852,-7.73240712766843,-6.72919917583345));
#69817=CARTESIAN_POINT('Ctrl Pts',(37.1095842765501,-7.93301292912841,-7.6126523561178));
#69818=CARTESIAN_POINT('Ctrl Pts',(36.4559747126355,-8.13361873058839,-10.2301500795792));
#69819=CARTESIAN_POINT('Ctrl Pts',(38.2905435407064,-8.33422453204837,-12.2082443741029));
#69820=CARTESIAN_POINT('Ctrl Pts',(40.9497730997094,-8.53483033350836,-11.7532741041371));
#69821=CARTESIAN_POINT('Ctrl Pts',(42.0223745705614,-8.73543613496833,-9.27778913525879));
#69822=CARTESIAN_POINT('Ctrl Pts',(40.5357534698105,-8.93604193642833,-7.02646559967134));
#69823=CARTESIAN_POINT('Ctrl Pts',(37.8379216484013,-9.13664773788829,-7.04071866315316));
#69824=CARTESIAN_POINT('Ctrl Pts',(36.3751709299713,-9.33725353934829,-9.30762399663186));
#69825=CARTESIAN_POINT('Ctrl Pts',(37.4738685180293,-9.53785934080825,-11.7716379179115));
#69826=CARTESIAN_POINT('Ctrl Pts',(40.1377566782039,-9.73846514226827,-12.1984850299003));
#69827=CARTESIAN_POINT('Ctrl Pts',(41.9513229223509,-9.93907094372821,-10.2011179327488));
#69828=CARTESIAN_POINT('Ctrl Pts',(41.2700927993691,-10.1396767451883,-7.59067081103199));
#69829=CARTESIAN_POINT('Ctrl Pts',(38.7117822700447,-10.3402825466482,-6.73420387847481));
#69830=CARTESIAN_POINT('Ctrl Pts',(36.596166219581,-10.5408883481082,-8.40831829576861));
#69831=CARTESIAN_POINT('Ctrl Pts',(36.8416138787086,-10.7414941495682,-11.095011291306));
#69832=CARTESIAN_POINT('Ctrl Pts',(39.225545799572,-10.9420999510282,-12.3580503446663));
#69833=CARTESIAN_POINT('Ctrl Pts',(41.5863355026778,-11.1427057524881,-11.0522394086686));
#69834=CARTESIAN_POINT('Ctrl Pts',(41.7832438274538,-11.3433115539481,-8.36148187294322));
#69835=CARTESIAN_POINT('Ctrl Pts',(39.6378476098593,-11.5439173554081,-6.72596142787065));
#69836=CARTESIAN_POINT('Ctrl Pts',(37.095264708429,-11.7445231568681,-7.62810634102885));
#69837=CARTESIAN_POINT('Ctrl Pts',(36.4614952627569,-11.9451289583281,-10.2510598762372));
#69838=CARTESIAN_POINT('Ctrl Pts',(38.3102738378103,-12.1457347597881,-12.2141266245507));
#69839=CARTESIAN_POINT('Ctrl Pts',(40.9670458444618,-12.346340561248,-11.741799149493));
#69840=CARTESIAN_POINT('Ctrl Pts',(42.0192942539946,-12.5469793475859,-9.25282332578296));
#69841=CARTESIAN_POINT('Ctrl Pts',(41.0190233754115,-12.6807495334372,-7.76761236952371));
#69842=CARTESIAN_POINT('Ctrl Pts',(40.3151665400905,-12.7476511188018,-7.39852924898774));
#69843=CARTESIAN_POINT('Ctrl Pts',(38.0010709531129,5.97216720292314,-7.17426527865005));
#69844=CARTESIAN_POINT('Ctrl Pts',(37.2233890314003,5.90529860243647,-7.57090103542516));
#69845=CARTESIAN_POINT('Ctrl Pts',(36.1055778694168,5.77156140146314,-9.1896428507662));
#69846=CARTESIAN_POINT('Ctrl Pts',(37.2293094227601,5.57095560000318,-11.9380535294654));
#69847=CARTESIAN_POINT('Ctrl Pts',(40.1427127214274,5.37034979854318,-12.4916940558357));
#69848=CARTESIAN_POINT('Ctrl Pts',(42.1999162563905,5.16974399708322,-10.3585339149708));
#69849=CARTESIAN_POINT('Ctrl Pts',(41.5376152951616,4.96913819562322,-7.46789107047617));
#69850=CARTESIAN_POINT('Ctrl Pts',(38.7552924165738,4.76853239416325,-6.44340671317846));
#69851=CARTESIAN_POINT('Ctrl Pts',(36.3763978807827,4.56792659270326,-8.21276050276974));
#69852=CARTESIAN_POINT('Ctrl Pts',(36.5577448190182,4.36732079124328,-11.1722252772934));
#69853=CARTESIAN_POINT('Ctrl Pts',(39.1350369839945,4.1667149897833,-12.6379351055101));
#69854=CARTESIAN_POINT('Ctrl Pts',(41.7712105677572,3.96610918832332,-11.281010979347));
#69855=CARTESIAN_POINT('Ctrl Pts',(42.0759201791991,3.76550338686334,-8.33177289407273));
#69856=CARTESIAN_POINT('Ctrl Pts',(39.7728476794813,3.56489758540335,-6.46452315703079));
#69857=CARTESIAN_POINT('Ctrl Pts',(36.9503418411289,3.36429178394337,-7.37239039154066));
#69858=CARTESIAN_POINT('Ctrl Pts',(36.1677392948574,3.16368598248338,-10.232166585046));
#69859=CARTESIAN_POINT('Ctrl Pts',(38.1346769749741,2.96308018102341,-12.450708837338));
#69860=CARTESIAN_POINT('Ctrl Pts',(41.067608861102,2.76247437956342,-12.0163299556329));
#69861=CARTESIAN_POINT('Ctrl Pts',(42.3070638622291,2.56186857810344,-9.32290673058429));
#69862=CARTESIAN_POINT('Ctrl Pts',(40.7291507042482,2.36126277664346,-6.81273431098717));
#69863=CARTESIAN_POINT('Ctrl Pts',(37.7646615569729,2.16065697518348,-6.76194174101064));
#69864=CARTESIAN_POINT('Ctrl Pts',(36.1016830157217,1.9600511737235,-9.21658601057989));
#69865=CARTESIAN_POINT('Ctrl Pts',(37.2481411963361,1.75944537226351,-11.9508883899875));
#69866=CARTESIAN_POINT('Ctrl Pts',(40.1644711405125,1.55883957080353,-12.485486908632));
#69867=CARTESIAN_POINT('Ctrl Pts',(42.2062551211676,1.35823376934355,-10.3356278130829));
#69868=CARTESIAN_POINT('Ctrl Pts',(41.5220806101492,1.15762796788356,-7.45072206794696));
#69869=CARTESIAN_POINT('Ctrl Pts',(38.7323311912751,0.957022166423585,-6.44669312916898));
#69870=CARTESIAN_POINT('Ctrl Pts',(36.3666461669734,0.7564163649636,-8.2339564838939));
#69871=CARTESIAN_POINT('Ctrl Pts',(36.5701392811891,0.555810563503619,-11.1918892892999));
#69872=CARTESIAN_POINT('Ctrl Pts',(39.1582906707855,0.355204762043637,-12.6383499057747));
#69873=CARTESIAN_POINT('Ctrl Pts',(41.784262503325,0.154598960583655,-11.2617425305772));
#69874=CARTESIAN_POINT('Ctrl Pts',(42.0669227982292,-0.0460068408763262,
-8.31032268788294));
#69875=CARTESIAN_POINT('Ctrl Pts',(39.7499658863656,-0.246612642336309,
-6.46032630978219));
#69876=CARTESIAN_POINT('Ctrl Pts',(36.9343207007013,-0.44721844379629,-7.38926017119132));
#69877=CARTESIAN_POINT('Ctrl Pts',(36.1731078475604,-0.647824245256273,
-10.2548021657482));
#69878=CARTESIAN_POINT('Ctrl Pts',(38.1565663638131,-0.848430046716256,
-12.4585871472511));
#69879=CARTESIAN_POINT('Ctrl Pts',(41.0861710533949,-1.04903584817623,-12.0023062105786));
#69880=CARTESIAN_POINT('Ctrl Pts',(42.3054671401856,-1.24964164963622,-9.29969765899009));
#69881=CARTESIAN_POINT('Ctrl Pts',(40.7088430292921,-1.4502474510962,-6.80138475246677));
#69882=CARTESIAN_POINT('Ctrl Pts',(37.7440571026318,-1.65085325255618,-6.77274318363257));
#69883=CARTESIAN_POINT('Ctrl Pts',(36.0994651520476,-1.85145905401616,-9.23974404428493));
#69884=CARTESIAN_POINT('Ctrl Pts',(37.2663209830207,-2.05206485547615,-11.9654042212166));
#69885=CARTESIAN_POINT('Ctrl Pts',(40.1865638420804,-2.25267065693612,-12.4781981120706));
#69886=CARTESIAN_POINT('Ctrl Pts',(42.2122279070932,-2.45327645839611,-10.3131436032643));
#69887=CARTESIAN_POINT('Ctrl Pts',(41.5065175859948,-2.65388225985609,-7.43343027151031));
#69888=CARTESIAN_POINT('Ctrl Pts',(38.7093443179308,-2.85448806131607,-6.45027329583733));
#69889=CARTESIAN_POINT('Ctrl Pts',(36.3570790726787,-3.05509386277605,-8.25516225263374));
#69890=CARTESIAN_POINT('Ctrl Pts',(36.5826670450864,-3.25569966423604,-11.2114920713602));
#69891=CARTESIAN_POINT('Ctrl Pts',(39.181553590335,-3.45630546569602,-12.6385746391581));
#69892=CARTESIAN_POINT('Ctrl Pts',(41.7971666424844,-3.656911267156,-11.2423854357145));
#69893=CARTESIAN_POINT('Ctrl Pts',(42.0577671714977,-3.85751706861598,-8.28893604649776));
#69894=CARTESIAN_POINT('Ctrl Pts',(39.727052469908,-4.05812287007596,-6.45630271978454));
#69895=CARTESIAN_POINT('Ctrl Pts',(36.9184265143081,-4.25872867153595,-7.40624807185329));
#69896=CARTESIAN_POINT('Ctrl Pts',(36.1786451385538,-4.45933447299593,-10.277397571004));
#69897=CARTESIAN_POINT('Ctrl Pts',(38.1785141260651,-4.65994027445591,-12.4663013978492));
#69898=CARTESIAN_POINT('Ctrl Pts',(41.1046278858496,-4.8605460759159,-11.9881443157238));
#69899=CARTESIAN_POINT('Ctrl Pts',(42.3036970849511,-5.06115187737588,-9.27650108953178));
#69900=CARTESIAN_POINT('Ctrl Pts',(40.6884511055362,-5.26175767883585,-6.79018728062308));
#69901=CARTESIAN_POINT('Ctrl Pts',(37.7235339358813,-5.46236348029585,-6.78369825354006));
#69902=CARTESIAN_POINT('Ctrl Pts',(36.0974203740146,-5.66296928175581,-9.26291801271858));
#69903=CARTESIAN_POINT('Ctrl Pts',(37.2846087211206,-5.86357508321581,-11.9797838097131));
#69904=CARTESIAN_POINT('Ctrl Pts',(40.2086014667897,-6.06418088467578,-12.4707444534163));
#69905=CARTESIAN_POINT('Ctrl Pts',(42.2180325334768,-6.26478668613577,-10.2906153933317));
#69906=CARTESIAN_POINT('Ctrl Pts',(41.4908257982998,-6.46539248759575,-7.41625523937237));
#69907=CARTESIAN_POINT('Ctrl Pts',(38.6863848359917,-6.66599828905573,-6.45402511130751));
#69908=CARTESIAN_POINT('Ctrl Pts',(36.347670686723,-6.86660409051572,-8.27643891130687));
#69909=CARTESIAN_POINT('Ctrl Pts',(36.5953409237878,-7.06720989197569,-11.2310007034914));
#69910=CARTESIAN_POINT('Ctrl Pts',(39.2048175396701,-7.26781569343568,-12.6386255547581));
#69911=CARTESIAN_POINT('Ctrl Pts',(41.8099257926419,-7.46842149489566,-11.2229324662745));
#69912=CARTESIAN_POINT('Ctrl Pts',(42.0484520076212,-7.66902729635564,-8.26761840959673));
#69913=CARTESIAN_POINT('Ctrl Pts',(39.7041096301685,-7.86963309781562,-6.45245044198942));
#69914=CARTESIAN_POINT('Ctrl Pts',(36.9026596989223,-8.07023889927561,-7.42335425428616));
#69915=CARTESIAN_POINT('Ctrl Pts',(36.1843510986247,-8.27084470073558,-10.2999509716909));
#69916=CARTESIAN_POINT('Ctrl Pts',(38.2005189146958,-8.47145050219558,-12.4738514505113));
#69917=CARTESIAN_POINT('Ctrl Pts',(41.1229783887533,-8.67205630365554,-11.9738449086261));
#69918=CARTESIAN_POINT('Ctrl Pts',(42.3017537674215,-8.87266210511554,-9.25331840285964));
#69919=CARTESIAN_POINT('Ctrl Pts',(40.6679760796267,-9.07326790657551,-6.77914246213601));
#69920=CARTESIAN_POINT('Ctrl Pts',(37.7030932100009,-9.2738737080355,-6.79480639767921));
#69921=CARTESIAN_POINT('Ctrl Pts',(36.0955487688721,-9.47447950949547,-9.28610653616747));
#69922=CARTESIAN_POINT('Ctrl Pts',(37.3030034485457,-9.67508531095546,-11.9940265064739));
#69923=CARTESIAN_POINT('Ctrl Pts',(40.2305826660579,-9.87569111241545,-12.4631260553198));
#69924=CARTESIAN_POINT('Ctrl Pts',(42.2236689094381,-10.0762969138754,-10.2680450114592));
#69925=CARTESIAN_POINT('Ctrl Pts',(41.4750056659128,-10.2769027153354,-7.39919681572548));
#69926=CARTESIAN_POINT('Ctrl Pts',(38.6634549223176,-10.4775085167954,-6.457950546559));
#69927=CARTESIAN_POINT('Ctrl Pts',(36.338419782266,-10.6781143182554,-8.29778100531444));
#69928=CARTESIAN_POINT('Ctrl Pts',(36.6081636388556,-10.8787201197154,-11.2504224469341));
#69929=CARTESIAN_POINT('Ctrl Pts',(39.2280745089226,-11.0793259211754,-12.6384863074236));
#69930=CARTESIAN_POINT('Ctrl Pts',(41.8225523759202,-11.2799317226353,-11.203416691747));
#69931=CARTESIAN_POINT('Ctrl Pts',(42.0389521212201,-11.4805375240954,-8.24630837214011));
#69932=CARTESIAN_POINT('Ctrl Pts',(39.6811889561377,-11.6811433255553,-6.44889219814528));
#69933=CARTESIAN_POINT('Ctrl Pts',(36.886922675626,-11.8817491270153,-7.44033798721073));
#69934=CARTESIAN_POINT('Ctrl Pts',(36.1904181130162,-12.0823549284753,-10.3229305723563));
#69935=CARTESIAN_POINT('Ctrl Pts',(38.2222022603483,-12.2829607299353,-12.4803159689624));
#69936=CARTESIAN_POINT('Ctrl Pts',(41.1419609156184,-12.4835665313952,-11.9612340793728));
#69937=CARTESIAN_POINT('Ctrl Pts',(42.2983685386799,-12.6842053177331,-9.22588129567827));
#69938=CARTESIAN_POINT('Ctrl Pts',(41.1990835612539,-12.8179755035844,-7.59365333875032));
#69939=CARTESIAN_POINT('Ctrl Pts',(40.4255538485596,-12.884877088949,-7.18803568205975));
#69940=CARTESIAN_POINT('Ctrl Pts',(37.8930817768831,5.83494123277593,-6.9625313926853));
#69941=CARTESIAN_POINT('Ctrl Pts',(37.0453529826617,5.76807263228927,-7.39489267362603));
#69942=CARTESIAN_POINT('Ctrl Pts',(35.826859043097,5.63433543131595,-9.15943677444951));
#69943=CARTESIAN_POINT('Ctrl Pts',(37.0518066317547,5.43372962985597,-12.155400555565));
#69944=CARTESIAN_POINT('Ctrl Pts',(40.227624143394,5.23312382839599,-12.7589082400674));
#69945=CARTESIAN_POINT('Ctrl Pts',(42.4701228095865,5.03251802693601,-10.433611452771));
#69946=CARTESIAN_POINT('Ctrl Pts',(41.7481674964967,4.83191222547602,-7.28260446048784));
#69947=CARTESIAN_POINT('Ctrl Pts',(38.7152369973462,4.63130642401604,-6.16584339833242));
#69948=CARTESIAN_POINT('Ctrl Pts',(36.1220721826552,4.43070062255606,-8.09456529956729));
#69949=CARTESIAN_POINT('Ctrl Pts',(36.3197532872223,4.23009482109608,-11.3205931070843));
#69950=CARTESIAN_POINT('Ctrl Pts',(39.1291856764446,4.02948901963609,-12.9183214207584));
#69951=CARTESIAN_POINT('Ctrl Pts',(42.0028030142381,3.82888321817611,-11.4391772858541));
#69952=CARTESIAN_POINT('Ctrl Pts',(42.3349582364225,3.62827741671613,-8.22429729945043));
#69953=CARTESIAN_POINT('Ctrl Pts',(39.8244448521188,3.42767161525615,-6.18886182911421));
#69954=CARTESIAN_POINT('Ctrl Pts',(36.7477120591531,3.22706581379617,-7.17850190500721));
#69955=CARTESIAN_POINT('Ctrl Pts',(35.8946194330003,3.02646001233618,-10.2958620449021));
#69956=CARTESIAN_POINT('Ctrl Pts',(38.0387218755544,2.8258542108762,-12.7142314269797));
#69957=CARTESIAN_POINT('Ctrl Pts',(41.2358269411907,2.62524840941622,-12.2407274463135));
#69958=CARTESIAN_POINT('Ctrl Pts',(42.5869213465787,2.42464260795624,-9.30470391387682));
#69959=CARTESIAN_POINT('Ctrl Pts',(40.8668833960298,2.22403680649626,-6.56843683714305));
#69960=CARTESIAN_POINT('Ctrl Pts',(37.6353786636475,2.02343100503627,-6.51306931103826));
#69961=CARTESIAN_POINT('Ctrl Pts',(35.8226133746117,1.82282520357629,-9.18880674145491));
#69962=CARTESIAN_POINT('Ctrl Pts',(37.0723346088889,1.62221940211631,-12.1693914694987));
#69963=CARTESIAN_POINT('Ctrl Pts',(40.2513423729944,1.42161360065633,-12.75214200664));
#69964=CARTESIAN_POINT('Ctrl Pts',(42.4770326245692,1.22100779919635,-10.4086421670107));
#69965=CARTESIAN_POINT('Ctrl Pts',(41.7312335811948,1.02040199773636,-7.26388902245885));
#69966=CARTESIAN_POINT('Ctrl Pts',(38.6902076231343,0.819796196276384,-6.16942582629837));
#69967=CARTESIAN_POINT('Ctrl Pts',(36.1114421186684,0.6191903948164,-8.11767043165157));
#69968=CARTESIAN_POINT('Ctrl Pts',(36.3332641355238,0.418584593356419,-11.3420282835007));
#69969=CARTESIAN_POINT('Ctrl Pts',(39.1545338545546,0.217978791896437,-12.9187735826493));
#69970=CARTESIAN_POINT('Ctrl Pts',(42.0170305554631,0.0173729904364543,
-11.4181733015951));
#69971=CARTESIAN_POINT('Ctrl Pts',(42.325150449064,-0.183232811023527,-8.20091504390175));
#69972=CARTESIAN_POINT('Ctrl Pts',(39.7995020646551,-0.383838612483509,
-6.1842869661037));
#69973=CARTESIAN_POINT('Ctrl Pts',(36.7302478727325,-0.584444413943491,
-7.19689116874442));
#69974=CARTESIAN_POINT('Ctrl Pts',(35.9004715385751,-0.785050215403473,
-10.320536443264));
#69975=CARTESIAN_POINT('Ctrl Pts',(38.0625828715332,-0.985656016863457,
-12.7228193470235));
#69976=CARTESIAN_POINT('Ctrl Pts',(41.2560610554877,-1.18626181832344,-12.2254405633946));
#69977=CARTESIAN_POINT('Ctrl Pts',(42.5851808056007,-1.38686761978342,-9.27940436951522));
#69978=CARTESIAN_POINT('Ctrl Pts',(40.844746581063,-1.5874734212434,-6.55606500839041));
#69979=CARTESIAN_POINT('Ctrl Pts',(37.6129183379714,-1.78807922270338,-6.52484365434506));
#69980=CARTESIAN_POINT('Ctrl Pts',(35.8201957449284,-1.98868502416336,-9.21405065087494));
#69981=CARTESIAN_POINT('Ctrl Pts',(37.0921518737822,-2.18929082562335,-12.185214761466));
#69982=CARTESIAN_POINT('Ctrl Pts',(40.2754249943571,-2.38989662708333,-12.7441966982204));
#69983=CARTESIAN_POINT('Ctrl Pts',(42.4835433874781,-2.59050242854331,-10.3841327737147));
#69984=CARTESIAN_POINT('Ctrl Pts',(41.7142687742056,-2.79110823000329,-7.24503973030753));
#69985=CARTESIAN_POINT('Ctrl Pts',(38.6651502907223,-2.99171403146327,-6.17332846346677));
#69986=CARTESIAN_POINT('Ctrl Pts',(36.1010133031279,-3.19231983292326,-8.14078623293544));
#69987=CARTESIAN_POINT('Ctrl Pts',(36.3469202922205,-3.39292563438324,-11.3633967149062));
#69988=CARTESIAN_POINT('Ctrl Pts',(39.1798920970303,-3.59353143584322,-12.9190185580753));
#69989=CARTESIAN_POINT('Ctrl Pts',(42.0310969880554,-3.79413723730321,-11.3970726867687));
#69990=CARTESIAN_POINT('Ctrl Pts',(42.3151701625321,-3.99474303876318,-8.17760207852641));
#69991=CARTESIAN_POINT('Ctrl Pts',(39.774524805492,-4.19534884022317,-6.17990096586128));
#69992=CARTESIAN_POINT('Ctrl Pts',(36.7129220752694,-4.39595464168314,-7.21540919281373));
#69993=CARTESIAN_POINT('Ctrl Pts',(35.9065075809288,-4.59656044314314,-10.3451670475223));
#69994=CARTESIAN_POINT('Ctrl Pts',(38.0865074986978,-4.79716624460311,-12.7312284307056));
#69995=CARTESIAN_POINT('Ctrl Pts',(41.2761803200418,-4.9977720460631,-12.210003087334));
#69996=CARTESIAN_POINT('Ctrl Pts',(42.5832513190743,-5.19837784752307,-9.25411845337402));
#69997=CARTESIAN_POINT('Ctrl Pts',(40.822517928892,-5.39898364898306,-6.54385896496911));
#69998=CARTESIAN_POINT('Ctrl Pts',(37.5905466215699,-5.59958945044304,-6.53678546235682));
#69999=CARTESIAN_POINT('Ctrl Pts',(35.817966790946,-5.80019525190303,-9.23931193028633));
#70000=CARTESIAN_POINT('Ctrl Pts',(37.1120868134222,-6.000801053363,-12.2008895391316));
#70001=CARTESIAN_POINT('Ctrl Pts',(40.2994475780133,-6.20140685482298,-12.7360716783542));
#70002=CARTESIAN_POINT('Ctrl Pts',(42.4898708444855,-6.40201265628298,-10.3595754171542));
#70003=CARTESIAN_POINT('Ctrl Pts',(41.6971636057678,-6.60261845774295,-7.22631771957472));
#70004=CARTESIAN_POINT('Ctrl Pts',(38.640122816897,-6.80322425920293,-6.17741821007895));
#70005=CARTESIAN_POINT('Ctrl Pts',(36.0907574910032,-7.00383006066292,-8.16397930930566));
#70006=CARTESIAN_POINT('Ctrl Pts',(36.3607357244811,-7.20443586212289,-11.3846625161698));
#70007=CARTESIAN_POINT('Ctrl Pts',(39.2052514620458,-7.40504166358289,-12.919074059713));
#70008=CARTESIAN_POINT('Ctrl Pts',(42.0450053722886,-7.60564746504285,-11.3758675618108));
#70009=CARTESIAN_POINT('Ctrl Pts',(42.3050159691265,-7.80625326650285,-8.15436433296333));
#70010=CARTESIAN_POINT('Ctrl Pts',(39.7495154728519,-8.00685906796282,-6.17570170814539));
#70011=CARTESIAN_POINT('Ctrl Pts',(36.6957351212943,-8.20746486942281,-7.2340561524545));
#70012=CARTESIAN_POINT('Ctrl Pts',(35.9127274846142,-8.40807067088279,-10.3697518638027));
#70013=CARTESIAN_POINT('Ctrl Pts',(38.1104942886851,-8.60867647234277,-12.7394585269196));
#70014=CARTESIAN_POINT('Ctrl Pts',(41.2961836777971,-8.80928227380275,-12.1944157131151));
#70015=CARTESIAN_POINT('Ctrl Pts',(42.5811329642816,-9.00988807526274,-9.22884767046046));
#70016=CARTESIAN_POINT('Ctrl Pts',(40.800198689443,-9.21049387672271,-6.5318193246007));
#70017=CARTESIAN_POINT('Ctrl Pts',(37.5682647716004,-9.4110996781827,-6.54889413220524));
#70018=CARTESIAN_POINT('Ctrl Pts',(35.815926607773,-9.61170547964268,-9.26458907570309));
#70019=CARTESIAN_POINT('Ctrl Pts',(37.132138379062,-9.81231128110266,-12.2164150950363));
#70020=CARTESIAN_POINT('Ctrl Pts',(40.323408653912,-10.0129170825627,-12.7277670807392));
#70021=CARTESIAN_POINT('Ctrl Pts',(42.4960148965253,-10.2135228840226,-10.3349720901695));
#70022=CARTESIAN_POINT('Ctrl Pts',(41.6799185324564,-10.4141286854826,-7.20772282041896));
#70023=CARTESIAN_POINT('Ctrl Pts',(38.6151275745906,-10.6147344869426,-6.1816972146432));
#70024=CARTESIAN_POINT('Ctrl Pts',(36.080673344951,-10.8153402884026,-8.18724371486027));
#70025=CARTESIAN_POINT('Ctrl Pts',(36.3747133990027,-11.0159460898626,-11.4058336025622));
#70026=CARTESIAN_POINT('Ctrl Pts',(39.2306032182732,-11.2165518913226,-12.9189222701809));
#70027=CARTESIAN_POINT('Ctrl Pts',(42.0587692491625,-11.4171576927825,-11.3545939748253));
#70028=CARTESIAN_POINT('Ctrl Pts',(42.2946604149865,-11.6177634942425,-8.131134871337));
#70029=CARTESIAN_POINT('Ctrl Pts',(39.7245303024159,-11.8183692957025,-6.1718229684199));
#70030=CARTESIAN_POINT('Ctrl Pts',(36.678580642823,-12.0189750971625,-7.2525696333926));
#70031=CARTESIAN_POINT('Ctrl Pts',(35.9193409632754,-12.2195808986225,-10.3948012684755));
#70032=CARTESIAN_POINT('Ctrl Pts',(38.1341306828862,-12.4201867000825,-12.7465053133741));
#70033=CARTESIAN_POINT('Ctrl Pts',(41.3168759867752,-12.6207925015424,-12.1806690092526));
#70034=CARTESIAN_POINT('Ctrl Pts',(42.5774428233651,-12.8214312878803,-9.19893926557358));
#70035=CARTESIAN_POINT('Ctrl Pts',(41.3791437470964,-12.9552014737316,-7.41969430797695));
#70036=CARTESIAN_POINT('Ctrl Pts',(40.5359411570286,-13.0221030590962,-6.97754211513178));
#70037=CARTESIAN_POINT('Ctrl Pts',(37.7850926006533,5.69771526262873,-6.75079750672056));
#70038=CARTESIAN_POINT('Ctrl Pts',(36.8673169339229,5.63084666214207,-7.2188843118269));
#70039=CARTESIAN_POINT('Ctrl Pts',(35.5481402167774,5.49710946116874,-9.12923069813283));
#70040=CARTESIAN_POINT('Ctrl Pts',(36.8743038407491,5.29650365970877,-12.3727475816646));
#70041=CARTESIAN_POINT('Ctrl Pts',(40.3125355653607,5.09589785824878,-13.0261224242991));
#70042=CARTESIAN_POINT('Ctrl Pts',(42.7403293627825,4.89529205678881,-10.5086889905711));
#70043=CARTESIAN_POINT('Ctrl Pts',(41.9587196978319,4.69468625532882,-7.09731785049951));
#70044=CARTESIAN_POINT('Ctrl Pts',(38.6751815781184,4.49408045386884,-5.88828008348638));
#70045=CARTESIAN_POINT('Ctrl Pts',(35.8677464845275,4.29347465240886,-7.97637009636483));
#70046=CARTESIAN_POINT('Ctrl Pts',(36.0817617554265,4.09286885094887,-11.468960936875));
#70047=CARTESIAN_POINT('Ctrl Pts',(39.1233343688946,3.89226304948889,-13.1987077360068));
#70048=CARTESIAN_POINT('Ctrl Pts',(42.2343954607189,3.69165724802891,-11.5973435923613));
#70049=CARTESIAN_POINT('Ctrl Pts',(42.5939962936459,3.49105144656893,-8.11682170482813));
#70050=CARTESIAN_POINT('Ctrl Pts',(39.8760420247564,3.29044564510895,-5.91320050119763));
#70051=CARTESIAN_POINT('Ctrl Pts',(36.5450822771773,3.08983984364896,-6.98461341847376));
#70052=CARTESIAN_POINT('Ctrl Pts',(35.6214995711431,2.88923404218898,-10.3595575047582));
#70053=CARTESIAN_POINT('Ctrl Pts',(37.9427667761347,2.688628240729,-12.9777540166216));
#70054=CARTESIAN_POINT('Ctrl Pts',(41.4040450212794,2.48802243926902,-12.465124936994));
#70055=CARTESIAN_POINT('Ctrl Pts',(42.8667788309283,2.28741663780904,-9.28650109716934));
#70056=CARTESIAN_POINT('Ctrl Pts',(41.0046160878115,2.08681083634905,-6.32413936329892));
#70057=CARTESIAN_POINT('Ctrl Pts',(37.506095770322,1.88620503488907,-6.26419688106589));
#70058=CARTESIAN_POINT('Ctrl Pts',(35.5435437335017,1.68559923342909,-9.1610274723299));
#70059=CARTESIAN_POINT('Ctrl Pts',(36.8965280214417,1.48499343196911,-12.3878945490098));
#70060=CARTESIAN_POINT('Ctrl Pts',(40.3382136054761,1.28438763050913,-13.018797104648));
#70061=CARTESIAN_POINT('Ctrl Pts',(42.7478101279706,1.08378182904914,-10.4816565209386));
#70062=CARTESIAN_POINT('Ctrl Pts',(41.9403865522403,0.883176027589163,-7.07705597697076));
#70063=CARTESIAN_POINT('Ctrl Pts',(38.6480840549934,0.682570226129183,-5.89215852342776));
#70064=CARTESIAN_POINT('Ctrl Pts',(35.8562380703633,0.481964424669198,-8.00138437940923));
#70065=CARTESIAN_POINT('Ctrl Pts',(36.0963889898587,0.281358623209219,-11.4921672777015));
#70066=CARTESIAN_POINT('Ctrl Pts',(39.1507770383239,0.0807528217492357,
-13.1991972595238));
#70067=CARTESIAN_POINT('Ctrl Pts',(42.249798607601,-0.119852979710745,-11.5746040726131));
#70068=CARTESIAN_POINT('Ctrl Pts',(42.5833780998989,-0.320458781170727,
-8.09150739992054));
#70069=CARTESIAN_POINT('Ctrl Pts',(39.8490382429447,-0.52106458263071,-5.90824762242522));
#70070=CARTESIAN_POINT('Ctrl Pts',(36.5261750447638,-0.721670384090691,
-7.00452216629751));
#70071=CARTESIAN_POINT('Ctrl Pts',(35.6278352295899,-0.922276185550674,
-10.3862707207798));
#70072=CARTESIAN_POINT('Ctrl Pts',(37.9685993792531,-1.12288198701066,-12.9870515467959));
#70073=CARTESIAN_POINT('Ctrl Pts',(41.4259510575803,-1.32348778847064,-12.4485749162106));
#70074=CARTESIAN_POINT('Ctrl Pts',(42.8648944710158,-1.52409358993062,-9.25911108004038));
#70075=CARTESIAN_POINT('Ctrl Pts',(40.980650132834,-1.72469939139061,-6.31074526431405));
#70076=CARTESIAN_POINT('Ctrl Pts',(37.4817795733109,-1.92530519285059,-6.27694412505756));
#70077=CARTESIAN_POINT('Ctrl Pts',(35.5409263378092,-2.12591099431056,-9.18835725746494));
#70078=CARTESIAN_POINT('Ctrl Pts',(36.9179827645437,-2.32651679577055,-12.4050253017153));
#70079=CARTESIAN_POINT('Ctrl Pts',(40.3642861466337,-2.52712259723053,-13.0101952843703));
#70080=CARTESIAN_POINT('Ctrl Pts',(42.7548588678629,-2.72772839869051,-10.455121944165));
#70081=CARTESIAN_POINT('Ctrl Pts',(41.9220199624163,-2.92833420015049,-7.05664918910476));
#70082=CARTESIAN_POINT('Ctrl Pts',(38.6209562635138,-3.12894000161048,-5.8963836310962));
#70083=CARTESIAN_POINT('Ctrl Pts',(35.8449475335771,-3.32954580307046,-8.02641021323713));
#70084=CARTESIAN_POINT('Ctrl Pts',(36.1111735393545,-3.53015160453044,-11.5153013584522));
#70085=CARTESIAN_POINT('Ctrl Pts',(39.1782306037257,-3.73075740599042,-13.1994624769925));
#70086=CARTESIAN_POINT('Ctrl Pts',(42.2650273336264,-3.93136320745041,-11.5517599378228));
#70087=CARTESIAN_POINT('Ctrl Pts',(42.5725731535664,-4.13196900891039,-8.06626811055506));
#70088=CARTESIAN_POINT('Ctrl Pts',(39.8219971410761,-4.33257481037037,-5.90349921193802));
#70089=CARTESIAN_POINT('Ctrl Pts',(36.5074176362308,-4.53318061183036,-7.02457031377417));
#70090=CARTESIAN_POINT('Ctrl Pts',(35.6343700233036,-4.73378641329033,-10.4129365240405));
#70091=CARTESIAN_POINT('Ctrl Pts',(37.9945008713306,-4.93439221475032,-12.9961554635622));
#70092=CARTESIAN_POINT('Ctrl Pts',(41.447732754234,-5.1349980162103,-12.4318618589442));
#70093=CARTESIAN_POINT('Ctrl Pts',(42.8628055531978,-5.33560381767028,-9.23173581721625));
#70094=CARTESIAN_POINT('Ctrl Pts',(40.9565847522478,-5.53620961913025,-6.29753064931515));
#70095=CARTESIAN_POINT('Ctrl Pts',(37.4575593072585,-5.73681542059025,-6.28987267117355));
#70096=CARTESIAN_POINT('Ctrl Pts',(35.5385132078774,-5.93742122205023,-9.2157058478541));
#70097=CARTESIAN_POINT('Ctrl Pts',(36.9395649057238,-6.13802702351021,-12.4219952685503));
#70098=CARTESIAN_POINT('Ctrl Pts',(40.3902936892369,-6.33863282497019,-13.0013989032921));
#70099=CARTESIAN_POINT('Ctrl Pts',(42.7617091554941,-6.53923862643018,-10.4285354409766));
#70100=CARTESIAN_POINT('Ctrl Pts',(41.9035014132359,-6.73984442789015,-7.03638019977707));
#70101=CARTESIAN_POINT('Ctrl Pts',(38.5938607978023,-6.94045022935015,-5.90081130885039));
#70102=CARTESIAN_POINT('Ctrl Pts',(35.8338442952836,-7.14105603081011,-8.05151970730447));
#70103=CARTESIAN_POINT('Ctrl Pts',(36.1261305251742,-7.3416618322701,-11.5383243288482));
#70104=CARTESIAN_POINT('Ctrl Pts',(39.2056853844216,-7.54226763373008,-13.1995225646678));
#70105=CARTESIAN_POINT('Ctrl Pts',(42.2800849519353,-7.74287343519007,-11.5288026573471));
#70106=CARTESIAN_POINT('Ctrl Pts',(42.561579930632,-7.94347923665003,-8.04111025632993));
#70107=CARTESIAN_POINT('Ctrl Pts',(39.7949213155352,-8.14408503811002,-5.89895297430136));
#70108=CARTESIAN_POINT('Ctrl Pts',(36.4888105436665,-8.34469083957002,-7.04475805062286));
#70109=CARTESIAN_POINT('Ctrl Pts',(35.6411038706034,-8.54529664102998,-10.4395527559144));
#70110=CARTESIAN_POINT('Ctrl Pts',(38.0204696626744,-8.74590244248998,-13.005065603328));
#70111=CARTESIAN_POINT('Ctrl Pts',(41.469388966841,-8.94650824394996,-12.4149865176041));
#70112=CARTESIAN_POINT('Ctrl Pts',(42.8605121611417,-9.14711404540993,-9.20437693806131));
#70113=CARTESIAN_POINT('Ctrl Pts',(40.9324212992594,-9.34771984686993,-6.28449618706538));
#70114=CARTESIAN_POINT('Ctrl Pts',(37.4334363331999,-9.5483256483299,-6.30298186673129));
#70115=CARTESIAN_POINT('Ctrl Pts',(35.5363044466738,-9.74893144978988,-9.2430716152387));
#70116=CARTESIAN_POINT('Ctrl Pts',(36.9612733095783,-9.94953725124986,-12.4388036835987));
#70117=CARTESIAN_POINT('Ctrl Pts',(40.4162346417662,-10.1501430527099,-12.9924081061586));
#70118=CARTESIAN_POINT('Ctrl Pts',(42.7683608836124,-10.3507488541699,-10.4018991688799));
#70119=CARTESIAN_POINT('Ctrl Pts',(41.8848313990001,-10.5513546556298,-7.01624882511245));
#70120=CARTESIAN_POINT('Ctrl Pts',(38.5668002268634,-10.7519604570898,-5.9054438827274));
#70121=CARTESIAN_POINT('Ctrl Pts',(35.822926907636,-10.9525662585498,-8.0767064244061));
#70122=CARTESIAN_POINT('Ctrl Pts',(36.1412631591497,-11.1531720600098,-11.5612447581902));
#70123=CARTESIAN_POINT('Ctrl Pts',(39.2331319276237,-11.3537778614698,-13.1993582329382));
#70124=CARTESIAN_POINT('Ctrl Pts',(42.294986122405,-11.5543836629298,-11.5057712579037));
#70125=CARTESIAN_POINT('Ctrl Pts',(42.5503687087529,-11.7549894643897,-8.0159613705339));
#70126=CARTESIAN_POINT('Ctrl Pts',(39.7678716486943,-11.9555952658497,-5.89475373869452));
#70127=CARTESIAN_POINT('Ctrl Pts',(36.47023861002,-12.1562010673097,-7.06480127957447));
#70128=CARTESIAN_POINT('Ctrl Pts',(35.6482638135347,-12.3568068687697,-10.4666719645947));
#70129=CARTESIAN_POINT('Ctrl Pts',(38.0460591054243,-12.5574126702297,-13.0126946577859));
#70130=CARTESIAN_POINT('Ctrl Pts',(41.4917910579318,-12.7580184716896,-12.4001039391323));
#70131=CARTESIAN_POINT('Ctrl Pts',(42.8565171080503,-12.9586572580275,-9.17199723546892));
#70132=CARTESIAN_POINT('Ctrl Pts',(41.5592039329389,-13.0924274438788,-7.24573527720356));
#70133=CARTESIAN_POINT('Ctrl Pts',(40.6463284654976,-13.1593290292434,-6.76704854820381));
#70134=CARTESIAN_POINT('Ctrl Pts',(41.0695067500478,-12.75,-12.0106538705994));
#70135=CARTESIAN_POINT('Ctrl Pts',(41.0824973530166,-12.75,-12.0007220309186));
#70136=CARTESIAN_POINT('Ctrl Pts',(41.0954879559853,-12.75,-11.9907901912378));
#70137=CARTESIAN_POINT('Ctrl Pts',(41.1084785589541,-12.75,-11.9808583515571));
#70138=CARTESIAN_POINT('Ctrl Pts',(37.728785320723,5.69999999999999,-11.4333446637284));
#70139=CARTESIAN_POINT('Ctrl Pts',(37.7087477093809,5.7,-11.4221525029985));
#70140=CARTESIAN_POINT('Ctrl Pts',(37.6888978346145,5.69999999999999,-11.4106547954623));
#70141=CARTESIAN_POINT('Ctrl Pts',(37.6692433579699,5.69999999999999,-11.398853237781));
#70142=CARTESIAN_POINT('Ctrl Pts',(37.5993515170885,5.69999999999998,-11.3568865852708));
#70143=CARTESIAN_POINT('Ctrl Pts',(37.5319297638091,5.70000000000001,-11.3110817734132));
#70144=CARTESIAN_POINT('Ctrl Pts',(37.4670658763312,5.70000000000001,-11.261804086503));
#70145=CARTESIAN_POINT('Ctrl Pts',(37.4252790635777,5.70000000000002,-11.2300582637362));
#70146=CARTESIAN_POINT('Ctrl Pts',(37.3845539662202,5.69999999999999,-11.1968700068083));
#70147=CARTESIAN_POINT('Ctrl Pts',(37.3449168132708,5.69999999999999,-11.1623261463859));
#70148=CARTESIAN_POINT('Ctrl Pts',(37.3249009813365,5.69999999999999,-11.1448823076354));
#70149=CARTESIAN_POINT('Ctrl Pts',(37.3051626180758,5.69999999999999,-11.1270926610294));
#70150=CARTESIAN_POINT('Ctrl Pts',(37.2857053911122,5.7,-11.1089676468229));
#70151=CARTESIAN_POINT('Ctrl Pts',(37.2676753613394,5.70000000000001,-11.0921721113448));
#70152=CARTESIAN_POINT('Ctrl Pts',(37.2498826753603,5.69999999999999,-11.0750843516763));
#70153=CARTESIAN_POINT('Ctrl Pts',(37.2323538947033,5.69999999999999,-11.0577362182599));
#70154=CARTESIAN_POINT('Ctrl Pts',(37.1711091481097,5.7,-10.9971226447461));
#70155=CARTESIAN_POINT('Ctrl Pts',(37.1130372095074,5.7,-10.9332931219723));
#70156=CARTESIAN_POINT('Ctrl Pts',(37.0582414952906,5.69999999999999,-10.8666339257479));
#70157=CARTESIAN_POINT('Ctrl Pts',(37.0110924346456,5.69999999999999,-10.809276912882));
#70158=CARTESIAN_POINT('Ctrl Pts',(36.9663690199974,5.7,-10.7498237353702));
#70159=CARTESIAN_POINT('Ctrl Pts',(36.9241497379828,5.69999999999999,-10.6884923583133));
#70160=CARTESIAN_POINT('Ctrl Pts',(36.9110147566815,5.69999999999998,-10.6694113495329));
#70161=CARTESIAN_POINT('Ctrl Pts',(36.8981222563253,5.7,-10.650148377145));
#70162=CARTESIAN_POINT('Ctrl Pts',(36.8854748972125,5.70000000000001,-10.6307095675714));
#70163=CARTESIAN_POINT('Ctrl Pts',(36.8750183316657,5.70000000000001,-10.6146379762895));
#70164=CARTESIAN_POINT('Ctrl Pts',(36.8647282092343,5.69999999999999,-10.5984441400613));
#70165=CARTESIAN_POINT('Ctrl Pts',(36.8546183260729,5.7,-10.5821517814802));
#70166=CARTESIAN_POINT('Ctrl Pts',(36.8071375712008,5.70000000000002,-10.5056352212263));
#70167=CARTESIAN_POINT('Ctrl Pts',(36.7635688418601,5.7,-10.4268571011546));
#70168=CARTESIAN_POINT('Ctrl Pts',(36.7240163215064,5.70000000000001,-10.346221435102));
#70169=CARTESIAN_POINT('Ctrl Pts',(36.6838955920464,5.70000000000001,-10.2644273619659));
#70170=CARTESIAN_POINT('Ctrl Pts',(36.6479066092487,5.7,-10.1807213198273));
#70171=CARTESIAN_POINT('Ctrl Pts',(36.6161866100473,5.7,-10.0954787389638));
#70172=CARTESIAN_POINT('Ctrl Pts',(36.584458411875,5.70000000000001,-10.010214124637));
#70173=CARTESIAN_POINT('Ctrl Pts',(36.557000760613,5.70000000000001,-9.92341135179696));
#70174=CARTESIAN_POINT('Ctrl Pts',(36.5339892249958,5.70000000000001,-9.83541163480388));
#70175=CARTESIAN_POINT('Ctrl Pts',(36.5199184927481,5.70000000000001,-9.78160295048657));
#70176=CARTESIAN_POINT('Ctrl Pts',(36.5075108969285,5.7,-9.72734611867408));
#70177=CARTESIAN_POINT('Ctrl Pts',(36.4968152084323,5.70000000000001,-9.67271484734734));
#70178=CARTESIAN_POINT('Ctrl Pts',(36.4942456073919,5.70000000000001,-9.65958987912383));
#70179=CARTESIAN_POINT('Ctrl Pts',(36.4917756758722,5.69999999999998,-9.64644730221114));
#70180=CARTESIAN_POINT('Ctrl Pts',(36.4894073031302,5.69999999999998,-9.63329626042469));
#70181=CARTESIAN_POINT('Ctrl Pts',(36.4726467923812,5.7,-9.54022890944844));
#70182=CARTESIAN_POINT('Ctrl Pts',(36.4609458027478,5.70000000000002,-9.4466211194787));
#70183=CARTESIAN_POINT('Ctrl Pts',(36.4544382976075,5.70000000000002,-9.35287324812201));
#70184=CARTESIAN_POINT('Ctrl Pts',(36.4515913175639,5.70000000000002,-9.31185932448558));
#70185=CARTESIAN_POINT('Ctrl Pts',(36.4497388534778,5.7,-9.27081811781351));
#70186=CARTESIAN_POINT('Ctrl Pts',(36.448894611127,5.7,-9.22978125151666));
#70187=CARTESIAN_POINT('Ctrl Pts',(36.4470147422982,5.70000000000001,-9.13840473420257));
#70188=CARTESIAN_POINT('Ctrl Pts',(36.4501300278111,5.7,-9.04705059907772));
#70189=CARTESIAN_POINT('Ctrl Pts',(36.457994679238,5.7,-8.95599261583192));
#70190=CARTESIAN_POINT('Ctrl Pts',(36.4658593306648,5.7,-8.86493463258612));
#70191=CARTESIAN_POINT('Ctrl Pts',(36.4784735398518,5.70000000000001,-8.77417207849568));
#70192=CARTESIAN_POINT('Ctrl Pts',(36.4956433647121,5.69999999999999,-8.68397016390274));
#70193=CARTESIAN_POINT('Ctrl Pts',(36.5003730644743,5.69999999999998,-8.65912262017583));
#70194=CARTESIAN_POINT('Ctrl Pts',(36.5054487442588,5.69999999999998,-8.63431760414533));
#70195=CARTESIAN_POINT('Ctrl Pts',(36.5108670105061,5.69999999999998,-8.60956066002757));
#70196=CARTESIAN_POINT('Ctrl Pts',(36.514033736065,5.69999999999998,-8.59509137333682));
#70197=CARTESIAN_POINT('Ctrl Pts',(36.5173157137729,5.69999999999999,-8.58064673454195));
#70198=CARTESIAN_POINT('Ctrl Pts',(36.5207107833831,5.69999999999999,-8.5662322749048));
#70199=CARTESIAN_POINT('Ctrl Pts',(36.5424498539559,5.69999999999998,-8.47393462233966));
#70200=CARTESIAN_POINT('Ctrl Pts',(36.5688339721789,5.70000000000001,-8.38281777898905));
#70201=CARTESIAN_POINT('Ctrl Pts',(36.5995785196194,5.7,-8.29317222432108));
#70202=CARTESIAN_POINT('Ctrl Pts',(36.6308667367852,5.69999999999999,-8.20194142680089));
#70203=CARTESIAN_POINT('Ctrl Pts',(36.6666710622638,5.7,-8.11223365464869));
#70204=CARTESIAN_POINT('Ctrl Pts',(36.706745771912,5.70000000000001,-8.02434657747373));
#70205=CARTESIAN_POINT('Ctrl Pts',(36.7473987381782,5.70000000000002,-7.93519133679955));
#70206=CARTESIAN_POINT('Ctrl Pts',(36.7924463811748,5.69999999999998,-7.84790883854002));
#70207=CARTESIAN_POINT('Ctrl Pts',(36.8416854714683,5.69999999999999,-7.76281362595471));
#70208=CARTESIAN_POINT('Ctrl Pts',(36.8710196912118,5.69999999999999,-7.71211809827107));
#70209=CARTESIAN_POINT('Ctrl Pts',(36.90184253833,5.70000000000001,-7.6621990125104));
#70210=CARTESIAN_POINT('Ctrl Pts',(36.9341194258415,5.70000000000001,-7.61312550909832));
#70211=CARTESIAN_POINT('Ctrl Pts',(36.9423623839345,5.70000000000002,-7.60059298619142));
#70212=CARTESIAN_POINT('Ctrl Pts',(36.950701478377,5.69999999999998,-7.58811375585398));
#70213=CARTESIAN_POINT('Ctrl Pts',(36.9591320851161,5.69999999999998,-7.57569504140518));
#70214=CARTESIAN_POINT('Ctrl Pts',(37.0161848823531,5.7,-7.49165335623092));
#70215=CARTESIAN_POINT('Ctrl Pts',(37.0772645446978,5.7,-7.4106154107815));
#70216=CARTESIAN_POINT('Ctrl Pts',(37.1420944926193,5.7,-7.33289755586651));
#70217=CARTESIAN_POINT('Ctrl Pts',(37.2072916133539,5.69999999999999,-7.25473953580667));
#70218=CARTESIAN_POINT('Ctrl Pts',(37.2762819290764,5.70000000000001,-7.17993839635292));
#70219=CARTESIAN_POINT('Ctrl Pts',(37.3488364291232,5.7,-7.10882490265184));
#70220=CARTESIAN_POINT('Ctrl Pts',(37.420303235415,5.69999999999999,-7.03877749999878));
#70221=CARTESIAN_POINT('Ctrl Pts',(37.4952286266382,5.69999999999999,-6.97230716483109));
#70222=CARTESIAN_POINT('Ctrl Pts',(37.5734383173599,5.7,-6.90975177261387));
#70223=CARTESIAN_POINT('Ctrl Pts',(37.642088746257,5.70000000000001,-6.85484227909835));
#70224=CARTESIAN_POINT('Ctrl Pts',(37.713270487887,5.70000000000001,-6.80294912851935));
#70225=CARTESIAN_POINT('Ctrl Pts',(37.7868905613917,5.7,-6.75432276015121));
#70226=CARTESIAN_POINT('Origin',(39.2,5.7,-9.525));
#70227=CARTESIAN_POINT('',(40.6568071307763,5.7,-6.77704737365809));
#70228=CARTESIAN_POINT('',(39.2,5.7,-12.63523));
#70229=CARTESIAN_POINT('Origin',(39.2,5.7,-9.525));
#70230=CARTESIAN_POINT('Ctrl Pts',(40.6568071307763,5.70000000000001,-6.77704737365808));
#70231=CARTESIAN_POINT('Ctrl Pts',(40.6675536326424,5.70000000000001,-6.78439681724126));
#70232=CARTESIAN_POINT('Ctrl Pts',(40.6782480875051,5.70000000000001,-6.79181954081017));
#70233=CARTESIAN_POINT('Ctrl Pts',(40.6888896732699,5.7,-6.79931561182634));
#70234=CARTESIAN_POINT('Ctrl Pts',(40.7723747072434,5.7,-6.85812355241729));
#70235=CARTESIAN_POINT('Ctrl Pts',(40.8526093240026,5.69999999999999,-6.92144304811511));
#70236=CARTESIAN_POINT('Ctrl Pts',(40.9294099877629,5.7,-6.98888738755383));
#70237=CARTESIAN_POINT('Ctrl Pts',(41.0059278390579,5.7,-7.05608336846313));
#70238=CARTESIAN_POINT('Ctrl Pts',(41.0790373165767,5.7,-7.12737486738236));
#70239=CARTESIAN_POINT('Ctrl Pts',(41.1485115022755,5.70000000000001,-7.2024036428382));
#70240=CARTESIAN_POINT('Ctrl Pts',(41.1673345977946,5.70000000000001,-7.22273167968936));
#70241=CARTESIAN_POINT('Ctrl Pts',(41.1858945771364,5.70000000000001,-7.24333894727815));
#70242=CARTESIAN_POINT('Ctrl Pts',(41.2041638506315,5.70000000000001,-7.26419219781226));
#70243=CARTESIAN_POINT('Ctrl Pts',(41.2706073697102,5.69999999999999,-7.3400333827441));
#70244=CARTESIAN_POINT('Ctrl Pts',(41.3332586489075,5.70000000000002,-7.41917632680374));
#70245=CARTESIAN_POINT('Ctrl Pts',(41.3919233565839,5.70000000000001,-7.50125544373537));
#70246=CARTESIAN_POINT('Ctrl Pts',(41.4388414115273,5.7,-7.5668995536343));
#70247=CARTESIAN_POINT('Ctrl Pts',(41.483208740423,5.70000000000001,-7.63442243831006));
#70248=CARTESIAN_POINT('Ctrl Pts',(41.5249027839362,5.70000000000002,-7.70364346292023));
#70249=CARTESIAN_POINT('Ctrl Pts',(41.5463341925284,5.70000000000002,-7.73922418228907));
#70250=CARTESIAN_POINT('Ctrl Pts',(41.5670589402089,5.70000000000001,-7.77525362777195));
#70251=CARTESIAN_POINT('Ctrl Pts',(41.5870581128508,5.70000000000002,-7.81170739628005));
#70252=CARTESIAN_POINT('Ctrl Pts',(41.5951145473919,5.70000000000002,-7.82639237375482));
#70253=CARTESIAN_POINT('Ctrl Pts',(41.6030535695938,5.70000000000002,-7.84114703580276));
#70254=CARTESIAN_POINT('Ctrl Pts',(41.6108663637285,5.70000000000002,-7.85595507323248));
#70255=CARTESIAN_POINT('Ctrl Pts',(41.6565060237786,5.70000000000002,-7.94245854211309));
#70256=CARTESIAN_POINT('Ctrl Pts',(41.697906904009,5.70000000000002,-8.03089833473493));
#70257=CARTESIAN_POINT('Ctrl Pts',(41.734896049887,5.70000000000001,-8.12093975713746));
#70258=CARTESIAN_POINT('Ctrl Pts',(41.7714636499846,5.70000000000001,-8.20995502495378));
#70259=CARTESIAN_POINT('Ctrl Pts',(41.8037196667702,5.69999999999999,-8.30053652523976));
#70260=CARTESIAN_POINT('Ctrl Pts',(41.8314470651491,5.7,-8.39236717500651));
#70261=CARTESIAN_POINT('Ctrl Pts',(41.8583795823913,5.70000000000002,-8.4815652499361));
#70262=CARTESIAN_POINT('Ctrl Pts',(41.8810393953456,5.70000000000003,-8.57194261465344));
#70263=CARTESIAN_POINT('Ctrl Pts',(41.8991793540274,5.70000000000002,-8.66320276814808));
#70264=CARTESIAN_POINT('Ctrl Pts',(41.9098047963858,5.70000000000002,-8.71665820967326));
#70265=CARTESIAN_POINT('Ctrl Pts',(41.9188785638188,5.70000000000001,-8.7704163693359));
#70266=CARTESIAN_POINT('Ctrl Pts',(41.926342968605,5.70000000000001,-8.82441520057859));
#70267=CARTESIAN_POINT('Ctrl Pts',(41.9289015008942,5.70000000000001,-8.84292407801371));
#70268=CARTESIAN_POINT('Ctrl Pts',(41.9312709007728,5.7,-8.86146121090835));
#70269=CARTESIAN_POINT('Ctrl Pts',(41.9334486793056,5.70000000000001,-8.88002403124186));
#70270=CARTESIAN_POINT('Ctrl Pts',(41.9350635864279,5.70000000000002,-8.89378908141335));
#70271=CARTESIAN_POINT('Ctrl Pts',(41.9365720127068,5.70000000000003,-8.90755883338214));
#70272=CARTESIAN_POINT('Ctrl Pts',(41.9379732767689,5.70000000000002,-8.92133132839933));
#70273=CARTESIAN_POINT('Ctrl Pts',(41.9471904729052,5.70000000000001,-9.01192366662318));
#70274=CARTESIAN_POINT('Ctrl Pts',(41.9517768375676,5.70000000000004,-9.10264924907603));
#70275=CARTESIAN_POINT('Ctrl Pts',(41.9515425093424,5.70000000000001,-9.19322849973003));
#70276=CARTESIAN_POINT('Ctrl Pts',(41.9514418239969,5.7,-9.23214828045617));
#70277=CARTESIAN_POINT('Ctrl Pts',(41.9504504972526,5.70000000000003,-9.27104096258455));
#70278=CARTESIAN_POINT('Ctrl Pts',(41.9485505426635,5.70000000000003,-9.30988376714684));
#70279=CARTESIAN_POINT('Ctrl Pts',(41.9439536835233,5.70000000000002,-9.40386227706026));
#70280=CARTESIAN_POINT('Ctrl Pts',(41.9340411346708,5.70000000000004,-9.49755072743953));
#70281=CARTESIAN_POINT('Ctrl Pts',(41.9190010975822,5.70000000000003,-9.59059001157079));
#70282=CARTESIAN_POINT('Ctrl Pts',(41.9039610604935,5.70000000000001,-9.68362929570204));
#70283=CARTESIAN_POINT('Ctrl Pts',(41.8837928305745,5.7,-9.77602030848649));
#70284=CARTESIAN_POINT('Ctrl Pts',(41.85864192099,5.70000000000002,-9.86736982038934));
#70285=CARTESIAN_POINT('Ctrl Pts',(41.8537552257159,5.70000000000003,-9.88511857124902));
#70286=CARTESIAN_POINT('Ctrl Pts',(41.8486803209392,5.70000000000003,-9.90282787810892));
#70287=CARTESIAN_POINT('Ctrl Pts',(41.8434181219726,5.7,-9.92049466307744));
#70288=CARTESIAN_POINT('Ctrl Pts',(41.8394338258671,5.69999999999999,-9.93387114370734));
#70289=CARTESIAN_POINT('Ctrl Pts',(41.8353447148482,5.70000000000001,-9.9472146109527));
#70290=CARTESIAN_POINT('Ctrl Pts',(41.8311523643973,5.70000000000001,-9.96052145256901));
#70291=CARTESIAN_POINT('Ctrl Pts',(41.804022806364,5.70000000000001,-10.0466327488685));
#70292=CARTESIAN_POINT('Ctrl Pts',(41.7725634087528,5.70000000000001,-10.1312469744334));
#70293=CARTESIAN_POINT('Ctrl Pts',(41.7369695874477,5.70000000000001,-10.2140570115954));
#70294=CARTESIAN_POINT('Ctrl Pts',(41.7014462364436,5.70000000000001,-10.2967030975987));
#70295=CARTESIAN_POINT('Ctrl Pts',(41.6618041288342,5.70000000000002,-10.3775528985299));
#70296=CARTESIAN_POINT('Ctrl Pts',(41.6181978547607,5.70000000000001,-10.4562680583345));
#70297=CARTESIAN_POINT('Ctrl Pts',(41.5754612696166,5.69999999999999,-10.5334133132456));
#70298=CARTESIAN_POINT('Ctrl Pts',(41.5289163600446,5.70000000000001,-10.6085087758867));
#70299=CARTESIAN_POINT('Ctrl Pts',(41.4786809385008,5.70000000000001,-10.6811946178604));
#70300=CARTESIAN_POINT('Ctrl Pts',(41.4633843153438,5.70000000000001,-10.703327366016));
#70301=CARTESIAN_POINT('Ctrl Pts',(41.447745351846,5.70000000000001,-10.7252363699564));
#70302=CARTESIAN_POINT('Ctrl Pts',(41.431766999022,5.70000000000001,-10.7469105719195));
#70303=CARTESIAN_POINT('Ctrl Pts',(41.4181638265902,5.70000000000001,-10.7653629061416));
#70304=CARTESIAN_POINT('Ctrl Pts',(41.4043146626224,5.70000000000001,-10.7836450498864));
#70305=CARTESIAN_POINT('Ctrl Pts',(41.3902212496529,5.7,-10.801749916543));
#70306=CARTESIAN_POINT('Ctrl Pts',(41.3820353977903,5.69999999999999,-10.8122657338801));
#70307=CARTESIAN_POINT('Ctrl Pts',(41.3737678280459,5.70000000000001,-10.8227207590788));
#70308=CARTESIAN_POINT('Ctrl Pts',(41.3654268033884,5.70000000000001,-10.833104081773));
#70309=CARTESIAN_POINT('Ctrl Pts',(41.3116872772203,5.70000000000001,-10.9000017189995));
#70310=CARTESIAN_POINT('Ctrl Pts',(41.254815874147,5.69999999999999,-10.964036668235));
#70311=CARTESIAN_POINT('Ctrl Pts',(41.1949561042646,5.69999999999999,-11.0249156502104));
#70312=CARTESIAN_POINT('Ctrl Pts',(41.1360360400568,5.7,-11.0848389264599));
#70313=CARTESIAN_POINT('Ctrl Pts',(41.0742200470205,5.70000000000001,-11.141705013839));
#70314=CARTESIAN_POINT('Ctrl Pts',(41.0096218112891,5.7,-11.1951903084968));
#70315=CARTESIAN_POINT('Ctrl Pts',(40.9469513398941,5.7,-11.2470794752977));
#70316=CARTESIAN_POINT('Ctrl Pts',(40.8816616316492,5.70000000000001,-11.2957868641724));
#70317=CARTESIAN_POINT('Ctrl Pts',(40.8138434619797,5.69999999999999,-11.3409703464158));
#70318=CARTESIAN_POINT('Ctrl Pts',(40.766577340876,5.69999999999998,-11.3724611394292));
#70319=CARTESIAN_POINT('Ctrl Pts',(40.7180827620352,5.7,-11.4022392586719));
#70320=CARTESIAN_POINT('Ctrl Pts',(40.6683886799114,5.7,-11.4301739104629));
#70321=CARTESIAN_POINT('Origin',(39.2,5.7,-9.525));
#70322=CARTESIAN_POINT('Ctrl Pts',(41.099774813423,6.10922971516948,-11.9923764941264));
#70323=CARTESIAN_POINT('Ctrl Pts',(41.9164782428699,6.04232813665392,-11.3635994721406));
#70324=CARTESIAN_POINT('Ctrl Pts',(42.8624587143743,5.90855795765171,-9.24274905943794));
#70325=CARTESIAN_POINT('Ctrl Pts',(40.9620531289813,5.70791917816281,-6.29820309169915));
#70326=CARTESIAN_POINT('Ctrl Pts',(37.4625022647654,5.50731337670284,-6.28846198413748));
#70327=CARTESIAN_POINT('Ctrl Pts',(35.5393356313202,5.30670757524286,-9.20937120381493));
#70328=CARTESIAN_POINT('Ctrl Pts',(36.9350656861766,5.10610177378287,-12.4185714191142));
#70329=CARTESIAN_POINT('Ctrl Pts',(40.3847855154406,4.90549597232289,-13.0029231033536));
#70330=CARTESIAN_POINT('Ctrl Pts',(42.7600675205086,4.70489017086291,-10.4341711122309));
#70331=CARTESIAN_POINT('Ctrl Pts',(41.9072757812719,4.50428436940293,-7.04073827364627));
#70332=CARTESIAN_POINT('Ctrl Pts',(38.5995975862866,4.30367856794295,-5.90008259990626));
#70333=CARTESIAN_POINT('Ctrl Pts',(35.8363575143004,4.10307276648297,-8.04629210832045));
#70334=CARTESIAN_POINT('Ctrl Pts',(36.1231331479275,3.90246696502298,-11.5333752820698));
#70335=CARTESIAN_POINT('Ctrl Pts',(39.1998994778117,3.701861163563,-13.1993206345152));
#70336=CARTESIAN_POINT('Ctrl Pts',(42.2767548315279,3.50125536210303,-11.5335406820516));
#70337=CARTESIAN_POINT('Ctrl Pts',(42.5637263103221,3.30064956064303,-8.0464869970296));
#70338=CARTESIAN_POINT('Ctrl Pts',(39.800597384115,3.10004375918305,-5.90009555072928));
#70339=CARTESIAN_POINT('Ctrl Pts',(36.4928697401343,2.89943795772307,-7.04062911559291));
#70340=CARTESIAN_POINT('Ctrl Pts',(35.6398653250698,2.69883215626309,-10.4338969393871));
#70341=CARTESIAN_POINT('Ctrl Pts',(38.0150565132925,2.49822635480311,-13.0030110403416));
#70342=CARTESIAN_POINT('Ctrl Pts',(41.4647096194439,2.29762055334312,-12.4183963930662));
#70343=CARTESIAN_POINT('Ctrl Pts',(42.8608096815054,2.09701475188314,-9.21015919524167));
#70344=CARTESIAN_POINT('Ctrl Pts',(40.9374259147327,1.89640895042316,-6.28740778173331));
#70345=CARTESIAN_POINT('Ctrl Pts',(37.4386100185307,1.69580314896318,-6.30038256839133));
#70346=CARTESIAN_POINT('Ctrl Pts',(35.5369559639688,1.4951973475032,-9.23731854427653));
#70347=CARTESIAN_POINT('Ctrl Pts',(36.9568117578627,1.29459154604321,-12.4351131820842));
#70348=CARTESIAN_POINT('Ctrl Pts',(40.410705843259,1.09398574458323,-12.9941272089789));
#70349=CARTESIAN_POINT('Ctrl Pts',(42.76677764218,0.893379943123255,-10.4074678347248));
#70350=CARTESIAN_POINT('Ctrl Pts',(41.8886303202978,0.692774141663271,-7.02061999125906));
#70351=CARTESIAN_POINT('Ctrl Pts',(38.5725346701973,0.492168340203288,-5.90464925892042));
#70352=CARTESIAN_POINT('Ctrl Pts',(35.8254008592128,0.291562538743307,-8.07147570812169));
#70353=CARTESIAN_POINT('Ctrl Pts',(36.1382259692999,0.090956737283325,-11.5563030332699));
#70354=CARTESIAN_POINT('Ctrl Pts',(39.227352017236,-0.109649064176656,-13.19922156318));
#70355=CARTESIAN_POINT('Ctrl Pts',(42.291676290017,-0.310254865636639,-11.510494886889));
#70356=CARTESIAN_POINT('Ctrl Pts',(42.5525853866673,-0.510860667096621,
-8.02139651063807));
#70357=CARTESIAN_POINT('Ctrl Pts',(39.7734968022572,-0.711466468556603,
-5.89570893342317));
#70358=CARTESIAN_POINT('Ctrl Pts',(36.4743829991325,-0.912072270016586,
-7.06092528670388));
#70359=CARTESIAN_POINT('Ctrl Pts',(35.6467556479424,-1.11267807147657,-10.4604714333933));
#70360=CARTESIAN_POINT('Ctrl Pts',(38.0410759415337,-1.31328387293655,-13.0117674506389));
#70361=CARTESIAN_POINT('Ctrl Pts',(41.4862647571546,-1.51388967439654,-12.4013945640885));
#70362=CARTESIAN_POINT('Ctrl Pts',(42.8583551253254,-1.71449547585652,-9.18281583155971));
#70363=CARTESIAN_POINT('Ctrl Pts',(40.9131873733246,-1.9151012773165,-6.27451676638583));
#70364=CARTESIAN_POINT('Ctrl Pts',(37.4145660798143,-2.11570707877648,-6.31363300995112));
#70365=CARTESIAN_POINT('Ctrl Pts',(35.5349087651602,-2.31631288023646,-9.26469543141597));
#70366=CARTESIAN_POINT('Ctrl Pts',(36.9786176201205,-2.51691868169644,-12.4517921946197));
#70367=CARTESIAN_POINT('Ctrl Pts',(40.4365920357559,-2.71752448315643,-12.9849844458076));
#70368=CARTESIAN_POINT('Ctrl Pts',(42.7732715438646,-2.91813028461641,-10.3807936094251));
#70369=CARTESIAN_POINT('Ctrl Pts',(41.8698435068077,-3.11873608607639,-7.00060148207879));
#70370=CARTESIAN_POINT('Ctrl Pts',(38.5455023136619,-3.31934188753637,-5.90943849358033));
#70371=CARTESIAN_POINT('Ctrl Pts',(35.8146348786017,-3.51994768899636,-8.09672998948182));
#70372=CARTESIAN_POINT('Ctrl Pts',(36.1534885487898,-3.72055349045633,-11.5791227338624));
#70373=CARTESIAN_POINT('Ctrl Pts',(39.2548036267735,-3.92115929191632,-13.198914641172));
#70374=CARTESIAN_POINT('Ctrl Pts',(42.3064248479004,-4.1217650933763,-11.4873396475821));
#70375=CARTESIAN_POINT('Ctrl Pts',(42.541257458194,-4.32237089483629,-7.99638924961627));
#70376=CARTESIAN_POINT('Ctrl Pts',(39.7463641247024,-4.52297669629626,-5.89152528956596));
#70377=CARTESIAN_POINT('Ctrl Pts',(36.4560484587279,-4.72358249775625,-7.08135883009064));
#70378=CARTESIAN_POINT('Ctrl Pts',(35.6538443127724,-4.92418829921622,-10.4869937993917));
#70379=CARTESIAN_POINT('Ctrl Pts',(38.067160078324,-5.12479410067622,-13.0203291604629));
#70380=CARTESIAN_POINT('Ctrl Pts',(41.5076922567986,-5.32539990213619,-12.3842321829538));
#70381=CARTESIAN_POINT('Ctrl Pts',(42.8556963412319,-5.52600570359617,-9.15549155783884));
#70382=CARTESIAN_POINT('Ctrl Pts',(40.8888531903923,-5.72661150505615,-6.26180721847069));
#70383=CARTESIAN_POINT('Ctrl Pts',(37.390621815149,-5.92721730651614,-6.3270627253933));
#70384=CARTESIAN_POINT('Ctrl Pts',(35.5330661727275,-6.12782310797612,-9.29208685197852));
#70385=CARTESIAN_POINT('Ctrl Pts',(37.0005474930735,-6.32842890943611,-12.4683078156879));
#70386=CARTESIAN_POINT('Ctrl Pts',(40.4624091943875,-6.52903471089608,-12.9756485265975));
#70387=CARTESIAN_POINT('Ctrl Pts',(42.7795659647536,-6.72964051235607,-10.354071608499));
#70388=CARTESIAN_POINT('Ctrl Pts',(41.8509076470888,-6.93024631381605,-6.98072389967437));
#70389=CARTESIAN_POINT('Ctrl Pts',(38.5185064949806,-7.13085211527603,-5.91442956983856));
#70390=CARTESIAN_POINT('Ctrl Pts',(35.8040578888541,-7.33145791673602,-8.12206400532603));
#70391=CARTESIAN_POINT('Ctrl Pts',(36.1689212021761,-7.532063718196,-11.6018277611446));
#70392=CARTESIAN_POINT('Ctrl Pts',(39.2822521770986,-7.73266951965597,-13.1984026202339));
#70393=CARTESIAN_POINT('Ctrl Pts',(42.3209999865671,-7.93327532111597,-11.4640748582897));
#70394=CARTESIAN_POINT('Ctrl Pts',(42.5297430022072,-8.13388112257593,-7.97146732602006));
#70395=CARTESIAN_POINT('Ctrl Pts',(39.7192009440691,-8.33448692403593,-5.88754448456992));
#70396=CARTESIAN_POINT('Ctrl Pts',(36.4378671053041,-8.5350927254959,-7.10192879737212));
#70397=CARTESIAN_POINT('Ctrl Pts',(35.6611309375955,-8.73569852695589,-10.513462450324));
#70398=CARTESIAN_POINT('Ctrl Pts',(38.093307470686,-8.93630432841588,-13.0286957621018));
#70399=CARTESIAN_POINT('Ctrl Pts',(41.5289909005289,-9.13691012987584,-12.3669101408529));
#70400=CARTESIAN_POINT('Ctrl Pts',(42.8528335278548,-9.33751593133584,-9.12818799432527));
#70401=CARTESIAN_POINT('Ctrl Pts',(40.8644246221869,-9.53812173279581,-6.24927968040188));
#70402=CARTESIAN_POINT('Ctrl Pts',(37.3667787632686,-9.73872753425581,-6.34067128246068));
#70403=CARTESIAN_POINT('Ctrl Pts',(35.5314278932901,-9.93933333571576,-9.31949066061397));
#70404=CARTESIAN_POINT('Ctrl Pts',(37.0226009281239,-10.1399391371757,-12.4846603262167));
#70405=CARTESIAN_POINT('Ctrl Pts',(40.4881543603094,-10.3405449386357,-12.9661176206786));
#70406=CARTESIAN_POINT('Ctrl Pts',(42.785663522224,-10.5411507400957,-10.3273079236824));
#70407=CARTESIAN_POINT('Ctrl Pts',(41.8318179907986,-10.7417565415557,-6.9609793558109));
#70408=CARTESIAN_POINT('Ctrl Pts',(38.4915600815517,-10.9423623430157,-5.91963981024859));
#70409=CARTESIAN_POINT('Ctrl Pts',(35.7936482578035,-11.1429681444757,-8.14744191072689));
#70410=CARTESIAN_POINT('Ctrl Pts',(36.1845665389655,-11.3435739459356,-11.6244841995046));
#70411=CARTESIAN_POINT('Ctrl Pts',(39.3096110991439,-11.5441797473956,-13.1975537759688));
#70412=CARTESIAN_POINT('Ctrl Pts',(42.3355672427447,-11.7447855488556,-11.4409595689041));
#70413=CARTESIAN_POINT('Ctrl Pts',(42.5177171990917,-11.9453913503156,-7.94612769865488));
#70414=CARTESIAN_POINT('Ctrl Pts',(39.6926460209969,-12.1459971517755,-5.88475596888554));
#70415=CARTESIAN_POINT('Ctrl Pts',(36.4185870787412,-12.3466029532356,-7.12067230223758));
#70416=CARTESIAN_POINT('Ctrl Pts',(35.6711340431576,-12.5472087546955,-10.5439995150024));
#70417=CARTESIAN_POINT('Ctrl Pts',(37.2996374022545,-12.6809459556688,-12.1983898865047));
#70418=CARTESIAN_POINT('Ctrl Pts',(38.2842826159495,-12.7478145561555,-12.5013321319679));
#70419=CARTESIAN_POINT('Ctrl Pts',(40.9548065210116,5.97203701228902,-11.8040955702177));
#70420=CARTESIAN_POINT('Ctrl Pts',(41.7091888265352,5.90513543377346,-11.2232993565576));
#70421=CARTESIAN_POINT('Ctrl Pts',(42.5829832828131,5.77136525477125,-9.26428710520824));
#70422=CARTESIAN_POINT('Ctrl Pts',(40.8275941228708,5.57072647528236,-6.54443397888103));
#70423=CARTESIAN_POINT('Ctrl Pts',(37.5950874943231,5.37012067382238,-6.53543619717014));
#70424=CARTESIAN_POINT('Ctrl Pts',(35.8186741396894,5.16951487236241,-9.2334562518404));
#70425=CARTESIAN_POINT('Ctrl Pts',(37.1078986227854,4.96890907090242,-12.1977683509632));
#70426=CARTESIAN_POINT('Ctrl Pts',(40.2943767302342,4.76830326944244,-12.7375292420027));
#70427=CARTESIAN_POINT('Ctrl Pts',(42.4884053710417,4.56769746798245,-10.3647939509386));
#70428=CARTESIAN_POINT('Ctrl Pts',(41.7006885877136,4.36709166652247,-7.23030767830835));
#70429=CARTESIAN_POINT('Ctrl Pts',(38.6454131808827,4.16648586506249,-6.17669332340427));
#70430=CARTESIAN_POINT('Ctrl Pts',(36.0930308336797,3.96588006360251,-8.15912956490612));
#70431=CARTESIAN_POINT('Ctrl Pts',(36.3579231506009,3.76527426214253,-11.3801198893222));
#70432=CARTESIAN_POINT('Ctrl Pts',(39.1999071484734,3.56466846068254,-12.918940041829));
#70433=CARTESIAN_POINT('Ctrl Pts',(42.0419733769346,3.36406265922256,-11.3802726679382));
#70434=CARTESIAN_POINT('Ctrl Pts',(42.3070465944413,3.16345685776258,-8.15930958201932));
#70435=CARTESIAN_POINT('Ctrl Pts',(39.7547669116891,2.9628510563026,-6.17670528597399));
#70436=CARTESIAN_POINT('Ctrl Pts',(36.6994458292241,2.76224525484262,-7.23020684990363));
#70437=CARTESIAN_POINT('Ctrl Pts',(35.9115325989661,2.56163945338263,-10.364540699716));
#70438=CARTESIAN_POINT('Ctrl Pts',(38.1054773529932,2.36103365192266,-12.7376104686823));
#70439=CARTESIAN_POINT('Ctrl Pts',(41.2918938288466,2.16042785046267,-12.1976066808283));
#70440=CARTESIAN_POINT('Ctrl Pts',(42.5814600845839,1.95982204900269,-9.23418411310284));
#70441=CARTESIAN_POINT('Ctrl Pts',(40.8048461656643,1.75921624754271,-6.53446243899614));
#70442=CARTESIAN_POINT('Ctrl Pts',(37.5730184210845,1.55861044608272,-6.54644714374924));
#70443=CARTESIAN_POINT('Ctrl Pts',(35.81647606034,1.35800464462275,-9.25927098258661));
#70444=CARTESIAN_POINT('Ctrl Pts',(37.1279852920744,1.15739884316276,-12.2130478426818));
#70445=CARTESIAN_POINT('Ctrl Pts',(40.3183191259124,0.956793041702779,-12.7294045460136));
#70446=CARTESIAN_POINT('Ctrl Pts',(42.4946034557738,0.756187240242797,-10.340128351011));
#70447=CARTESIAN_POINT('Ctrl Pts',(41.6834659272838,0.555581438782815,-7.21172458473581));
#70448=CARTESIAN_POINT('Ctrl Pts',(38.6204153857253,0.354975637322832,-6.18091150913903));
#70449=CARTESIAN_POINT('Ctrl Pts',(36.0829102606201,0.154369835862851,-8.18239145091573));
#70450=CARTESIAN_POINT('Ctrl Pts',(36.3718642667677,-0.0462359655971322,
-11.4012980663534));
#70451=CARTESIAN_POINT('Ctrl Pts',(39.2252648355318,-0.246841767057112,
-12.9188485304437));
#70452=CARTESIAN_POINT('Ctrl Pts',(42.0557562066018,-0.447447568517095,
-11.3589854546603));
#70453=CARTESIAN_POINT('Ctrl Pts',(42.2967558140069,-0.648053369977079,
-8.13613370410783));
#70454=CARTESIAN_POINT('Ctrl Pts',(39.7297343249682,-0.848659171437058,
-6.17265340329844));
#70455=CARTESIAN_POINT('Ctrl Pts',(36.6823697771398,-1.04926497289704,-7.24895425784137));
#70456=CARTESIAN_POINT('Ctrl Pts',(35.91789713408,-1.24987077435702,-10.3890873433735));
#70457=CARTESIAN_POINT('Ctrl Pts',(38.1295112869248,-1.45047657581701,-12.7456986935507));
#70458=CARTESIAN_POINT('Ctrl Pts',(41.3118041339779,-1.65108237727699,-12.1819022298859));
#70459=CARTESIAN_POINT('Ctrl Pts',(42.5791928310334,-1.85168817873697,-9.20892727078845));
#70460=CARTESIAN_POINT('Ctrl Pts',(40.7824572223946,-2.05229398019695,-6.52255511312024));
#70461=CARTESIAN_POINT('Ctrl Pts',(37.5508092307361,-2.25289978165693,-6.5586864686898));
#70462=CARTESIAN_POINT('Ctrl Pts',(35.8145850794753,-2.45350558311692,-9.28455879024563));
#70463=CARTESIAN_POINT('Ctrl Pts',(37.1481271894279,-2.65411138457689,-12.2284541107061));
#70464=CARTESIAN_POINT('Ctrl Pts',(40.3422299910721,-2.85471718603688,-12.7209594501424));
#70465=CARTESIAN_POINT('Ctrl Pts',(42.5006018198656,-3.05532298749686,-10.3154895863701));
#70466=CARTESIAN_POINT('Ctrl Pts',(41.6661127006862,-3.25592878895684,-7.19323365086183));
#70467=CARTESIAN_POINT('Ctrl Pts',(38.595445818179,-3.45653459041683,-6.18533528618488));
#70468=CARTESIAN_POINT('Ctrl Pts',(36.0729658120213,-3.65714039187681,-8.20571862490556));
#70469=CARTESIAN_POINT('Ctrl Pts',(36.3859621871249,-3.85774619333678,-11.4223764379185));
#70470=CARTESIAN_POINT('Ctrl Pts',(39.2506216636613,-4.05835199479678,-12.9185650290848));
#70471=CARTESIAN_POINT('Ctrl Pts',(42.0693793293881,-4.25895779625675,-11.3375971487179));
#70472=CARTESIAN_POINT('Ctrl Pts',(42.286292298745,-4.45956359771674,-8.11303470079247));
#70473=CARTESIAN_POINT('Ctrl Pts',(39.7046720917133,-4.66016939917672,-6.16878900554438));
#70474=CARTESIAN_POINT('Ctrl Pts',(36.6654343115076,-4.8607752006367,-7.26782855543132));
#70475=CARTESIAN_POINT('Ctrl Pts',(35.9244448760446,-5.06138100209668,-10.413585836815));
#70476=CARTESIAN_POINT('Ctrl Pts',(38.1536049916162,-5.26198680355667,-12.7536070751778));
#70477=CARTESIAN_POINT('Ctrl Pts',(41.3315965408666,-5.46259260501664,-12.1660494782237));
#70478=CARTESIAN_POINT('Ctrl Pts',(42.5767369338228,-5.66319840647663,-9.18368806171562));
#70479=CARTESIAN_POINT('Ctrl Pts',(40.7599799358282,-5.8638042079366,-6.51081540723351));
#70480=CARTESIAN_POINT('Ctrl Pts',(37.528692108497,-6.0644100093966,-6.57109138745532));
#70481=CARTESIAN_POINT('Ctrl Pts',(35.8128830918537,-6.26501581085657,-9.30986002230918));
#70482=CARTESIAN_POINT('Ctrl Pts',(37.16838363445,-6.46562161231656,-12.2437094553629));
#70483=CARTESIAN_POINT('Ctrl Pts',(40.3660770902129,-6.66622741377654,-12.7123359376115));
#70484=CARTESIAN_POINT('Ctrl Pts',(42.506415925171,-6.86683321523652,-10.2908066917722));
#70485=CARTESIAN_POINT('Ctrl Pts',(41.6486218013013,-7.06743901669651,-7.1748728899028));
#70486=CARTESIAN_POINT('Ctrl Pts',(38.5705100003509,-7.26804481815648,-6.18994550267102));
#70487=CARTESIAN_POINT('Ctrl Pts',(36.0631959327435,-7.46865061961647,-8.22911944898889));
#70488=CARTESIAN_POINT('Ctrl Pts',(36.400217203355,-7.66925642107645,-11.4433488866808));
#70489=CARTESIAN_POINT('Ctrl Pts',(39.2759756660211,-7.86986222253643,-12.9180920795149));
#70490=CARTESIAN_POINT('Ctrl Pts',(42.0828422662563,-8.07046802399641,-11.3161076523461));
#70491=CARTESIAN_POINT('Ctrl Pts',(42.2756564895382,-8.27107382545639,-8.09001452296202));
#70492=CARTESIAN_POINT('Ctrl Pts',(39.6795816830134,-8.47167962691638,-6.16511196839422));
#70493=CARTESIAN_POINT('Ctrl Pts',(36.6486403434418,-8.67228542837637,-7.28682886666163));
#70494=CARTESIAN_POINT('Ctrl Pts',(35.9311754720423,-8.87289122983634,-10.4380347140871));
#70495=CARTESIAN_POINT('Ctrl Pts',(38.1777571249638,-9.07349703129632,-12.7613352369636));
#70496=CARTESIAN_POINT('Ctrl Pts',(41.3512699245974,-9.27410283275631,-12.1500492490276));
#70497=CARTESIAN_POINT('Ctrl Pts',(42.5740925764247,-9.47470863421628,-9.15846798249258));
#70498=CARTESIAN_POINT('Ctrl Pts',(40.7374154663536,-9.67531443567627,-6.49924382235935));
#70499=CARTESIAN_POINT('Ctrl Pts',(37.5066684756828,-9.87592023713625,-6.58366150077329));
#70500=CARTESIAN_POINT('Ctrl Pts',(35.8113698264815,-10.0765260385962,-9.33517269713481));
#70501=CARTESIAN_POINT('Ctrl Pts',(37.1887542127754,-10.2771318400562,-12.2588141361429));
#70502=CARTESIAN_POINT('Ctrl Pts',(40.389857690274,-10.4777376415162,-12.7035323174459));
#70503=CARTESIAN_POINT('Ctrl Pts',(42.5120481893403,-10.6783434429762,-10.266085294104));
#70504=CARTESIAN_POINT('Ctrl Pts',(41.6309888412761,-10.8789492444362,-7.15663501556043));
#70505=CARTESIAN_POINT('Ctrl Pts',(38.5456198177521,-11.0795550458962,-6.19475815929904));
#70506=CARTESIAN_POINT('Ctrl Pts',(36.0535806413312,-11.2801608473562,-8.2525608134982));
#70507=CARTESIAN_POINT('Ctrl Pts',(36.4146686735121,-11.4807666488161,-11.4642764542515));
#70508=CARTESIAN_POINT('Ctrl Pts',(39.301246879469,-11.6813724502761,-12.9173080089812));
#70509=CARTESIAN_POINT('Ctrl Pts',(42.0962979221335,-11.8819782517361,-11.2947562478204));
#70510=CARTESIAN_POINT('Ctrl Pts',(42.2645483531536,-12.0825840531961,-8.06660851556254));
#70511=CARTESIAN_POINT('Ctrl Pts',(39.6550531168681,-12.2831898546561,-6.16253623916968));
#70512=CARTESIAN_POINT('Ctrl Pts',(36.6308315399463,-12.483795656116,-7.30414208943529));
#70513=CARTESIAN_POINT('Ctrl Pts',(35.9404152591722,-12.684401457576,-10.4662415519984));
#70514=CARTESIAN_POINT('Ctrl Pts',(37.4446505473975,-12.8181386585493,-11.9943884627264));
#70515=CARTESIAN_POINT('Ctrl Pts',(38.3541593111027,-12.885007259036,-12.2742137473193));
#70516=CARTESIAN_POINT('Ctrl Pts',(40.8098382286002,5.83484430940857,-11.6158146463091));
#70517=CARTESIAN_POINT('Ctrl Pts',(41.5018994102006,5.76794273089301,-11.0829992409746));
#70518=CARTESIAN_POINT('Ctrl Pts',(42.303507851252,5.63417255189079,-9.28582515097854));
#70519=CARTESIAN_POINT('Ctrl Pts',(40.6931351167602,5.43353377240191,-6.79066486606293));
#70520=CARTESIAN_POINT('Ctrl Pts',(37.7276727238809,5.23292797094192,-6.78241041020279));
#70521=CARTESIAN_POINT('Ctrl Pts',(36.0980126480587,5.03232216948195,-9.25754129986588));
#70522=CARTESIAN_POINT('Ctrl Pts',(37.280731559394,4.83171636802196,-11.9769652828124));
#70523=CARTESIAN_POINT('Ctrl Pts',(40.2039679450279,4.63111056656198,-12.4721353806518));
#70524=CARTESIAN_POINT('Ctrl Pts',(42.2167432215747,4.43050476510199,-10.2954167896462));
#70525=CARTESIAN_POINT('Ctrl Pts',(41.4941013941553,4.22989896364201,-7.41987708297046));
#70526=CARTESIAN_POINT('Ctrl Pts',(38.6912287754788,4.02929316218203,-6.45330404690225));
#70527=CARTESIAN_POINT('Ctrl Pts',(36.3497041530591,3.82868736072205,-8.27196702149181));
#70528=CARTESIAN_POINT('Ctrl Pts',(36.5927131532743,3.62808155926206,-11.2268644965746));
#70529=CARTESIAN_POINT('Ctrl Pts',(39.1999148191352,3.42747575780209,-12.6385594491428));
#70530=CARTESIAN_POINT('Ctrl Pts',(41.8071919223413,3.2268699563421,-11.2270046538248));
#70531=CARTESIAN_POINT('Ctrl Pts',(42.0503668785605,3.02626415488212,-8.27213216700902));
#70532=CARTESIAN_POINT('Ctrl Pts',(39.7089364392632,2.82565835342213,-6.4533150212187));
#70533=CARTESIAN_POINT('Ctrl Pts',(36.9060219183138,2.62505255196216,-7.41978458421434));
#70534=CARTESIAN_POINT('Ctrl Pts',(36.1831998728624,2.42444675050217,-10.2951844600449));
#70535=CARTESIAN_POINT('Ctrl Pts',(38.1958981926941,2.22384094904219,-12.4722098970229));
#70536=CARTESIAN_POINT('Ctrl Pts',(41.1190780382492,2.02323514758221,-11.9768169685905));
#70537=CARTESIAN_POINT('Ctrl Pts',(42.3021104876626,1.82262934612223,-9.25820903096404));
#70538=CARTESIAN_POINT('Ctrl Pts',(40.6722664165957,1.62202354466224,-6.78151709625895));
#70539=CARTESIAN_POINT('Ctrl Pts',(37.7074268236383,1.42141774320227,-6.79251171910715));
#70540=CARTESIAN_POINT('Ctrl Pts',(36.0959961567111,1.22081194174228,-9.28122342089669));
#70541=CARTESIAN_POINT('Ctrl Pts',(37.2991588262862,1.0202061402823,-11.9909825032795));
#70542=CARTESIAN_POINT('Ctrl Pts',(40.2259324085659,0.81960033882232,-12.4646818830482));
#70543=CARTESIAN_POINT('Ctrl Pts',(42.2224292693677,0.61899453736234,-10.2727888672974));
#70544=CARTESIAN_POINT('Ctrl Pts',(41.4783015342697,0.418388735902356,-7.40282917821255));
#70545=CARTESIAN_POINT('Ctrl Pts',(38.6682961012533,0.217782934442375,-6.45717375935766));
#70546=CARTESIAN_POINT('Ctrl Pts',(36.3404196620272,0.017177132982393,-8.29330719370977));
#70547=CARTESIAN_POINT('Ctrl Pts',(36.6055025642355,-0.183428668477588,
-11.246293099437));
#70548=CARTESIAN_POINT('Ctrl Pts',(39.2231776538277,-0.384034469937571,
-12.6384754977072));
#70549=CARTESIAN_POINT('Ctrl Pts',(41.8198361231866,-0.584640271397551,
-11.2074760224316));
#70550=CARTESIAN_POINT('Ctrl Pts',(42.0409262413466,-0.785246072857537,
-8.25087089757759));
#70551=CARTESIAN_POINT('Ctrl Pts',(39.6859718476791,-0.985851874317515,
-6.44959787317372));
#70552=CARTESIAN_POINT('Ctrl Pts',(36.8903565551472,-1.18645767577751,-7.43698322897887));
#70553=CARTESIAN_POINT('Ctrl Pts',(36.1890386202178,-1.38706347723748,-10.3177032533537));
#70554=CARTESIAN_POINT('Ctrl Pts',(38.217946632316,-1.58766927869747,-12.4796299364624));
#70555=CARTESIAN_POINT('Ctrl Pts',(41.1373435108012,-1.78827508015745,-11.9624098956833));
#70556=CARTESIAN_POINT('Ctrl Pts',(42.3000305367416,-1.98888088161743,-9.23503871001721));
#70557=CARTESIAN_POINT('Ctrl Pts',(40.6517270714646,-2.18948668307741,-6.77059345985466));
#70558=CARTESIAN_POINT('Ctrl Pts',(37.6870523816581,-2.3900924845374,-6.80373992742849));
#70559=CARTESIAN_POINT('Ctrl Pts',(36.0942613937905,-2.59069828599738,-9.30442214907529));
#70560=CARTESIAN_POINT('Ctrl Pts',(37.3176367587351,-2.79130408745736,-12.0051160267924));
#70561=CARTESIAN_POINT('Ctrl Pts',(40.2478679463885,-2.99190988891734,-12.4569344544771));
#70562=CARTESIAN_POINT('Ctrl Pts',(42.2279320958664,-3.19251569037733,-10.2501855633152));
#70563=CARTESIAN_POINT('Ctrl Pts',(41.4623818945649,-3.3931214918373,-7.38586581964484));
#70564=CARTESIAN_POINT('Ctrl Pts',(38.645389322696,-3.59372729329729,-6.46123207878943));
#70565=CARTESIAN_POINT('Ctrl Pts',(36.3312967454408,-3.79433309475727,-8.31470726032929));
#70566=CARTESIAN_POINT('Ctrl Pts',(36.61843582546,-3.99493889621725,-11.2656301419746));
#70567=CARTESIAN_POINT('Ctrl Pts',(39.246439700549,-4.19554469767724,-12.6382154169976));
#70568=CARTESIAN_POINT('Ctrl Pts',(41.8323338108756,-4.39615049913721,-11.1878546498535));
#70569=CARTESIAN_POINT('Ctrl Pts',(42.0313271392962,-4.5967563005972,-8.22968015196867));
#70570=CARTESIAN_POINT('Ctrl Pts',(39.6629800587242,-4.79736210205718,-6.4460527215228));
#70571=CARTESIAN_POINT('Ctrl Pts',(36.8748201642874,-4.99796790351717,-7.45429828077202));
#70572=CARTESIAN_POINT('Ctrl Pts',(36.1950454393167,-5.19857370497714,-10.3401778742381));
#70573=CARTESIAN_POINT('Ctrl Pts',(38.2400499049083,-5.39917950643713,-12.4868849898927));
#70574=CARTESIAN_POINT('Ctrl Pts',(41.1555008249347,-5.59978530789711,-11.9478667734935));
#70575=CARTESIAN_POINT('Ctrl Pts',(42.2977775264137,-5.80039110935709,-9.21188456559238));
#70576=CARTESIAN_POINT('Ctrl Pts',(40.631106681264,-6.00099691081707,-6.75982359599637));
#70577=CARTESIAN_POINT('Ctrl Pts',(37.6667624018449,-6.20160271227705,-6.81512004951732));
#70578=CARTESIAN_POINT('Ctrl Pts',(36.0927000109799,-6.40220851373704,-9.32763319263987));
#70579=CARTESIAN_POINT('Ctrl Pts',(37.3362197758266,-6.60281431519701,-12.0191110950378));
#70580=CARTESIAN_POINT('Ctrl Pts',(40.2697449860384,-6.803420116657,-12.4490233486254));
#70581=CARTESIAN_POINT('Ctrl Pts',(42.2332658855884,-7.00402591811698,-10.2275417750453));
#70582=CARTESIAN_POINT('Ctrl Pts',(41.4463359555139,-7.20463171957697,-7.36902188013124));
#70583=CARTESIAN_POINT('Ctrl Pts',(38.6225135057212,-7.40523752103695,-6.46546143550347));
#70584=CARTESIAN_POINT('Ctrl Pts',(36.322333976633,-7.60584332249693,-8.33617489265172));
#70585=CARTESIAN_POINT('Ctrl Pts',(36.631513204534,-7.8064491239569,-11.2848700122171));
#70586=CARTESIAN_POINT('Ctrl Pts',(39.2696991549437,-8.0070549254169,-12.6377815387958));
#70587=CARTESIAN_POINT('Ctrl Pts',(41.8446845459455,-8.20766072687687,-11.1681404464025));
#70588=CARTESIAN_POINT('Ctrl Pts',(42.0215699768691,-8.40826652833686,-8.208561719904));
#70589=CARTESIAN_POINT('Ctrl Pts',(39.6399624219577,-8.60887232979683,-6.44267945221849));
#70590=CARTESIAN_POINT('Ctrl Pts',(36.8594135815794,-8.80947813125683,-7.47172893595116));
#70591=CARTESIAN_POINT('Ctrl Pts',(36.2012200064891,-9.0100839327168,-10.3626069778503));
#70592=CARTESIAN_POINT('Ctrl Pts',(38.2622067792416,-9.21068973417679,-12.4939747118254));
#70593=CARTESIAN_POINT('Ctrl Pts',(41.173548948666,-9.41129553563677,-11.9331883572021));
#70594=CARTESIAN_POINT('Ctrl Pts',(42.2953516249946,-9.61190133709674,-9.18874797065989));
#70595=CARTESIAN_POINT('Ctrl Pts',(40.6104063105204,-9.81250713855674,-6.7492079643168));
#70596=CARTESIAN_POINT('Ctrl Pts',(37.6465581880969,-10.0131129400167,-6.82665171908593));
#70597=CARTESIAN_POINT('Ctrl Pts',(36.0913117596729,-10.2137187414767,-9.35085473365563));
#70598=CARTESIAN_POINT('Ctrl Pts',(37.3549074974267,-10.4143245429366,-12.0329679460693));
#70599=CARTESIAN_POINT('Ctrl Pts',(40.2915610202388,-10.6149303443966,-12.440947014213));
#70600=CARTESIAN_POINT('Ctrl Pts',(42.2384328564565,-10.8155361458566,-10.2048626645257));
#70601=CARTESIAN_POINT('Ctrl Pts',(41.4301596917537,-11.0161419473166,-7.35229067530997));
#70602=CARTESIAN_POINT('Ctrl Pts',(38.5996795539523,-11.2167477487766,-6.46987650834947));
#70603=CARTESIAN_POINT('Ctrl Pts',(36.313513024859,-11.4173535502366,-8.35767971626948));
#70604=CARTESIAN_POINT('Ctrl Pts',(36.6447708080588,-11.6179593516965,-11.3040687089986));
#70605=CARTESIAN_POINT('Ctrl Pts',(39.2928826597942,-11.8185651531565,-12.6370622419936));
#70606=CARTESIAN_POINT('Ctrl Pts',(41.8570286015223,-12.0191709546165,-11.1485529267368));
#70607=CARTESIAN_POINT('Ctrl Pts',(42.0113795072156,-12.2197767560765,-8.18708933247013));
#70608=CARTESIAN_POINT('Ctrl Pts',(39.6174602127394,-12.4203825575364,-6.44031650945386));
#70609=CARTESIAN_POINT('Ctrl Pts',(36.8430760011515,-12.6209883589965,-7.48761187663297));
#70610=CARTESIAN_POINT('Ctrl Pts',(36.2096964751867,-12.8215941604564,-10.3884835889945));
#70611=CARTESIAN_POINT('Ctrl Pts',(37.5896636925404,-12.9553313614297,-11.7903870389479));
#70612=CARTESIAN_POINT('Ctrl Pts',(38.4240360062559,-13.0221999619164,-12.0470953626707));
#70613=CARTESIAN_POINT('Ctrl Pts',(40.6648699361887,5.6976516065281,-11.4275337224004));
#70614=CARTESIAN_POINT('Ctrl Pts',(41.2946099938659,5.63075002801254,-10.9426991253916));
#70615=CARTESIAN_POINT('Ctrl Pts',(42.0240324196909,5.49697984901032,-9.30736319674886));
#70616=CARTESIAN_POINT('Ctrl Pts',(40.5586761106497,5.29634106952145,-7.03689575324481));
#70617=CARTESIAN_POINT('Ctrl Pts',(37.8602579534387,5.09573526806147,-7.02938462323545));
#70618=CARTESIAN_POINT('Ctrl Pts',(36.3773511564279,4.89512946660149,-9.28162634789135));
#70619=CARTESIAN_POINT('Ctrl Pts',(37.4535644960028,4.6945236651415,-11.7561622146614));
#70620=CARTESIAN_POINT('Ctrl Pts',(40.1135591598215,4.49391786368153,-12.2067415193008));
#70621=CARTESIAN_POINT('Ctrl Pts',(41.9450810721079,4.29331206222154,-10.2260396283539));
#70622=CARTESIAN_POINT('Ctrl Pts',(41.2875142005968,4.09270626076156,-7.60944648763255));
#70623=CARTESIAN_POINT('Ctrl Pts',(38.737044370075,3.89210045930158,-6.72991477040025));
#70624=CARTESIAN_POINT('Ctrl Pts',(36.6063774724384,3.6914946578416,-8.3848044780775));
#70625=CARTESIAN_POINT('Ctrl Pts',(36.8275031559477,3.49088885638161,-11.0736091038271));
#70626=CARTESIAN_POINT('Ctrl Pts',(39.199922489797,3.29028305492163,-12.3581788564566));
#70627=CARTESIAN_POINT('Ctrl Pts',(41.5724104677478,3.08967725346165,-11.0737366397114));
#70628=CARTESIAN_POINT('Ctrl Pts',(41.7936871626797,2.88907145200167,-8.38495475199873));
#70629=CARTESIAN_POINT('Ctrl Pts',(39.6631059668373,2.68846565054169,-6.72992475646342));
#70630=CARTESIAN_POINT('Ctrl Pts',(37.1125980074036,2.4878598490817,-7.60936231852505));
#70631=CARTESIAN_POINT('Ctrl Pts',(36.4548671467587,2.28725404762172,-10.2258282203738));
#70632=CARTESIAN_POINT('Ctrl Pts',(38.286319032395,2.08664824616174,-12.2068093253635));
#70633=CARTESIAN_POINT('Ctrl Pts',(40.9462622476518,1.88604244470176,-11.7560272563527));
#70634=CARTESIAN_POINT('Ctrl Pts',(42.0227608907411,1.68543664324178,-9.2822339488252));
#70635=CARTESIAN_POINT('Ctrl Pts',(40.5396866675272,1.48483084178179,-7.02857175352177));
#70636=CARTESIAN_POINT('Ctrl Pts',(37.8418352261923,1.28422504032181,-7.03857629446507));
#70637=CARTESIAN_POINT('Ctrl Pts',(36.3755162530822,1.08361923886183,-9.30317585920677));
#70638=CARTESIAN_POINT('Ctrl Pts',(37.470332360498,0.883013437401846,-11.7689171638771));
#70639=CARTESIAN_POINT('Ctrl Pts',(40.1335456912194,0.682407635941864,-12.1999592200829));
#70640=CARTESIAN_POINT('Ctrl Pts',(41.9502550829617,0.481801834481882,-10.2054493835837));
#70641=CARTESIAN_POINT('Ctrl Pts',(41.2731371412557,0.2811960330219,-7.59393377168929));
#70642=CARTESIAN_POINT('Ctrl Pts',(38.7161768167814,0.0805902315619172,
-6.73343600957629));
#70643=CARTESIAN_POINT('Ctrl Pts',(36.5979290634346,-0.120015569898064,
-8.4042229365038));
#70644=CARTESIAN_POINT('Ctrl Pts',(36.8391408617033,-0.320621371358047,
-11.0912881325205));
#70645=CARTESIAN_POINT('Ctrl Pts',(39.2210904721234,-0.521227172818027,
-12.3581024649709));
#70646=CARTESIAN_POINT('Ctrl Pts',(41.5839160397715,-0.72183297427801,-11.055966590203));
#70647=CARTESIAN_POINT('Ctrl Pts',(41.7850966686863,-0.922438775737993,
-8.36560809104734));
#70648=CARTESIAN_POINT('Ctrl Pts',(39.6422093703901,-1.12304457719797,-6.72654234304899));
#70649=CARTESIAN_POINT('Ctrl Pts',(37.0983433331545,-1.32365037865796,-7.62501220011637));
#70650=CARTESIAN_POINT('Ctrl Pts',(36.4601801063555,-1.52425618011794,-10.2463191633339));
#70651=CARTESIAN_POINT('Ctrl Pts',(38.3063819777072,-1.72486198157792,-12.2135611793742));
#70652=CARTESIAN_POINT('Ctrl Pts',(40.9628828876245,-1.9254677830379,-11.7429175614806));
#70653=CARTESIAN_POINT('Ctrl Pts',(42.0208682424496,-2.12607358449789,-9.26115014924594));
#70654=CARTESIAN_POINT('Ctrl Pts',(40.5209969205346,-2.32667938595786,-7.01863180658909));
#70655=CARTESIAN_POINT('Ctrl Pts',(37.82329553258,-2.52728518741785,-7.04879338616719));
#70656=CARTESIAN_POINT('Ctrl Pts',(36.3739377081057,-2.72789098887783,-9.32428550790495));
#70657=CARTESIAN_POINT('Ctrl Pts',(37.4871463280423,-2.92849679033781,-11.7817779428789));
#70658=CARTESIAN_POINT('Ctrl Pts',(40.1535059017048,-3.12910259179779,-12.1929094588119));
#70659=CARTESIAN_POINT('Ctrl Pts',(41.9552623718673,-3.32970839325778,-10.1848815402601));
#70660=CARTESIAN_POINT('Ctrl Pts',(41.2586510884434,-3.53031419471776,-7.57849798842788));
#70661=CARTESIAN_POINT('Ctrl Pts',(38.6953328272131,-3.73091999617774,-6.73712887139397));
#70662=CARTESIAN_POINT('Ctrl Pts',(36.5896276788603,-3.93152579763772,-8.42369589575305));
#70663=CARTESIAN_POINT('Ctrl Pts',(36.8509094637952,-4.1321315990977,-11.1088838460307));
#70664=CARTESIAN_POINT('Ctrl Pts',(39.2422577374368,-4.33273740055769,-12.3578658049104));
#70665=CARTESIAN_POINT('Ctrl Pts',(41.5952882923632,-4.53334320201766,-11.0381121509893));
#70666=CARTESIAN_POINT('Ctrl Pts',(41.7763619798471,-4.73394900347766,-8.34632560314489));
#70667=CARTESIAN_POINT('Ctrl Pts',(39.6212880257352,-4.93455480493762,-6.72331643750121));
#70668=CARTESIAN_POINT('Ctrl Pts',(37.084206017067,-5.13516060639762,-7.64076800611272));
#70669=CARTESIAN_POINT('Ctrl Pts',(36.465646002589,-5.33576640785759,-10.2667699116612));
#70670=CARTESIAN_POINT('Ctrl Pts',(38.3264948182005,-5.53637220931758,-12.2201629046076));
#70671=CARTESIAN_POINT('Ctrl Pts',(40.9794051090027,-5.73697801077756,-11.7296840687635));
#70672=CARTESIAN_POINT('Ctrl Pts',(42.0188181190045,-5.93758381223754,-9.24008106946917));
#70673=CARTESIAN_POINT('Ctrl Pts',(40.5022334266998,-6.13818961369753,-7.00883178475918));
#70674=CARTESIAN_POINT('Ctrl Pts',(37.8048326951929,-6.3387954151575,-7.05914871157936));
#70675=CARTESIAN_POINT('Ctrl Pts',(36.3725169301061,-6.53940121661749,-9.34540636297052));
#70676=CARTESIAN_POINT('Ctrl Pts',(37.5040559172031,-6.74000701807747,-11.7945127347128));
#70677=CARTESIAN_POINT('Ctrl Pts',(40.1734128818639,-6.94061281953745,-12.1857107596392));
#70678=CARTESIAN_POINT('Ctrl Pts',(41.9601158460058,-7.14121862099744,-10.1642768583185));
#70679=CARTESIAN_POINT('Ctrl Pts',(41.2440501097264,-7.34182442245742,-7.56317087035968));
#70680=CARTESIAN_POINT('Ctrl Pts',(38.6745170110914,-7.5424302239174,-6.74097736833593));
#70681=CARTESIAN_POINT('Ctrl Pts',(36.5814720205227,-7.74303602537738,-8.44323033631458));
#70682=CARTESIAN_POINT('Ctrl Pts',(36.8628092057128,-7.94364182683736,-11.1263911377534));
#70683=CARTESIAN_POINT('Ctrl Pts',(39.2634226438662,-8.14424762829735,-12.3574709980766));
#70684=CARTESIAN_POINT('Ctrl Pts',(41.6065268256346,-8.34485342975733,-11.0201732404588));
#70685=CARTESIAN_POINT('Ctrl Pts',(41.7674834642002,-8.54545923121731,-8.32710891684597));
#70686=CARTESIAN_POINT('Ctrl Pts',(39.6003431609019,-8.74606503267729,-6.72024693604278));
#70687=CARTESIAN_POINT('Ctrl Pts',(37.0701868197171,-8.94667083413728,-7.65662900524067));
#70688=CARTESIAN_POINT('Ctrl Pts',(36.4712645409359,-9.14727663559725,-10.2871792416134));
#70689=CARTESIAN_POINT('Ctrl Pts',(38.3466564335193,-9.34788243705725,-12.2266141866871));
#70690=CARTESIAN_POINT('Ctrl Pts',(40.9958279727346,-9.54848823851721,-11.7163274653768));
#70691=CARTESIAN_POINT('Ctrl Pts',(42.0166106735645,-9.74909403997722,-9.2190279588272));
#70692=CARTESIAN_POINT('Ctrl Pts',(40.4833971546871,-9.94969984143717,-6.99917210627425));
#70693=CARTESIAN_POINT('Ctrl Pts',(37.7864479005111,-10.1503056428972,-7.06964193739857));
#70694=CARTESIAN_POINT('Ctrl Pts',(36.3712536928645,-10.3509114443572,-9.36653677017645));
#70695=CARTESIAN_POINT('Ctrl Pts',(37.5210607820781,-10.5515172458171,-11.8071217559955));
#70696=CARTESIAN_POINT('Ctrl Pts',(40.1932643502035,-10.7521230472771,-12.1783617109801));
#70697=CARTESIAN_POINT('Ctrl Pts',(41.9648175235727,-10.9527288487371,-10.1436400349473));
#70698=CARTESIAN_POINT('Ctrl Pts',(41.2293305422313,-11.1533346501971,-7.54794633505948));
#70699=CARTESIAN_POINT('Ctrl Pts',(38.6537392901525,-11.3539404516571,-6.74499485739993));
#70700=CARTESIAN_POINT('Ctrl Pts',(36.5734454083867,-11.5545462531171,-8.46279861904078));
#70701=CARTESIAN_POINT('Ctrl Pts',(36.8748729426055,-11.755152054577,-11.1438609637455));
#70702=CARTESIAN_POINT('Ctrl Pts',(39.2845184401193,-11.955757856037,-12.356816475006));
#70703=CARTESIAN_POINT('Ctrl Pts',(41.6177592809111,-12.156363657497,-11.0023496056531));
#70704=CARTESIAN_POINT('Ctrl Pts',(41.7582106612774,-12.356969458957,-8.30757014937776));
#70705=CARTESIAN_POINT('Ctrl Pts',(39.5798673086106,-12.557575260417,-6.71809677973804));
#70706=CARTESIAN_POINT('Ctrl Pts',(37.0553204623567,-12.758181061877,-7.67108166383065));
#70707=CARTESIAN_POINT('Ctrl Pts',(36.4789776912014,-12.9587868633369,-10.3107256259906));
#70708=CARTESIAN_POINT('Ctrl Pts',(37.7346768376834,-13.0925240643102,-11.5863856151695));
#70709=CARTESIAN_POINT('Ctrl Pts',(38.4939127014091,-13.1593926647969,-11.8199769780221));
#70710=CARTESIAN_POINT('Ctrl Pts',(40.6132835138381,5.7,-6.75441154943334));
#70711=CARTESIAN_POINT('Ctrl Pts',(40.6277913861508,5.7,-6.76195682417492));
#70712=CARTESIAN_POINT('Ctrl Pts',(40.6422992584636,5.7,-6.7695020989165));
#70713=CARTESIAN_POINT('Ctrl Pts',(40.6568071307763,5.7,-6.77704737365809));
#70714=CARTESIAN_POINT('Origin',(39.2,5.7,-9.525));
#70715=CARTESIAN_POINT('',(39.2,5.9,-12.83523));
#70716=CARTESIAN_POINT('Origin',(39.2,5.9,-9.525));
#70717=CARTESIAN_POINT('Origin',(39.2,5.7,-12.83523));
#70718=CARTESIAN_POINT('Origin',(39.2,5.9,-9.525));
#70719=CARTESIAN_POINT('',(34.4375,5.9,-9.525));
#70720=CARTESIAN_POINT('Origin',(39.2,5.9,-9.525));
#70721=CARTESIAN_POINT('Origin',(39.2,-12.95,-9.525));
#70722=CARTESIAN_POINT('',(36.48977,-13.15,-9.525));
#70723=CARTESIAN_POINT('',(36.28977,-12.95,-9.525));
#70724=CARTESIAN_POINT('Origin',(39.2,-13.15,-9.525));
#70725=CARTESIAN_POINT('Origin',(39.2,-13.15,-9.525));
#70726=CARTESIAN_POINT('Origin',(44.2203188851577,12.25,-10.2071323488364));
#70727=CARTESIAN_POINT('',(43.9012309732892,6.5,-10.2864680464642));
#70728=CARTESIAN_POINT('',(43.9012309732892,11.85,-10.2864680464642));
#70729=CARTESIAN_POINT('',(43.9012309732892,5.9,-10.2864680464642));
#70730=CARTESIAN_POINT('',(43.7424257607688,6.5,-10.3259522194887));
#70731=CARTESIAN_POINT('',(44.2203188851577,6.5,-10.2071323488364));
#70732=CARTESIAN_POINT('',(43.7424257607688,12.,-10.3259522194887));
#70733=CARTESIAN_POINT('',(43.7424257607688,12.25,-10.3259522194887));
#70734=CARTESIAN_POINT('Ctrl Pts',(43.9012309732892,11.85,-10.2864680464642));
#70735=CARTESIAN_POINT('Ctrl Pts',(43.8205579253287,11.9264281650905,-10.3065260063607));
#70736=CARTESIAN_POINT('Ctrl Pts',(43.7424257607688,12.,-10.3259522194887));
#70737=CARTESIAN_POINT('Origin',(43.7424257607688,12.25,-10.3259522194887));
#70738=CARTESIAN_POINT('',(43.8781494645997,11.85,-10.4173697870648));
#70739=CARTESIAN_POINT('',(43.8781494645997,6.5,-10.4173697870648));
#70740=CARTESIAN_POINT('',(43.8781494645997,5.9,-10.4173697870648));
#70741=CARTESIAN_POINT('Ctrl Pts',(43.7424257607688,12.,-10.3259522194887));
#70742=CARTESIAN_POINT('Ctrl Pts',(43.8092018230531,11.9264281650909,-10.3709296627358));
#70743=CARTESIAN_POINT('Ctrl Pts',(43.8781494645997,11.85,-10.4173697870648));
#70744=CARTESIAN_POINT('',(43.7424257607688,6.5,-10.3259522194887));
#70745=CARTESIAN_POINT('Origin',(43.9640075051966,6.5,-10.3650230594638));
#70746=CARTESIAN_POINT('Origin',(39.2,6.5,-9.525));
#70747=CARTESIAN_POINT('Origin',(39.2,12.05,-9.525));
#70748=CARTESIAN_POINT('',(34.5875,12.,-9.525));
#70749=CARTESIAN_POINT('',(34.4379637501835,11.85,-9.45853944452601));
#70750=CARTESIAN_POINT('Ctrl Pts',(34.5875,12.,-9.525));
#70751=CARTESIAN_POINT('Ctrl Pts',(34.5139281650903,11.9264281650903,-9.49230140670682));
#70752=CARTESIAN_POINT('Ctrl Pts',(34.4379637501835,11.85,-9.45853944452601));
#70753=CARTESIAN_POINT('',(34.4987690267108,11.85,-8.76353195353579));
#70754=CARTESIAN_POINT('Origin',(39.2,11.85,-9.525));
#70755=CARTESIAN_POINT('',(34.6575742392312,12.,-8.72404778051128));
#70756=CARTESIAN_POINT('Ctrl Pts',(34.4987690267108,11.85,-8.76353195353579));
#70757=CARTESIAN_POINT('Ctrl Pts',(34.579442074671,11.9264281650901,-8.74347399363938));
#70758=CARTESIAN_POINT('Ctrl Pts',(34.6575742392312,12.,-8.72404778051128));
#70759=CARTESIAN_POINT('',(34.5218505354004,11.85,-8.63263021293523));
#70760=CARTESIAN_POINT('Ctrl Pts',(34.6575742392312,12.,-8.72404778051128));
#70761=CARTESIAN_POINT('Ctrl Pts',(34.5907981769464,11.9264281650903,-8.67907033726385));
#70762=CARTESIAN_POINT('Ctrl Pts',(34.5218505354003,11.85,-8.63263021293522));
#70763=CARTESIAN_POINT('',(34.7024188274238,11.85,-7.95874017286797));
#70764=CARTESIAN_POINT('Origin',(39.2,11.85,-9.525));
#70765=CARTESIAN_POINT('',(34.865667786625,12.,-7.94743208891035));
#70766=CARTESIAN_POINT('Ctrl Pts',(34.7024188274237,11.85,-7.95874017286797));
#70767=CARTESIAN_POINT('Ctrl Pts',(34.7853492986979,11.9264281650903,-7.9529956662175));
#70768=CARTESIAN_POINT('Ctrl Pts',(34.865667786625,12.,-7.94743208891035));
#70769=CARTESIAN_POINT('',(34.7478805248412,11.85,-7.8338351857635));
#70770=CARTESIAN_POINT('Ctrl Pts',(34.865667786625,12.,-7.94743208891035));
#70771=CARTESIAN_POINT('Ctrl Pts',(34.8077164538273,11.9264281650903,-7.89154241256207));
#70772=CARTESIAN_POINT('Ctrl Pts',(34.7478805248412,11.85,-7.83383518576349));
#70773=CARTESIAN_POINT('',(35.0427253561796,11.85,-7.20153840448186));
#70774=CARTESIAN_POINT('Origin',(39.2,11.85,-9.525));
#70775=CARTESIAN_POINT('',(35.2054578250443,12.,-7.21875));
#70776=CARTESIAN_POINT('Ctrl Pts',(35.0427253561796,11.85,-7.20153840448186));
#70777=CARTESIAN_POINT('Ctrl Pts',(35.1253934503629,11.9264281650903,-7.21028189500508));
#70778=CARTESIAN_POINT('Ctrl Pts',(35.2054578250443,12.,-7.21875));
#70779=CARTESIAN_POINT('',(35.1091859116536,11.85,-7.08642534570168));
#70780=CARTESIAN_POINT('Ctrl Pts',(35.2054578250443,12.,-7.21875));
#70781=CARTESIAN_POINT('Ctrl Pts',(35.1580920436562,11.9264281650905,-7.15364627008541));
#70782=CARTESIAN_POINT('Ctrl Pts',(35.1091859116536,11.85,-7.08642534570167));
#70783=CARTESIAN_POINT('',(35.5093485713054,11.85,-6.51493384094727));
#70784=CARTESIAN_POINT('Origin',(39.2,11.85,-9.525));
#70785=CARTESIAN_POINT('',(35.6666200061137,12.,-6.56014215032084));
#70786=CARTESIAN_POINT('Ctrl Pts',(35.5093485713054,11.85,-6.51493384094727));
#70787=CARTESIAN_POINT('Ctrl Pts',(35.5892424601881,11.9264281650904,-6.53789966210907));
#70788=CARTESIAN_POINT('Ctrl Pts',(35.6666200061137,12.,-6.56014215032084));
#70789=CARTESIAN_POINT('',(35.5947886144885,11.85,-6.41311036253237));
#70790=CARTESIAN_POINT('Ctrl Pts',(35.6666200061137,12.,-6.56014215032084));
#70791=CARTESIAN_POINT('Ctrl Pts',(35.6312789614341,11.9264281650902,-6.48780251072884));
#70792=CARTESIAN_POINT('Ctrl Pts',(35.5947886144885,11.85,-6.41311036253236));
#70793=CARTESIAN_POINT('',(36.0881103625324,11.85,-5.91978861448852));
#70794=CARTESIAN_POINT('Origin',(39.2,11.85,-9.525));
#70795=CARTESIAN_POINT('',(36.2351421503208,12.,-5.99162000611371));
#70796=CARTESIAN_POINT('Ctrl Pts',(36.0881103625324,11.85,-5.91978861448852));
#70797=CARTESIAN_POINT('Ctrl Pts',(36.1628025107291,11.9264281650905,-5.95627896143419));
#70798=CARTESIAN_POINT('Ctrl Pts',(36.2351421503208,12.,-5.99162000611371));
#70799=CARTESIAN_POINT('',(36.1899338409473,11.85,-5.83434857130539));
#70800=CARTESIAN_POINT('Ctrl Pts',(36.2351421503208,12.,-5.99162000611371));
#70801=CARTESIAN_POINT('Ctrl Pts',(36.2128996621091,11.9264281650904,-5.91424246018812));
#70802=CARTESIAN_POINT('Ctrl Pts',(36.1899338409473,11.85,-5.83434857130539));
#70803=CARTESIAN_POINT('',(36.7614253457017,11.85,-5.43418591165355));
#70804=CARTESIAN_POINT('Origin',(39.2,11.85,-9.525));
#70805=CARTESIAN_POINT('',(36.89375,12.,-5.53045782504427));
#70806=CARTESIAN_POINT('Ctrl Pts',(36.7614253457017,11.85,-5.43418591165355));
#70807=CARTESIAN_POINT('Ctrl Pts',(36.8286462700852,11.9264281650903,-5.48309204365601));
#70808=CARTESIAN_POINT('Ctrl Pts',(36.89375,12.,-5.53045782504428));
#70809=CARTESIAN_POINT('',(36.8765384044819,11.85,-5.36772535617957));
#70810=CARTESIAN_POINT('Ctrl Pts',(36.89375,12.,-5.53045782504427));
#70811=CARTESIAN_POINT('Ctrl Pts',(36.885281895005,11.9264281650899,-5.45039345036243));
#70812=CARTESIAN_POINT('Ctrl Pts',(36.8765384044819,11.85,-5.36772535617957));
#70813=CARTESIAN_POINT('',(37.5088351857635,11.85,-5.07288052484118));
#70814=CARTESIAN_POINT('Origin',(39.2,11.85,-9.525));
#70815=CARTESIAN_POINT('',(37.6224320889104,12.,-5.19066778662499));
#70816=CARTESIAN_POINT('Ctrl Pts',(37.5088351857635,11.85,-5.07288052484117));
#70817=CARTESIAN_POINT('Ctrl Pts',(37.5665424125622,11.9264281650904,-5.13271645382743));
#70818=CARTESIAN_POINT('Ctrl Pts',(37.6224320889104,12.,-5.19066778662499));
#70819=CARTESIAN_POINT('',(37.633740172868,11.85,-5.02741882742375));
#70820=CARTESIAN_POINT('Ctrl Pts',(37.6224320889104,12.,-5.19066778662499));
#70821=CARTESIAN_POINT('Ctrl Pts',(37.6279956662175,11.9264281650906,-5.11034929869827));
#70822=CARTESIAN_POINT('Ctrl Pts',(37.633740172868,11.85,-5.02741882742374));
#70823=CARTESIAN_POINT('',(38.3076302129352,11.85,-4.84685053540035));
#70824=CARTESIAN_POINT('Origin',(39.2,11.85,-9.525));
#70825=CARTESIAN_POINT('',(38.3990477805113,12.,-4.98257423923119));
#70826=CARTESIAN_POINT('Ctrl Pts',(38.3076302129352,11.85,-4.84685053540035));
#70827=CARTESIAN_POINT('Ctrl Pts',(38.354070337264,11.9264281650904,-4.91579817694654));
#70828=CARTESIAN_POINT('Ctrl Pts',(38.3990477805113,12.,-4.98257423923119));
#70829=CARTESIAN_POINT('',(38.4385319535358,11.85,-4.82376902671077));
#70830=CARTESIAN_POINT('Ctrl Pts',(38.3990477805113,12.,-4.98257423923119));
#70831=CARTESIAN_POINT('Ctrl Pts',(38.4184739936393,11.9264281650905,-4.90444207467138));
#70832=CARTESIAN_POINT('Ctrl Pts',(38.4385319535358,11.85,-4.82376902671077));
#70833=CARTESIAN_POINT('',(39.133539444526,11.85,-4.76296375018353));
#70834=CARTESIAN_POINT('Origin',(39.2,11.85,-9.525));
#70835=CARTESIAN_POINT('',(39.2,12.,-4.9125));
#70836=CARTESIAN_POINT('Ctrl Pts',(39.133539444526,11.85,-4.76296375018353));
#70837=CARTESIAN_POINT('Ctrl Pts',(39.1673014067068,11.9264281650904,-4.83892816509036));
#70838=CARTESIAN_POINT('Ctrl Pts',(39.2,12.,-4.9125));
#70839=CARTESIAN_POINT('',(39.266460555474,11.85,-4.76296375018353));
#70840=CARTESIAN_POINT('Ctrl Pts',(39.2,12.,-4.9125));
#70841=CARTESIAN_POINT('Ctrl Pts',(39.2326985932933,11.9264281650901,-4.83892816509014));
#70842=CARTESIAN_POINT('Ctrl Pts',(39.266460555474,11.85,-4.76296375018353));
#70843=CARTESIAN_POINT('',(39.9614680464642,11.85,-4.82376902671077));
#70844=CARTESIAN_POINT('Origin',(39.2,11.85,-9.525));
#70845=CARTESIAN_POINT('',(40.0009522194887,12.,-4.98257423923119));
#70846=CARTESIAN_POINT('Ctrl Pts',(39.9614680464642,11.85,-4.82376902671077));
#70847=CARTESIAN_POINT('Ctrl Pts',(39.9815260063607,11.9264281650903,-4.90444207467118));
#70848=CARTESIAN_POINT('Ctrl Pts',(40.0009522194887,12.,-4.98257423923119));
#70849=CARTESIAN_POINT('',(40.0923697870648,11.85,-4.84685053540035));
#70850=CARTESIAN_POINT('Ctrl Pts',(40.0009522194887,12.,-4.98257423923119));
#70851=CARTESIAN_POINT('Ctrl Pts',(40.0459296627363,11.92642816509,-4.91579817694619));
#70852=CARTESIAN_POINT('Ctrl Pts',(40.0923697870648,11.85,-4.84685053540035));
#70853=CARTESIAN_POINT('',(40.766259827132,11.85,-5.02741882742375));
#70854=CARTESIAN_POINT('Origin',(39.2,11.85,-9.525));
#70855=CARTESIAN_POINT('',(40.7775679110897,12.,-5.190667786625));
#70856=CARTESIAN_POINT('Ctrl Pts',(40.766259827132,11.85,-5.02741882742374));
#70857=CARTESIAN_POINT('Ctrl Pts',(40.7720043337825,11.9264281650901,-5.11034929869772));
#70858=CARTESIAN_POINT('Ctrl Pts',(40.7775679110897,12.,-5.190667786625));
#70859=CARTESIAN_POINT('',(40.8911648142365,11.85,-5.07288052484118));
#70860=CARTESIAN_POINT('Ctrl Pts',(40.7775679110897,12.,-5.190667786625));
#70861=CARTESIAN_POINT('Ctrl Pts',(40.8334575874378,11.9264281650904,-5.13271645382747));
#70862=CARTESIAN_POINT('Ctrl Pts',(40.8911648142365,11.85,-5.07288052484118));
#70863=CARTESIAN_POINT('',(41.5234615955181,11.85,-5.36772535617957));
#70864=CARTESIAN_POINT('Origin',(39.2,11.85,-9.525));
#70865=CARTESIAN_POINT('',(41.50625,12.,-5.53045782504427));
#70866=CARTESIAN_POINT('Ctrl Pts',(41.5234615955181,11.85,-5.36772535617957));
#70867=CARTESIAN_POINT('Ctrl Pts',(41.5147181049949,11.9264281650903,-5.45039345036284));
#70868=CARTESIAN_POINT('Ctrl Pts',(41.50625,12.,-5.53045782504428));
#70869=CARTESIAN_POINT('',(41.6385746542983,11.85,-5.43418591165355));
#70870=CARTESIAN_POINT('Ctrl Pts',(41.50625,12.,-5.53045782504427));
#70871=CARTESIAN_POINT('Ctrl Pts',(41.5713537299146,11.9264281650904,-5.48309204365614));
#70872=CARTESIAN_POINT('Ctrl Pts',(41.6385746542983,11.85,-5.43418591165355));
#70873=CARTESIAN_POINT('',(42.2100661590527,11.85,-5.83434857130539));
#70874=CARTESIAN_POINT('Origin',(39.2,11.85,-9.525));
#70875=CARTESIAN_POINT('',(42.1648578496792,12.,-5.99162000611371));
#70876=CARTESIAN_POINT('Ctrl Pts',(42.2100661590527,11.85,-5.83434857130539));
#70877=CARTESIAN_POINT('Ctrl Pts',(42.1871003378909,11.9264281650905,-5.91424246018825));
#70878=CARTESIAN_POINT('Ctrl Pts',(42.1648578496792,12.,-5.99162000611371));
#70879=CARTESIAN_POINT('',(42.3118896374676,11.85,-5.91978861448852));
#70880=CARTESIAN_POINT('Ctrl Pts',(42.1648578496792,12.,-5.99162000611371));
#70881=CARTESIAN_POINT('Ctrl Pts',(42.2371974892713,11.9264281650901,-5.956278961434));
#70882=CARTESIAN_POINT('Ctrl Pts',(42.3118896374676,11.85,-5.91978861448852));
#70883=CARTESIAN_POINT('',(42.8052113855115,11.85,-6.41311036253237));
#70884=CARTESIAN_POINT('Origin',(39.2,11.85,-9.525));
#70885=CARTESIAN_POINT('',(42.7333799938863,12.,-6.56014215032084));
#70886=CARTESIAN_POINT('Ctrl Pts',(42.8052113855115,11.85,-6.41311036253237));
#70887=CARTESIAN_POINT('Ctrl Pts',(42.7687210385659,11.9264281650903,-6.48780251072892));
#70888=CARTESIAN_POINT('Ctrl Pts',(42.7333799938863,12.,-6.56014215032084));
#70889=CARTESIAN_POINT('',(42.8906514286946,11.85,-6.51493384094727));
#70890=CARTESIAN_POINT('Ctrl Pts',(42.7333799938863,12.,-6.56014215032084));
#70891=CARTESIAN_POINT('Ctrl Pts',(42.8107575398122,11.9264281650901,-6.53789966210898));
#70892=CARTESIAN_POINT('Ctrl Pts',(42.8906514286946,11.85,-6.51493384094727));
#70893=CARTESIAN_POINT('',(43.2908140883465,11.85,-7.08642534570167));
#70894=CARTESIAN_POINT('Origin',(39.2,11.85,-9.525));
#70895=CARTESIAN_POINT('',(43.1945421749557,12.,-7.21875000000001));
#70896=CARTESIAN_POINT('Ctrl Pts',(43.2908140883465,11.85,-7.08642534570168));
#70897=CARTESIAN_POINT('Ctrl Pts',(43.2419079563444,11.9264281650897,-7.15364627008465));
#70898=CARTESIAN_POINT('Ctrl Pts',(43.1945421749557,12.,-7.21875000000001));
#70899=CARTESIAN_POINT('',(43.3572746438204,11.85,-7.20153840448187));
#70900=CARTESIAN_POINT('Ctrl Pts',(43.1945421749557,12.,-7.21875000000001));
#70901=CARTESIAN_POINT('Ctrl Pts',(43.2746065496371,11.9264281650904,-7.21028189500509));
#70902=CARTESIAN_POINT('Ctrl Pts',(43.3572746438204,11.85,-7.20153840448187));
#70903=CARTESIAN_POINT('',(43.6521194751588,11.85,-7.83383518576351));
#70904=CARTESIAN_POINT('Origin',(39.2,11.85,-9.525));
#70905=CARTESIAN_POINT('',(43.534332213375,12.,-7.94743208891035));
#70906=CARTESIAN_POINT('Ctrl Pts',(43.6521194751588,11.85,-7.83383518576351));
#70907=CARTESIAN_POINT('Ctrl Pts',(43.5922835461722,11.9264281650908,-7.89154241256252));
#70908=CARTESIAN_POINT('Ctrl Pts',(43.534332213375,12.,-7.94743208891035));
#70909=CARTESIAN_POINT('',(43.6975811725762,11.85,-7.95874017286797));
#70910=CARTESIAN_POINT('Ctrl Pts',(43.534332213375,12.,-7.94743208891035));
#70911=CARTESIAN_POINT('Ctrl Pts',(43.614650701302,11.9264281650903,-7.9529956662175));
#70912=CARTESIAN_POINT('Ctrl Pts',(43.6975811725763,11.85,-7.95874017286797));
#70913=CARTESIAN_POINT('',(43.8781494645997,11.85,-8.63263021293523));
#70914=CARTESIAN_POINT('Origin',(39.2,11.85,-9.525));
#70915=CARTESIAN_POINT('',(43.7424257607688,12.,-8.72404778051128));
#70916=CARTESIAN_POINT('Ctrl Pts',(43.8781494645997,11.85,-8.63263021293523));
#70917=CARTESIAN_POINT('Ctrl Pts',(43.8092018230542,11.9264281650896,-8.67907033726344));
#70918=CARTESIAN_POINT('Ctrl Pts',(43.7424257607688,12.,-8.72404778051128));
#70919=CARTESIAN_POINT('',(43.9012309732892,11.85,-8.76353195353579));
#70920=CARTESIAN_POINT('Ctrl Pts',(43.7424257607688,12.,-8.72404778051128));
#70921=CARTESIAN_POINT('Ctrl Pts',(43.8205579253292,11.92642816509,-8.74347399363942));
#70922=CARTESIAN_POINT('Ctrl Pts',(43.9012309732892,11.85,-8.76353195353579));
#70923=CARTESIAN_POINT('',(43.9620362498165,11.85,-9.45853944452601));
#70924=CARTESIAN_POINT('Origin',(39.2,11.85,-9.525));
#70925=CARTESIAN_POINT('',(43.8125,12.,-9.525));
#70926=CARTESIAN_POINT('Ctrl Pts',(43.9620362498165,11.85,-9.45853944452602));
#70927=CARTESIAN_POINT('Ctrl Pts',(43.8860718349096,11.9264281650904,-9.49230140670684));
#70928=CARTESIAN_POINT('Ctrl Pts',(43.8125,12.,-9.525));
#70929=CARTESIAN_POINT('',(43.9620362498165,11.85,-9.59146055547398));
#70930=CARTESIAN_POINT('Ctrl Pts',(43.8125,12.,-9.525));
#70931=CARTESIAN_POINT('Ctrl Pts',(43.8860718349093,11.9264281650907,-9.55769859329303));
#70932=CARTESIAN_POINT('Ctrl Pts',(43.9620362498165,11.85,-9.59146055547398));
#70933=CARTESIAN_POINT('Origin',(39.2,11.85,-9.525));
#70934=CARTESIAN_POINT('',(43.6975811725762,11.85,-11.091259827132));
#70935=CARTESIAN_POINT('Origin',(39.2,11.85,-9.525));
#70936=CARTESIAN_POINT('',(43.534332213375,12.,-11.1025679110897));
#70937=CARTESIAN_POINT('Ctrl Pts',(43.6975811725763,11.85,-11.091259827132));
#70938=CARTESIAN_POINT('Ctrl Pts',(43.6146507013022,11.9264281650902,-11.0970043337825));
#70939=CARTESIAN_POINT('Ctrl Pts',(43.534332213375,12.,-11.1025679110897));
#70940=CARTESIAN_POINT('',(43.6521194751588,11.85,-11.2161648142365));
#70941=CARTESIAN_POINT('Ctrl Pts',(43.534332213375,12.,-11.1025679110897));
#70942=CARTESIAN_POINT('Ctrl Pts',(43.5922835461725,11.9264281650904,-11.1584575874378));
#70943=CARTESIAN_POINT('Ctrl Pts',(43.6521194751588,11.85,-11.2161648142365));
#70944=CARTESIAN_POINT('',(43.3572746438204,11.85,-11.8484615955181));
#70945=CARTESIAN_POINT('Origin',(39.2,11.85,-9.525));
#70946=CARTESIAN_POINT('',(43.1945421749557,12.,-11.83125));
#70947=CARTESIAN_POINT('Ctrl Pts',(43.3572746438204,11.85,-11.8484615955181));
#70948=CARTESIAN_POINT('Ctrl Pts',(43.274606549637,11.9264281650904,-11.8397181049949));
#70949=CARTESIAN_POINT('Ctrl Pts',(43.1945421749557,12.,-11.83125));
#70950=CARTESIAN_POINT('',(43.2908140883465,11.85,-11.9635746542983));
#70951=CARTESIAN_POINT('Ctrl Pts',(43.1945421749557,12.,-11.83125));
#70952=CARTESIAN_POINT('Ctrl Pts',(43.2419079563437,11.9264281650907,-11.8963537299144));
#70953=CARTESIAN_POINT('Ctrl Pts',(43.2908140883465,11.85,-11.9635746542984));
#70954=CARTESIAN_POINT('',(42.8906514286946,11.85,-12.5350661590527));
#70955=CARTESIAN_POINT('Origin',(39.2,11.85,-9.525));
#70956=CARTESIAN_POINT('',(42.7333799938863,12.,-12.4898578496792));
#70957=CARTESIAN_POINT('Ctrl Pts',(42.8906514286946,11.85,-12.5350661590527));
#70958=CARTESIAN_POINT('Ctrl Pts',(42.8107575398114,11.9264281650908,-12.5121003378908));
#70959=CARTESIAN_POINT('Ctrl Pts',(42.7333799938863,12.,-12.4898578496792));
#70960=CARTESIAN_POINT('',(42.8052113855115,11.85,-12.6368896374676));
#70961=CARTESIAN_POINT('Ctrl Pts',(42.7333799938863,12.,-12.4898578496792));
#70962=CARTESIAN_POINT('Ctrl Pts',(42.7687210385655,11.9264281650911,-12.5621974892703));
#70963=CARTESIAN_POINT('Ctrl Pts',(42.8052113855115,11.85,-12.6368896374676));
#70964=CARTESIAN_POINT('',(42.3118896374676,11.85,-13.1302113855115));
#70965=CARTESIAN_POINT('Origin',(39.2,11.85,-9.525));
#70966=CARTESIAN_POINT('',(42.1648578496792,12.,-13.0583799938863));
#70967=CARTESIAN_POINT('Ctrl Pts',(42.3118896374676,11.85,-13.1302113855115));
#70968=CARTESIAN_POINT('Ctrl Pts',(42.2371974892713,11.9264281650901,-13.093721038566));
#70969=CARTESIAN_POINT('Ctrl Pts',(42.1648578496792,12.,-13.0583799938863));
#70970=CARTESIAN_POINT('',(42.2100661590527,11.85,-13.2156514286946));
#70971=CARTESIAN_POINT('Ctrl Pts',(42.1648578496792,12.,-13.0583799938863));
#70972=CARTESIAN_POINT('Ctrl Pts',(42.1871003378909,11.9264281650906,-13.1357575398117));
#70973=CARTESIAN_POINT('Ctrl Pts',(42.2100661590527,11.85,-13.2156514286946));
#70974=CARTESIAN_POINT('',(41.6385746542983,11.85,-13.6158140883464));
#70975=CARTESIAN_POINT('Origin',(39.2,11.85,-9.525));
#70976=CARTESIAN_POINT('',(41.50625,12.,-13.5195421749557));
#70977=CARTESIAN_POINT('Ctrl Pts',(41.6385746542983,11.85,-13.6158140883465));
#70978=CARTESIAN_POINT('Ctrl Pts',(41.5713537299148,11.9264281650902,-13.566907956344));
#70979=CARTESIAN_POINT('Ctrl Pts',(41.50625,12.,-13.5195421749557));
#70980=CARTESIAN_POINT('',(41.5234615955181,11.85,-13.6822746438204));
#70981=CARTESIAN_POINT('Ctrl Pts',(41.50625,12.,-13.5195421749557));
#70982=CARTESIAN_POINT('Ctrl Pts',(41.5147181049949,11.9264281650903,-13.5996065496372));
#70983=CARTESIAN_POINT('Ctrl Pts',(41.5234615955181,11.85,-13.6822746438204));
#70984=CARTESIAN_POINT('',(40.8911648142365,11.85,-13.9771194751588));
#70985=CARTESIAN_POINT('Origin',(39.2,11.85,-9.525));
#70986=CARTESIAN_POINT('',(40.7775679110896,12.,-13.859332213375));
#70987=CARTESIAN_POINT('Ctrl Pts',(40.8911648142365,11.85,-13.9771194751588));
#70988=CARTESIAN_POINT('Ctrl Pts',(40.8334575874381,11.92642816509,-13.9172835461729));
#70989=CARTESIAN_POINT('Ctrl Pts',(40.7775679110896,12.,-13.859332213375));
#70990=CARTESIAN_POINT('',(40.766259827132,11.85,-14.0225811725762));
#70991=CARTESIAN_POINT('Ctrl Pts',(40.7775679110896,12.,-13.859332213375));
#70992=CARTESIAN_POINT('Ctrl Pts',(40.7720043337825,11.9264281650902,-13.9396507013022));
#70993=CARTESIAN_POINT('Ctrl Pts',(40.766259827132,11.85,-14.0225811725763));
#70994=CARTESIAN_POINT('',(40.0923697870648,11.85,-14.2031494645996));
#70995=CARTESIAN_POINT('Origin',(39.2,11.85,-9.525));
#70996=CARTESIAN_POINT('',(40.0009522194887,12.,-14.0674257607688));
#70997=CARTESIAN_POINT('Ctrl Pts',(40.0923697870648,11.85,-14.2031494645997));
#70998=CARTESIAN_POINT('Ctrl Pts',(40.0459296627363,11.92642816509,-14.1342018230539));
#70999=CARTESIAN_POINT('Ctrl Pts',(40.0009522194887,12.,-14.0674257607688));
#71000=CARTESIAN_POINT('',(39.9614680464642,11.85,-14.2262309732892));
#71001=CARTESIAN_POINT('Ctrl Pts',(40.0009522194887,12.,-14.0674257607688));
#71002=CARTESIAN_POINT('Ctrl Pts',(39.9815260063607,11.9264281650904,-14.1455579253287));
#71003=CARTESIAN_POINT('Ctrl Pts',(39.9614680464642,11.85,-14.2262309732892));
#71004=CARTESIAN_POINT('',(39.266460555474,11.85,-14.2870362498165));
#71005=CARTESIAN_POINT('Origin',(39.2,11.85,-9.525));
#71006=CARTESIAN_POINT('',(39.2,12.,-14.1375));
#71007=CARTESIAN_POINT('Ctrl Pts',(39.266460555474,11.85,-14.2870362498165));
#71008=CARTESIAN_POINT('Ctrl Pts',(39.2326985932933,11.9264281650901,-14.2110718349099));
#71009=CARTESIAN_POINT('Ctrl Pts',(39.2,12.,-14.1375));
#71010=CARTESIAN_POINT('',(39.133539444526,11.85,-14.2870362498165));
#71011=CARTESIAN_POINT('Ctrl Pts',(39.2,12.,-14.1375));
#71012=CARTESIAN_POINT('Ctrl Pts',(39.1673014067067,11.9264281650901,-14.2110718349099));
#71013=CARTESIAN_POINT('Ctrl Pts',(39.133539444526,11.85,-14.2870362498165));
#71014=CARTESIAN_POINT('',(38.4385319535358,11.85,-14.2262309732892));
#71015=CARTESIAN_POINT('Origin',(39.2,11.85,-9.525));
#71016=CARTESIAN_POINT('',(38.3990477805113,12.,-14.0674257607688));
#71017=CARTESIAN_POINT('Ctrl Pts',(38.4385319535358,11.85,-14.2262309732892));
#71018=CARTESIAN_POINT('Ctrl Pts',(38.4184739936393,11.9264281650903,-14.1455579253288));
#71019=CARTESIAN_POINT('Ctrl Pts',(38.3990477805113,12.,-14.0674257607688));
#71020=CARTESIAN_POINT('',(38.3076302129352,11.85,-14.2031494645996));
#71021=CARTESIAN_POINT('Ctrl Pts',(38.3990477805113,12.,-14.0674257607688));
#71022=CARTESIAN_POINT('Ctrl Pts',(38.3540703372637,11.92642816509,-14.1342018230538));
#71023=CARTESIAN_POINT('Ctrl Pts',(38.3076302129352,11.85,-14.2031494645997));
#71024=CARTESIAN_POINT('',(37.633740172868,11.85,-14.0225811725762));
#71025=CARTESIAN_POINT('Origin',(39.2,11.85,-9.525));
#71026=CARTESIAN_POINT('',(37.6224320889104,12.,-13.859332213375));
#71027=CARTESIAN_POINT('Ctrl Pts',(37.633740172868,11.85,-14.0225811725763));
#71028=CARTESIAN_POINT('Ctrl Pts',(37.6279956662175,11.9264281650903,-13.9396507013021));
#71029=CARTESIAN_POINT('Ctrl Pts',(37.6224320889104,12.,-13.859332213375));
#71030=CARTESIAN_POINT('',(37.5088351857635,11.85,-13.9771194751588));
#71031=CARTESIAN_POINT('Ctrl Pts',(37.6224320889104,12.,-13.859332213375));
#71032=CARTESIAN_POINT('Ctrl Pts',(37.566542412562,11.9264281650902,-13.9172835461727));
#71033=CARTESIAN_POINT('Ctrl Pts',(37.5088351857635,11.85,-13.9771194751588));
#71034=CARTESIAN_POINT('',(36.8765384044819,11.85,-13.6822746438204));
#71035=CARTESIAN_POINT('Origin',(39.2,11.85,-9.525));
#71036=CARTESIAN_POINT('',(36.89375,12.,-13.5195421749557));
#71037=CARTESIAN_POINT('Ctrl Pts',(36.8765384044819,11.85,-13.6822746438204));
#71038=CARTESIAN_POINT('Ctrl Pts',(36.8852818950051,11.92642816509,-13.5996065496374));
#71039=CARTESIAN_POINT('Ctrl Pts',(36.89375,12.,-13.5195421749557));
#71040=CARTESIAN_POINT('',(36.7614253457017,11.85,-13.6158140883464));
#71041=CARTESIAN_POINT('Ctrl Pts',(36.89375,12.,-13.5195421749557));
#71042=CARTESIAN_POINT('Ctrl Pts',(36.8286462700851,11.9264281650902,-13.566907956344));
#71043=CARTESIAN_POINT('Ctrl Pts',(36.7614253457017,11.85,-13.6158140883465));
#71044=CARTESIAN_POINT('',(36.1899338409473,11.85,-13.2156514286946));
#71045=CARTESIAN_POINT('Origin',(39.2,11.85,-9.525));
#71046=CARTESIAN_POINT('',(36.2351421503208,12.,-13.0583799938863));
#71047=CARTESIAN_POINT('Ctrl Pts',(36.1899338409473,11.85,-13.2156514286946));
#71048=CARTESIAN_POINT('Ctrl Pts',(36.212899662109,11.9264281650902,-13.1357575398121));
#71049=CARTESIAN_POINT('Ctrl Pts',(36.2351421503208,12.,-13.0583799938863));
#71050=CARTESIAN_POINT('',(36.0881103625324,11.85,-13.1302113855115));
#71051=CARTESIAN_POINT('Ctrl Pts',(36.2351421503208,12.,-13.0583799938863));
#71052=CARTESIAN_POINT('Ctrl Pts',(36.1628025107289,11.9264281650903,-13.0937210385659));
#71053=CARTESIAN_POINT('Ctrl Pts',(36.0881103625324,11.85,-13.1302113855115));
#71054=CARTESIAN_POINT('',(35.5947886144885,11.85,-12.6368896374676));
#71055=CARTESIAN_POINT('Origin',(39.2,11.85,-9.525));
#71056=CARTESIAN_POINT('',(35.6666200061137,12.,-12.4898578496792));
#71057=CARTESIAN_POINT('Ctrl Pts',(35.5947886144885,11.85,-12.6368896374676));
#71058=CARTESIAN_POINT('Ctrl Pts',(35.6312789614341,11.9264281650903,-12.5621974892711));
#71059=CARTESIAN_POINT('Ctrl Pts',(35.6666200061137,12.,-12.4898578496792));
#71060=CARTESIAN_POINT('',(35.5093485713054,11.85,-12.5350661590527));
#71061=CARTESIAN_POINT('Ctrl Pts',(35.6666200061137,12.,-12.4898578496792));
#71062=CARTESIAN_POINT('Ctrl Pts',(35.589242460188,11.9264281650903,-12.512100337891));
#71063=CARTESIAN_POINT('Ctrl Pts',(35.5093485713054,11.85,-12.5350661590527));
#71064=CARTESIAN_POINT('',(35.1091859116536,11.85,-11.9635746542983));
#71065=CARTESIAN_POINT('Origin',(39.2,11.85,-9.525));
#71066=CARTESIAN_POINT('',(35.2054578250443,12.,-11.83125));
#71067=CARTESIAN_POINT('Ctrl Pts',(35.1091859116536,11.85,-11.9635746542983));
#71068=CARTESIAN_POINT('Ctrl Pts',(35.158092043656,11.9264281650902,-11.8963537299149));
#71069=CARTESIAN_POINT('Ctrl Pts',(35.2054578250443,12.,-11.83125));
#71070=CARTESIAN_POINT('',(35.0427253561796,11.85,-11.8484615955181));
#71071=CARTESIAN_POINT('Ctrl Pts',(35.2054578250443,12.,-11.83125));
#71072=CARTESIAN_POINT('Ctrl Pts',(35.1253934503631,11.9264281650906,-11.8397181049949));
#71073=CARTESIAN_POINT('Ctrl Pts',(35.0427253561796,11.85,-11.8484615955181));
#71074=CARTESIAN_POINT('',(34.7478805248412,11.85,-11.2161648142365));
#71075=CARTESIAN_POINT('Origin',(39.2,11.85,-9.525));
#71076=CARTESIAN_POINT('',(34.865667786625,12.,-11.1025679110896));
#71077=CARTESIAN_POINT('Ctrl Pts',(34.7478805248412,11.85,-11.2161648142365));
#71078=CARTESIAN_POINT('Ctrl Pts',(34.8077164538272,11.92642816509,-11.1584575874381));
#71079=CARTESIAN_POINT('Ctrl Pts',(34.865667786625,12.,-11.1025679110896));
#71080=CARTESIAN_POINT('',(34.7024188274238,11.85,-11.091259827132));
#71081=CARTESIAN_POINT('Ctrl Pts',(34.865667786625,12.,-11.1025679110896));
#71082=CARTESIAN_POINT('Ctrl Pts',(34.7853492986983,11.9264281650906,-11.0970043337825));
#71083=CARTESIAN_POINT('Ctrl Pts',(34.7024188274237,11.85,-11.091259827132));
#71084=CARTESIAN_POINT('',(34.5218505354004,11.85,-10.4173697870648));
#71085=CARTESIAN_POINT('Origin',(39.2,11.85,-9.525));
#71086=CARTESIAN_POINT('',(34.6575742392312,12.,-10.3259522194887));
#71087=CARTESIAN_POINT('Ctrl Pts',(34.5218505354003,11.85,-10.4173697870648));
#71088=CARTESIAN_POINT('Ctrl Pts',(34.5907981769464,11.9264281650903,-10.3709296627361));
#71089=CARTESIAN_POINT('Ctrl Pts',(34.6575742392312,12.,-10.3259522194887));
#71090=CARTESIAN_POINT('',(34.4987690267108,11.85,-10.2864680464642));
#71091=CARTESIAN_POINT('Ctrl Pts',(34.6575742392312,12.,-10.3259522194887));
#71092=CARTESIAN_POINT('Ctrl Pts',(34.5794420746714,11.9264281650906,-10.3065260063607));
#71093=CARTESIAN_POINT('Ctrl Pts',(34.4987690267108,11.85,-10.2864680464642));
#71094=CARTESIAN_POINT('',(34.4379637501835,11.85,-9.59146055547398));
#71095=CARTESIAN_POINT('Origin',(39.2,11.85,-9.525));
#71096=CARTESIAN_POINT('Ctrl Pts',(34.4379637501835,11.85,-9.59146055547399));
#71097=CARTESIAN_POINT('Ctrl Pts',(34.5139281650899,11.9264281650899,-9.55769859329336));
#71098=CARTESIAN_POINT('Ctrl Pts',(34.5875,12.,-9.525));
#71099=CARTESIAN_POINT('',(34.8375,12.25,-9.525));
#71100=CARTESIAN_POINT('',(34.6375,12.05,-9.525));
#71101=CARTESIAN_POINT('Origin',(39.2,12.25,-9.525));
#71102=CARTESIAN_POINT('Origin',(44.0255979213938,12.25,-11.068538451429));
#71103=CARTESIAN_POINT('',(43.6975811725762,6.5,-11.091259827132));
#71104=CARTESIAN_POINT('',(43.6975811725762,5.9,-11.091259827132));
#71105=CARTESIAN_POINT('',(43.534332213375,6.5,-11.1025679110896));
#71106=CARTESIAN_POINT('',(44.0255979213938,6.5,-11.068538451429));
#71107=CARTESIAN_POINT('',(43.534332213375,12.25,-11.1025679110896));
#71108=CARTESIAN_POINT('Origin',(43.534332213375,12.25,-11.1025679110896));
#71109=CARTESIAN_POINT('',(43.6521194751588,6.5,-11.2161648142365));
#71110=CARTESIAN_POINT('',(43.6521194751588,5.9,-11.2161648142365));
#71111=CARTESIAN_POINT('',(43.534332213375,6.5,-11.1025679110896));
#71112=CARTESIAN_POINT('Origin',(43.7457630530518,6.5,-11.1795224433379));
#71113=CARTESIAN_POINT('Origin',(39.2,6.5,-9.525));
#71114=CARTESIAN_POINT('Origin',(43.6842536066587,12.25,-11.8830449192431));
#71115=CARTESIAN_POINT('',(43.3572746438204,6.5,-11.8484615955181));
#71116=CARTESIAN_POINT('',(43.3572746438204,5.9,-11.8484615955181));
#71117=CARTESIAN_POINT('',(43.1945421749557,6.5,-11.83125));
#71118=CARTESIAN_POINT('',(43.6842536066587,6.5,-11.8830449192431));
#71119=CARTESIAN_POINT('',(43.1945421749557,12.25,-11.83125));
#71120=CARTESIAN_POINT('Origin',(43.1945421749557,12.25,-11.83125));
#71121=CARTESIAN_POINT('',(43.2908140883465,6.5,-11.9635746542983));
#71122=CARTESIAN_POINT('',(43.2908140883465,5.9,-11.9635746542983));
#71123=CARTESIAN_POINT('',(43.1945421749557,6.5,-11.83125));
#71124=CARTESIAN_POINT('Origin',(43.3893978908072,6.5,-11.94375));
#71125=CARTESIAN_POINT('Origin',(39.2,6.5,-9.525));
#71126=CARTESIAN_POINT('Origin',(43.2066575152271,12.25,-12.6259033854143));
#71127=CARTESIAN_POINT('',(42.8906514286946,6.5,-12.5350661590527));
#71128=CARTESIAN_POINT('',(42.8906514286946,5.9,-12.5350661590527));
#71129=CARTESIAN_POINT('',(42.7333799938863,6.5,-12.4898578496792));
#71130=CARTESIAN_POINT('',(43.2066575152271,6.5,-12.6259033854143));
#71131=CARTESIAN_POINT('',(42.7333799938863,12.25,-12.4898578496792));
#71132=CARTESIAN_POINT('Origin',(42.7333799938863,12.25,-12.4898578496792));
#71133=CARTESIAN_POINT('',(42.8052113855115,6.5,-12.6368896374676));
#71134=CARTESIAN_POINT('',(42.8052113855115,5.9,-12.6368896374676));
#71135=CARTESIAN_POINT('',(42.7333799938863,6.5,-12.4898578496792));
#71136=CARTESIAN_POINT('Origin',(42.9057399935881,6.5,-12.6344850618586));
#71137=CARTESIAN_POINT('Origin',(39.2,6.5,-9.525));
#71138=CARTESIAN_POINT('Origin',(42.6073211626619,12.25,-13.2745424713525));
#71139=CARTESIAN_POINT('',(42.3118896374676,6.5,-13.1302113855115));
#71140=CARTESIAN_POINT('',(42.3118896374676,5.9,-13.1302113855115));
#71141=CARTESIAN_POINT('',(42.1648578496792,6.5,-13.0583799938863));
#71142=CARTESIAN_POINT('',(42.6073211626619,6.5,-13.2745424713525));
#71143=CARTESIAN_POINT('',(42.1648578496792,12.25,-13.0583799938863));
#71144=CARTESIAN_POINT('Origin',(42.1648578496792,12.25,-13.0583799938863));
#71145=CARTESIAN_POINT('',(42.2100661590527,6.5,-13.2156514286946));
#71146=CARTESIAN_POINT('',(42.2100661590527,5.9,-13.2156514286946));
#71147=CARTESIAN_POINT('',(42.1648578496792,6.5,-13.0583799938863));
#71148=CARTESIAN_POINT('Origin',(42.3094850618586,6.5,-13.2307399935881));
#71149=CARTESIAN_POINT('Origin',(39.2,6.5,-9.525));
#71150=CARTESIAN_POINT('Origin',(41.9044550807569,12.25,-13.8092536066587));
#71151=CARTESIAN_POINT('',(41.6385746542983,6.5,-13.6158140883464));
#71152=CARTESIAN_POINT('',(41.6385746542983,5.9,-13.6158140883464));
#71153=CARTESIAN_POINT('',(41.50625,6.5,-13.5195421749557));
#71154=CARTESIAN_POINT('',(41.9044550807569,6.5,-13.8092536066587));
#71155=CARTESIAN_POINT('',(41.50625,12.25,-13.5195421749557));
#71156=CARTESIAN_POINT('Origin',(41.50625,12.25,-13.5195421749557));
#71157=CARTESIAN_POINT('',(41.5234615955181,6.5,-13.6822746438204));
#71158=CARTESIAN_POINT('',(41.5234615955181,5.9,-13.6822746438204));
#71159=CARTESIAN_POINT('',(41.50625,6.5,-13.5195421749557));
#71160=CARTESIAN_POINT('Origin',(41.61875,6.5,-13.7143978908072));
#71161=CARTESIAN_POINT('Origin',(39.2,6.5,-9.525));
#71162=CARTESIAN_POINT('Origin',(41.1194154997434,12.25,-14.2137898640635));
#71163=CARTESIAN_POINT('',(40.8911648142365,6.5,-13.9771194751588));
#71164=CARTESIAN_POINT('',(40.8911648142365,5.9,-13.9771194751588));
#71165=CARTESIAN_POINT('',(40.7775679110896,6.5,-13.859332213375));
#71166=CARTESIAN_POINT('',(41.1194154997434,6.5,-14.2137898640635));
#71167=CARTESIAN_POINT('',(40.7775679110896,12.25,-13.859332213375));
#71168=CARTESIAN_POINT('Origin',(40.7775679110896,12.25,-13.859332213375));
#71169=CARTESIAN_POINT('',(40.766259827132,6.5,-14.0225811725762));
#71170=CARTESIAN_POINT('',(40.766259827132,5.9,-14.0225811725762));
#71171=CARTESIAN_POINT('',(40.7775679110896,6.5,-13.859332213375));
#71172=CARTESIAN_POINT('Origin',(40.8545224433379,6.5,-14.0707630530518));
#71173=CARTESIAN_POINT('Origin',(39.2,6.5,-9.525));
#71174=CARTESIAN_POINT('Origin',(40.2760554500413,12.25,-14.4758596140909));
#71175=CARTESIAN_POINT('',(40.0923697870648,6.5,-14.2031494645996));
#71176=CARTESIAN_POINT('',(40.0923697870648,5.9,-14.2031494645996));
#71177=CARTESIAN_POINT('',(40.0009522194887,6.5,-14.0674257607688));
#71178=CARTESIAN_POINT('',(40.2760554500413,6.5,-14.4758596140909));
#71179=CARTESIAN_POINT('',(40.0009522194887,12.25,-14.0674257607688));
#71180=CARTESIAN_POINT('Origin',(40.0009522194887,12.25,-14.0674257607688));
#71181=CARTESIAN_POINT('',(39.9614680464642,6.5,-14.2262309732892));
#71182=CARTESIAN_POINT('',(39.9614680464642,5.9,-14.2262309732892));
#71183=CARTESIAN_POINT('',(40.0009522194887,6.5,-14.0674257607688));
#71184=CARTESIAN_POINT('Origin',(40.0400230594638,6.5,-14.2890075051966));
#71185=CARTESIAN_POINT('Origin',(39.2,6.5,-9.525));
#71186=CARTESIAN_POINT('Origin',(39.4,12.25,-14.5875));
#71187=CARTESIAN_POINT('',(39.266460555474,6.5,-14.2870362498165));
#71188=CARTESIAN_POINT('',(39.266460555474,5.9,-14.2870362498165));
#71189=CARTESIAN_POINT('',(39.2,6.5,-14.1375));
#71190=CARTESIAN_POINT('',(39.4,6.5,-14.5875));
#71191=CARTESIAN_POINT('',(39.2,12.25,-14.1375));
#71192=CARTESIAN_POINT('Origin',(39.2,12.25,-14.1375));
#71193=CARTESIAN_POINT('',(39.133539444526,6.5,-14.2870362498165));
#71194=CARTESIAN_POINT('',(39.133539444526,5.9,-14.2870362498165));
#71195=CARTESIAN_POINT('',(39.2,6.5,-14.1375));
#71196=CARTESIAN_POINT('Origin',(39.2,6.5,-14.3625));
#71197=CARTESIAN_POINT('Origin',(39.2,6.5,-9.525));
#71198=CARTESIAN_POINT('Origin',(38.5178676511636,12.25,-14.5453188851577));
#71199=CARTESIAN_POINT('',(38.4385319535358,6.5,-14.2262309732892));
#71200=CARTESIAN_POINT('',(38.4385319535358,5.9,-14.2262309732892));
#71201=CARTESIAN_POINT('',(38.3990477805113,6.5,-14.0674257607688));
#71202=CARTESIAN_POINT('',(38.5178676511636,6.5,-14.5453188851577));
#71203=CARTESIAN_POINT('',(38.3990477805113,12.25,-14.0674257607688));
#71204=CARTESIAN_POINT('Origin',(38.3990477805113,12.25,-14.0674257607688));
#71205=CARTESIAN_POINT('',(38.3076302129352,6.5,-14.2031494645996));
#71206=CARTESIAN_POINT('',(38.3076302129352,5.9,-14.2031494645996));
#71207=CARTESIAN_POINT('',(38.3990477805113,6.5,-14.0674257607688));
#71208=CARTESIAN_POINT('Origin',(38.3599769405362,6.5,-14.2890075051966));
#71209=CARTESIAN_POINT('Origin',(39.2,6.5,-9.525));
#71210=CARTESIAN_POINT('Origin',(37.656461548571,12.25,-14.3505979213938));
#71211=CARTESIAN_POINT('',(37.633740172868,6.5,-14.0225811725762));
#71212=CARTESIAN_POINT('',(37.633740172868,5.9,-14.0225811725762));
#71213=CARTESIAN_POINT('',(37.6224320889104,6.5,-13.859332213375));
#71214=CARTESIAN_POINT('',(37.656461548571,6.5,-14.3505979213938));
#71215=CARTESIAN_POINT('',(37.6224320889104,12.25,-13.859332213375));
#71216=CARTESIAN_POINT('Origin',(37.6224320889104,12.25,-13.859332213375));
#71217=CARTESIAN_POINT('',(37.5088351857635,6.5,-13.9771194751588));
#71218=CARTESIAN_POINT('',(37.5088351857635,5.9,-13.9771194751588));
#71219=CARTESIAN_POINT('',(37.6224320889104,6.5,-13.859332213375));
#71220=CARTESIAN_POINT('Origin',(37.5454775566621,6.5,-14.0707630530518));
#71221=CARTESIAN_POINT('Origin',(39.2,6.5,-9.525));
#71222=CARTESIAN_POINT('Origin',(36.8419550807569,12.25,-14.0092536066587));
#71223=CARTESIAN_POINT('',(36.8765384044819,6.5,-13.6822746438204));
#71224=CARTESIAN_POINT('',(36.8765384044819,5.9,-13.6822746438204));
#71225=CARTESIAN_POINT('',(36.89375,6.5,-13.5195421749557));
#71226=CARTESIAN_POINT('',(36.8419550807569,6.5,-14.0092536066587));
#71227=CARTESIAN_POINT('',(36.89375,12.25,-13.5195421749557));
#71228=CARTESIAN_POINT('Origin',(36.89375,12.25,-13.5195421749557));
#71229=CARTESIAN_POINT('',(36.7614253457017,6.5,-13.6158140883464));
#71230=CARTESIAN_POINT('',(36.7614253457017,5.9,-13.6158140883464));
#71231=CARTESIAN_POINT('',(36.89375,6.5,-13.5195421749557));
#71232=CARTESIAN_POINT('Origin',(36.78125,6.5,-13.7143978908072));
#71233=CARTESIAN_POINT('Origin',(39.2,6.5,-9.525));
#71234=CARTESIAN_POINT('Origin',(36.0990966145857,12.25,-13.5316575152271));
#71235=CARTESIAN_POINT('',(36.1899338409473,6.5,-13.2156514286946));
#71236=CARTESIAN_POINT('',(36.1899338409473,5.9,-13.2156514286946));
#71237=CARTESIAN_POINT('',(36.2351421503208,6.5,-13.0583799938863));
#71238=CARTESIAN_POINT('',(36.0990966145857,6.5,-13.5316575152271));
#71239=CARTESIAN_POINT('',(36.2351421503208,12.25,-13.0583799938863));
#71240=CARTESIAN_POINT('Origin',(36.2351421503208,12.25,-13.0583799938863));
#71241=CARTESIAN_POINT('',(36.0881103625324,6.5,-13.1302113855115));
#71242=CARTESIAN_POINT('',(36.0881103625324,5.9,-13.1302113855115));
#71243=CARTESIAN_POINT('',(36.2351421503208,6.5,-13.0583799938863));
#71244=CARTESIAN_POINT('Origin',(36.0905149381414,6.5,-13.2307399935881));
#71245=CARTESIAN_POINT('Origin',(39.2,6.5,-9.525));
#71246=CARTESIAN_POINT('Origin',(35.4504575286475,12.25,-12.9323211626619));
#71247=CARTESIAN_POINT('',(35.5947886144885,6.5,-12.6368896374676));
#71248=CARTESIAN_POINT('',(35.5947886144885,5.9,-12.6368896374676));
#71249=CARTESIAN_POINT('',(35.6666200061137,6.5,-12.4898578496792));
#71250=CARTESIAN_POINT('',(35.4504575286475,6.5,-12.9323211626619));
#71251=CARTESIAN_POINT('',(35.6666200061137,12.25,-12.4898578496792));
#71252=CARTESIAN_POINT('Origin',(35.6666200061137,12.25,-12.4898578496792));
#71253=CARTESIAN_POINT('',(35.5093485713054,6.5,-12.5350661590527));
#71254=CARTESIAN_POINT('',(35.5093485713054,5.9,-12.5350661590527));
#71255=CARTESIAN_POINT('',(35.6666200061137,6.5,-12.4898578496792));
#71256=CARTESIAN_POINT('Origin',(35.4942600064119,6.5,-12.6344850618586));
#71257=CARTESIAN_POINT('Origin',(39.2,6.5,-9.525));
#71258=CARTESIAN_POINT('Origin',(34.9157463933413,12.25,-12.2294550807569));
#71259=CARTESIAN_POINT('',(35.1091859116536,6.5,-11.9635746542983));
#71260=CARTESIAN_POINT('',(35.1091859116536,5.9,-11.9635746542983));
#71261=CARTESIAN_POINT('',(35.2054578250443,6.5,-11.83125));
#71262=CARTESIAN_POINT('',(34.9157463933413,6.5,-12.2294550807569));
#71263=CARTESIAN_POINT('',(35.2054578250443,12.25,-11.83125));
#71264=CARTESIAN_POINT('Origin',(35.2054578250443,12.25,-11.83125));
#71265=CARTESIAN_POINT('',(35.0427253561796,6.5,-11.8484615955181));
#71266=CARTESIAN_POINT('',(35.0427253561796,5.9,-11.8484615955181));
#71267=CARTESIAN_POINT('',(35.2054578250443,6.5,-11.83125));
#71268=CARTESIAN_POINT('Origin',(35.0106021091928,6.5,-11.94375));
#71269=CARTESIAN_POINT('Origin',(39.2,6.5,-9.525));
#71270=CARTESIAN_POINT('Origin',(34.5112101359365,12.25,-11.4444154997434));
#71271=CARTESIAN_POINT('',(34.7478805248412,6.5,-11.2161648142365));
#71272=CARTESIAN_POINT('',(34.7478805248412,5.9,-11.2161648142365));
#71273=CARTESIAN_POINT('',(34.865667786625,6.5,-11.1025679110896));
#71274=CARTESIAN_POINT('',(34.5112101359365,6.5,-11.4444154997434));
#71275=CARTESIAN_POINT('',(34.865667786625,12.25,-11.1025679110896));
#71276=CARTESIAN_POINT('Origin',(34.865667786625,12.25,-11.1025679110896));
#71277=CARTESIAN_POINT('',(34.7024188274238,6.5,-11.091259827132));
#71278=CARTESIAN_POINT('',(34.7024188274238,5.9,-11.091259827132));
#71279=CARTESIAN_POINT('',(34.865667786625,6.5,-11.1025679110896));
#71280=CARTESIAN_POINT('Origin',(34.6542369469482,6.5,-11.1795224433379));
#71281=CARTESIAN_POINT('Origin',(39.2,6.5,-9.525));
#71282=CARTESIAN_POINT('Origin',(34.2491403859091,12.25,-10.6010554500413));
#71283=CARTESIAN_POINT('',(34.5218505354004,6.5,-10.4173697870648));
#71284=CARTESIAN_POINT('',(34.5218505354004,5.9,-10.4173697870648));
#71285=CARTESIAN_POINT('',(34.6575742392312,6.5,-10.3259522194887));
#71286=CARTESIAN_POINT('',(34.2491403859091,6.5,-10.6010554500413));
#71287=CARTESIAN_POINT('',(34.6575742392312,12.25,-10.3259522194887));
#71288=CARTESIAN_POINT('Origin',(34.6575742392312,12.25,-10.3259522194887));
#71289=CARTESIAN_POINT('',(34.4987690267108,6.5,-10.2864680464642));
#71290=CARTESIAN_POINT('',(34.4987690267108,5.9,-10.2864680464642));
#71291=CARTESIAN_POINT('',(34.6575742392312,6.5,-10.3259522194887));
#71292=CARTESIAN_POINT('Origin',(34.4359924948034,6.5,-10.3650230594638));
#71293=CARTESIAN_POINT('Origin',(39.2,6.5,-9.525));
#71294=CARTESIAN_POINT('Origin',(34.1375,12.25,-9.725));
#71295=CARTESIAN_POINT('',(34.4379637501835,6.5,-9.59146055547398));
#71296=CARTESIAN_POINT('',(34.4379637501835,5.9,-9.59146055547398));
#71297=CARTESIAN_POINT('',(34.5875,6.5,-9.525));
#71298=CARTESIAN_POINT('',(34.1375,6.5,-9.725));
#71299=CARTESIAN_POINT('',(34.5875,12.25,-9.525));
#71300=CARTESIAN_POINT('Origin',(34.5875,12.25,-9.525));
#71301=CARTESIAN_POINT('',(34.4379637501835,6.5,-9.45853944452601));
#71302=CARTESIAN_POINT('',(34.4379637501835,5.9,-9.45853944452601));
#71303=CARTESIAN_POINT('',(34.5875,6.5,-9.525));
#71304=CARTESIAN_POINT('Origin',(34.3625,6.5,-9.525));
#71305=CARTESIAN_POINT('',(34.4375,6.5,-9.525));
#71306=CARTESIAN_POINT('Origin',(39.2,6.5,-9.525));
#71307=CARTESIAN_POINT('Origin',(39.2,6.5,-9.525));
#71308=CARTESIAN_POINT('Origin',(34.1796811148423,12.25,-8.84286765116361));
#71309=CARTESIAN_POINT('',(34.4987690267108,6.5,-8.76353195353579));
#71310=CARTESIAN_POINT('',(34.4987690267108,5.9,-8.76353195353579));
#71311=CARTESIAN_POINT('',(34.6575742392312,6.5,-8.72404778051128));
#71312=CARTESIAN_POINT('',(34.1796811148423,6.5,-8.84286765116361));
#71313=CARTESIAN_POINT('',(34.6575742392312,12.25,-8.72404778051128));
#71314=CARTESIAN_POINT('Origin',(34.6575742392312,12.25,-8.72404778051128));
#71315=CARTESIAN_POINT('',(34.5218505354004,6.5,-8.63263021293523));
#71316=CARTESIAN_POINT('',(34.5218505354004,5.9,-8.63263021293523));
#71317=CARTESIAN_POINT('',(34.6575742392312,6.5,-8.72404778051128));
#71318=CARTESIAN_POINT('Origin',(34.4359924948035,6.5,-8.68497694053623));
#71319=CARTESIAN_POINT('Origin',(39.2,6.5,-9.525));
#71320=CARTESIAN_POINT('Origin',(34.3744020786062,12.25,-7.98146154857098));
#71321=CARTESIAN_POINT('',(34.7024188274238,6.5,-7.95874017286797));
#71322=CARTESIAN_POINT('',(34.7024188274238,5.9,-7.95874017286797));
#71323=CARTESIAN_POINT('',(34.865667786625,6.5,-7.94743208891035));
#71324=CARTESIAN_POINT('',(34.3744020786062,6.5,-7.98146154857098));
#71325=CARTESIAN_POINT('',(34.865667786625,12.25,-7.94743208891035));
#71326=CARTESIAN_POINT('Origin',(34.865667786625,12.25,-7.94743208891035));
#71327=CARTESIAN_POINT('',(34.7478805248412,6.5,-7.8338351857635));
#71328=CARTESIAN_POINT('',(34.7478805248412,5.9,-7.8338351857635));
#71329=CARTESIAN_POINT('',(34.865667786625,6.5,-7.94743208891035));
#71330=CARTESIAN_POINT('Origin',(34.6542369469482,6.5,-7.87047755666207));
#71331=CARTESIAN_POINT('Origin',(39.2,6.5,-9.525));
#71332=CARTESIAN_POINT('Origin',(34.7157463933413,12.25,-7.16695508075689));
#71333=CARTESIAN_POINT('',(35.0427253561796,6.5,-7.20153840448186));
#71334=CARTESIAN_POINT('',(35.0427253561796,5.9,-7.20153840448186));
#71335=CARTESIAN_POINT('',(35.2054578250443,6.5,-7.21875));
#71336=CARTESIAN_POINT('',(34.7157463933413,6.5,-7.16695508075689));
#71337=CARTESIAN_POINT('',(35.2054578250443,12.25,-7.21875));
#71338=CARTESIAN_POINT('Origin',(35.2054578250443,12.25,-7.21875));
#71339=CARTESIAN_POINT('',(35.1091859116536,6.5,-7.08642534570167));
#71340=CARTESIAN_POINT('',(35.1091859116536,5.9,-7.08642534570168));
#71341=CARTESIAN_POINT('',(35.2054578250443,6.5,-7.21875));
#71342=CARTESIAN_POINT('Origin',(35.0106021091928,6.5,-7.10625));
#71343=CARTESIAN_POINT('Origin',(39.2,6.5,-9.525));
#71344=CARTESIAN_POINT('Origin',(35.1933424847729,12.25,-6.42409661458569));
#71345=CARTESIAN_POINT('',(35.5093485713054,6.5,-6.51493384094727));
#71346=CARTESIAN_POINT('',(35.5093485713054,5.9,-6.51493384094727));
#71347=CARTESIAN_POINT('',(35.6666200061137,6.5,-6.56014215032084));
#71348=CARTESIAN_POINT('',(35.1933424847729,6.5,-6.42409661458569));
#71349=CARTESIAN_POINT('',(35.6666200061137,12.25,-6.56014215032084));
#71350=CARTESIAN_POINT('Origin',(35.6666200061137,12.25,-6.56014215032084));
#71351=CARTESIAN_POINT('',(35.5947886144885,6.5,-6.41311036253237));
#71352=CARTESIAN_POINT('',(35.5947886144885,5.9,-6.41311036253237));
#71353=CARTESIAN_POINT('',(35.6666200061137,6.5,-6.56014215032084));
#71354=CARTESIAN_POINT('Origin',(35.4942600064119,6.5,-6.41551493814136));
#71355=CARTESIAN_POINT('Origin',(39.2,6.5,-9.525));
#71356=CARTESIAN_POINT('Origin',(35.7926788373381,12.25,-5.77545752864748));
#71357=CARTESIAN_POINT('',(36.0881103625324,6.5,-5.91978861448852));
#71358=CARTESIAN_POINT('',(36.0881103625324,5.9,-5.91978861448852));
#71359=CARTESIAN_POINT('',(36.2351421503208,6.5,-5.99162000611371));
#71360=CARTESIAN_POINT('',(35.7926788373381,6.5,-5.77545752864748));
#71361=CARTESIAN_POINT('',(36.2351421503208,12.25,-5.99162000611371));
#71362=CARTESIAN_POINT('Origin',(36.2351421503208,12.25,-5.99162000611371));
#71363=CARTESIAN_POINT('',(36.1899338409473,6.5,-5.83434857130539));
#71364=CARTESIAN_POINT('',(36.1899338409473,5.9,-5.83434857130539));
#71365=CARTESIAN_POINT('',(36.2351421503208,6.5,-5.99162000611371));
#71366=CARTESIAN_POINT('Origin',(36.0905149381414,6.5,-5.81926000641194));
#71367=CARTESIAN_POINT('Origin',(39.2,6.5,-9.525));
#71368=CARTESIAN_POINT('Origin',(36.4955449192431,12.25,-5.24074639334128));
#71369=CARTESIAN_POINT('',(36.7614253457017,6.5,-5.43418591165355));
#71370=CARTESIAN_POINT('',(36.7614253457017,5.9,-5.43418591165355));
#71371=CARTESIAN_POINT('',(36.89375,6.5,-5.53045782504427));
#71372=CARTESIAN_POINT('',(36.4955449192431,6.5,-5.24074639334128));
#71373=CARTESIAN_POINT('',(36.89375,12.25,-5.53045782504427));
#71374=CARTESIAN_POINT('Origin',(36.89375,12.25,-5.53045782504427));
#71375=CARTESIAN_POINT('',(36.8765384044819,6.5,-5.36772535617957));
#71376=CARTESIAN_POINT('',(36.8765384044819,5.9,-5.36772535617957));
#71377=CARTESIAN_POINT('',(36.89375,6.5,-5.53045782504427));
#71378=CARTESIAN_POINT('Origin',(36.78125,6.5,-5.33560210919277));
#71379=CARTESIAN_POINT('Origin',(39.2,6.5,-9.525));
#71380=CARTESIAN_POINT('Origin',(37.2805845002566,12.25,-4.83621013593647));
#71381=CARTESIAN_POINT('',(37.5088351857635,6.5,-5.07288052484118));
#71382=CARTESIAN_POINT('',(37.5088351857635,5.9,-5.07288052484118));
#71383=CARTESIAN_POINT('',(37.6224320889104,6.5,-5.19066778662499));
#71384=CARTESIAN_POINT('',(37.2805845002566,6.5,-4.83621013593647));
#71385=CARTESIAN_POINT('',(37.6224320889104,12.25,-5.19066778662499));
#71386=CARTESIAN_POINT('Origin',(37.6224320889104,12.25,-5.19066778662499));
#71387=CARTESIAN_POINT('',(37.633740172868,6.5,-5.02741882742375));
#71388=CARTESIAN_POINT('',(37.633740172868,5.9,-5.02741882742375));
#71389=CARTESIAN_POINT('',(37.6224320889104,6.5,-5.19066778662499));
#71390=CARTESIAN_POINT('Origin',(37.5454775566621,6.5,-4.97923694694816));
#71391=CARTESIAN_POINT('Origin',(39.2,6.5,-9.525));
#71392=CARTESIAN_POINT('Origin',(38.1239445499587,12.25,-4.57414038590907));
#71393=CARTESIAN_POINT('',(38.3076302129352,6.5,-4.84685053540035));
#71394=CARTESIAN_POINT('',(38.3076302129352,5.9,-4.84685053540035));
#71395=CARTESIAN_POINT('',(38.3990477805113,6.5,-4.98257423923119));
#71396=CARTESIAN_POINT('',(38.1239445499587,6.5,-4.57414038590907));
#71397=CARTESIAN_POINT('',(38.3990477805113,12.25,-4.98257423923119));
#71398=CARTESIAN_POINT('Origin',(38.3990477805113,12.25,-4.98257423923119));
#71399=CARTESIAN_POINT('',(38.4385319535358,6.5,-4.82376902671077));
#71400=CARTESIAN_POINT('',(38.4385319535358,5.9,-4.82376902671077));
#71401=CARTESIAN_POINT('',(38.3990477805113,6.5,-4.98257423923119));
#71402=CARTESIAN_POINT('Origin',(38.3599769405362,6.5,-4.76099249480344));
#71403=CARTESIAN_POINT('Origin',(39.2,6.5,-9.525));
#71404=CARTESIAN_POINT('Origin',(39.,12.25,-4.4625));
#71405=CARTESIAN_POINT('',(39.133539444526,6.5,-4.76296375018353));
#71406=CARTESIAN_POINT('',(39.133539444526,5.9,-4.76296375018353));
#71407=CARTESIAN_POINT('',(39.2,6.5,-4.9125));
#71408=CARTESIAN_POINT('',(39.,6.5,-4.4625));
#71409=CARTESIAN_POINT('',(39.2,12.25,-4.9125));
#71410=CARTESIAN_POINT('Origin',(39.2,12.25,-4.9125));
#71411=CARTESIAN_POINT('',(39.266460555474,6.5,-4.76296375018353));
#71412=CARTESIAN_POINT('',(39.266460555474,5.9,-4.76296375018353));
#71413=CARTESIAN_POINT('',(39.2,6.5,-4.9125));
#71414=CARTESIAN_POINT('Origin',(39.2,6.5,-4.6875));
#71415=CARTESIAN_POINT('Origin',(39.2,6.5,-9.525));
#71416=CARTESIAN_POINT('Origin',(39.8821323488364,12.25,-4.50468111484231));
#71417=CARTESIAN_POINT('',(39.9614680464642,6.5,-4.82376902671077));
#71418=CARTESIAN_POINT('',(39.9614680464642,5.9,-4.82376902671077));
#71419=CARTESIAN_POINT('',(40.0009522194887,6.5,-4.98257423923119));
#71420=CARTESIAN_POINT('',(39.8821323488364,6.5,-4.50468111484231));
#71421=CARTESIAN_POINT('',(40.0009522194887,12.25,-4.98257423923119));
#71422=CARTESIAN_POINT('Origin',(40.0009522194887,12.25,-4.98257423923119));
#71423=CARTESIAN_POINT('',(40.0923697870648,6.5,-4.84685053540035));
#71424=CARTESIAN_POINT('',(40.0923697870648,5.9,-4.84685053540035));
#71425=CARTESIAN_POINT('',(40.0009522194887,6.5,-4.98257423923119));
#71426=CARTESIAN_POINT('Origin',(40.0400230594638,6.5,-4.76099249480344));
#71427=CARTESIAN_POINT('Origin',(39.2,6.5,-9.525));
#71428=CARTESIAN_POINT('Origin',(40.743538451429,12.25,-4.69940207860621));
#71429=CARTESIAN_POINT('',(40.766259827132,6.5,-5.02741882742375));
#71430=CARTESIAN_POINT('',(40.766259827132,5.9,-5.02741882742375));
#71431=CARTESIAN_POINT('',(40.7775679110897,6.5,-5.190667786625));
#71432=CARTESIAN_POINT('',(40.743538451429,6.5,-4.69940207860621));
#71433=CARTESIAN_POINT('',(40.7775679110897,12.25,-5.190667786625));
#71434=CARTESIAN_POINT('Origin',(40.7775679110897,12.25,-5.190667786625));
#71435=CARTESIAN_POINT('',(40.8911648142365,6.5,-5.07288052484118));
#71436=CARTESIAN_POINT('',(40.8911648142365,5.9,-5.07288052484118));
#71437=CARTESIAN_POINT('',(40.7775679110897,6.5,-5.190667786625));
#71438=CARTESIAN_POINT('Origin',(40.8545224433379,6.5,-4.97923694694817));
#71439=CARTESIAN_POINT('Origin',(39.2,6.5,-9.525));
#71440=CARTESIAN_POINT('Origin',(41.5580449192431,12.25,-5.04074639334128));
#71441=CARTESIAN_POINT('',(41.5234615955181,6.5,-5.36772535617957));
#71442=CARTESIAN_POINT('',(41.5234615955181,5.9,-5.36772535617957));
#71443=CARTESIAN_POINT('',(41.50625,6.5,-5.53045782504427));
#71444=CARTESIAN_POINT('',(41.5580449192431,6.5,-5.04074639334128));
#71445=CARTESIAN_POINT('',(41.50625,12.25,-5.53045782504427));
#71446=CARTESIAN_POINT('Origin',(41.50625,12.25,-5.53045782504427));
#71447=CARTESIAN_POINT('',(41.6385746542983,6.5,-5.43418591165355));
#71448=CARTESIAN_POINT('',(41.6385746542983,5.9,-5.43418591165355));
#71449=CARTESIAN_POINT('',(41.50625,6.5,-5.53045782504427));
#71450=CARTESIAN_POINT('Origin',(41.61875,6.5,-5.33560210919277));
#71451=CARTESIAN_POINT('Origin',(39.2,6.5,-9.525));
#71452=CARTESIAN_POINT('Origin',(42.3009033854143,12.25,-5.51834248477286));
#71453=CARTESIAN_POINT('',(42.2100661590527,6.5,-5.83434857130539));
#71454=CARTESIAN_POINT('',(42.2100661590527,5.9,-5.83434857130539));
#71455=CARTESIAN_POINT('',(42.1648578496792,6.5,-5.99162000611371));
#71456=CARTESIAN_POINT('',(42.3009033854143,6.5,-5.51834248477286));
#71457=CARTESIAN_POINT('',(42.1648578496792,12.25,-5.99162000611371));
#71458=CARTESIAN_POINT('Origin',(42.1648578496792,12.25,-5.99162000611371));
#71459=CARTESIAN_POINT('',(42.3118896374676,6.5,-5.91978861448852));
#71460=CARTESIAN_POINT('',(42.3118896374676,5.9,-5.91978861448852));
#71461=CARTESIAN_POINT('',(42.1648578496792,6.5,-5.99162000611371));
#71462=CARTESIAN_POINT('Origin',(42.3094850618586,6.5,-5.81926000641194));
#71463=CARTESIAN_POINT('Origin',(39.2,6.5,-9.525));
#71464=CARTESIAN_POINT('Origin',(42.9495424713525,12.25,-6.1176788373381));
#71465=CARTESIAN_POINT('',(42.8052113855115,6.5,-6.41311036253237));
#71466=CARTESIAN_POINT('',(42.8052113855115,5.9,-6.41311036253237));
#71467=CARTESIAN_POINT('',(42.7333799938863,6.5,-6.56014215032084));
#71468=CARTESIAN_POINT('',(42.9495424713525,6.5,-6.1176788373381));
#71469=CARTESIAN_POINT('',(42.7333799938863,12.25,-6.56014215032084));
#71470=CARTESIAN_POINT('Origin',(42.7333799938863,12.25,-6.56014215032084));
#71471=CARTESIAN_POINT('',(42.8906514286946,6.5,-6.51493384094727));
#71472=CARTESIAN_POINT('',(42.8906514286946,5.9,-6.51493384094727));
#71473=CARTESIAN_POINT('',(42.7333799938863,6.5,-6.56014215032084));
#71474=CARTESIAN_POINT('Origin',(42.9057399935881,6.5,-6.41551493814136));
#71475=CARTESIAN_POINT('Origin',(39.2,6.5,-9.525));
#71476=CARTESIAN_POINT('Origin',(43.4842536066587,12.25,-6.82054491924312));
#71477=CARTESIAN_POINT('',(43.2908140883465,6.5,-7.08642534570167));
#71478=CARTESIAN_POINT('',(43.2908140883465,5.9,-7.08642534570167));
#71479=CARTESIAN_POINT('',(43.1945421749557,6.5,-7.21875));
#71480=CARTESIAN_POINT('',(43.4842536066587,6.5,-6.82054491924312));
#71481=CARTESIAN_POINT('',(43.1945421749557,12.25,-7.21875));
#71482=CARTESIAN_POINT('Origin',(43.1945421749557,12.25,-7.21875));
#71483=CARTESIAN_POINT('',(43.3572746438204,6.5,-7.20153840448187));
#71484=CARTESIAN_POINT('',(43.3572746438204,5.9,-7.20153840448187));
#71485=CARTESIAN_POINT('',(43.1945421749557,6.5,-7.21875));
#71486=CARTESIAN_POINT('Origin',(43.3893978908072,6.5,-7.10625));
#71487=CARTESIAN_POINT('Origin',(39.2,6.5,-9.525));
#71488=CARTESIAN_POINT('Origin',(43.8887898640635,12.25,-7.60558450025662));
#71489=CARTESIAN_POINT('',(43.6521194751588,6.5,-7.83383518576351));
#71490=CARTESIAN_POINT('',(43.6521194751588,5.9,-7.83383518576351));
#71491=CARTESIAN_POINT('',(43.534332213375,6.5,-7.94743208891035));
#71492=CARTESIAN_POINT('',(43.8887898640635,6.5,-7.60558450025662));
#71493=CARTESIAN_POINT('',(43.534332213375,12.25,-7.94743208891035));
#71494=CARTESIAN_POINT('Origin',(43.534332213375,12.25,-7.94743208891035));
#71495=CARTESIAN_POINT('',(43.6975811725762,6.5,-7.95874017286797));
#71496=CARTESIAN_POINT('',(43.6975811725762,5.9,-7.95874017286797));
#71497=CARTESIAN_POINT('',(43.534332213375,6.5,-7.94743208891035));
#71498=CARTESIAN_POINT('Origin',(43.7457630530518,6.5,-7.87047755666208));
#71499=CARTESIAN_POINT('Origin',(39.2,6.5,-9.525));
#71500=CARTESIAN_POINT('Origin',(44.1508596140909,12.25,-8.44894454995872));
#71501=CARTESIAN_POINT('',(43.8781494645997,6.5,-8.63263021293523));
#71502=CARTESIAN_POINT('',(43.8781494645997,5.9,-8.63263021293523));
#71503=CARTESIAN_POINT('',(43.7424257607688,6.5,-8.72404778051128));
#71504=CARTESIAN_POINT('',(44.1508596140909,6.5,-8.44894454995872));
#71505=CARTESIAN_POINT('',(43.7424257607688,12.25,-8.72404778051128));
#71506=CARTESIAN_POINT('Origin',(43.7424257607688,12.25,-8.72404778051128));
#71507=CARTESIAN_POINT('',(43.9012309732892,6.5,-8.76353195353578));
#71508=CARTESIAN_POINT('',(43.9012309732892,5.9,-8.76353195353579));
#71509=CARTESIAN_POINT('',(43.7424257607688,6.5,-8.72404778051128));
#71510=CARTESIAN_POINT('Origin',(43.9640075051965,6.5,-8.68497694053622));
#71511=CARTESIAN_POINT('Origin',(39.2,6.5,-9.525));
#71512=CARTESIAN_POINT('Origin',(44.2625,12.25,-9.325));
#71513=CARTESIAN_POINT('',(43.9620362498165,6.5,-9.45853944452601));
#71514=CARTESIAN_POINT('',(43.9620362498165,5.9,-9.45853944452601));
#71515=CARTESIAN_POINT('',(43.8125,6.5,-9.525));
#71516=CARTESIAN_POINT('',(44.2625,6.5,-9.325));
#71517=CARTESIAN_POINT('',(43.8125,12.25,-9.525));
#71518=CARTESIAN_POINT('Origin',(43.8125,12.25,-9.525));
#71519=CARTESIAN_POINT('',(43.9620362498165,6.5,-9.59146055547398));
#71520=CARTESIAN_POINT('',(43.9620362498165,5.9,-9.59146055547398));
#71521=CARTESIAN_POINT('',(43.8125,6.5,-9.525));
#71522=CARTESIAN_POINT('Origin',(44.0375,6.5,-9.525));
#71523=CARTESIAN_POINT('Origin',(39.2,6.5,-9.525));
#71524=CARTESIAN_POINT('Origin',(39.2,5.9,-9.525));
#71525=CARTESIAN_POINT('',(34.4375,5.9,-9.525));
#71526=CARTESIAN_POINT('Origin',(39.2,12.25,-9.525));
#71527=CARTESIAN_POINT('',(36.4503693429844,12.25,-9.525));
#71528=CARTESIAN_POINT('',(37.8251846714922,12.25,-11.90625));
#71529=CARTESIAN_POINT('',(36.7940731751114,12.25,-10.1203125));
#71530=CARTESIAN_POINT('',(40.5748153285078,12.25,-11.90625));
#71531=CARTESIAN_POINT('',(38.5125923357461,12.25,-11.90625));
#71532=CARTESIAN_POINT('',(41.9496306570156,12.25,-9.525));
#71533=CARTESIAN_POINT('',(40.9185191606347,12.25,-11.3109375));
#71534=CARTESIAN_POINT('',(40.5748153285078,12.25,-7.14375));
#71535=CARTESIAN_POINT('',(41.6059268248886,12.25,-8.9296875));
#71536=CARTESIAN_POINT('',(37.8251846714922,12.25,-7.14375));
#71537=CARTESIAN_POINT('',(39.8874076642539,12.25,-7.14375));
#71538=CARTESIAN_POINT('',(37.4814808393653,12.25,-7.7390625));
#71539=CARTESIAN_POINT('Origin',(41.9496306570156,9.05,-9.525));
#71540=CARTESIAN_POINT('',(36.4503693429844,9.05,-9.525));
#71541=CARTESIAN_POINT('',(37.8251846714922,9.05,-11.90625));
#71542=CARTESIAN_POINT('',(36.4503693429844,9.05,-9.525));
#71543=CARTESIAN_POINT('Origin',(39.2,9.05,-9.525));
#71544=CARTESIAN_POINT('Origin',(41.9496306570156,9.05,-9.525));
#71545=CARTESIAN_POINT('',(40.5748153285078,9.05,-11.90625));
#71546=CARTESIAN_POINT('',(37.8251846714922,9.05,-11.90625));
#71547=CARTESIAN_POINT('Origin',(39.2,9.05,-9.525));
#71548=CARTESIAN_POINT('Origin',(41.9496306570156,9.05,-9.525));
#71549=CARTESIAN_POINT('',(41.9496306570156,9.05,-9.525));
#71550=CARTESIAN_POINT('',(40.5748153285078,9.05,-11.90625));
#71551=CARTESIAN_POINT('Origin',(39.2,9.05,-9.525));
#71552=CARTESIAN_POINT('Origin',(41.9496306570156,9.05,-9.525));
#71553=CARTESIAN_POINT('',(40.5748153285078,9.05,-7.14375));
#71554=CARTESIAN_POINT('',(41.9496306570156,9.05,-9.525));
#71555=CARTESIAN_POINT('Origin',(39.2,9.05,-9.525));
#71556=CARTESIAN_POINT('Origin',(41.9496306570156,9.05,-9.525));
#71557=CARTESIAN_POINT('',(37.8251846714922,9.05,-7.14375));
#71558=CARTESIAN_POINT('',(40.5748153285078,9.05,-7.14375));
#71559=CARTESIAN_POINT('Origin',(39.2,9.05,-9.525));
#71560=CARTESIAN_POINT('Origin',(41.9496306570156,9.05,-9.525));
#71561=CARTESIAN_POINT('',(37.8251846714922,9.05,-7.14375));
#71562=CARTESIAN_POINT('Origin',(39.2,9.05,-9.525));
#71563=CARTESIAN_POINT('Origin',(39.2,9.05,-9.525));
#71564=CARTESIAN_POINT('',(39.2,7.39785522132845,-9.525));
#71565=CARTESIAN_POINT('',(36.4503693429844,9.05,-9.525));
#71566=CARTESIAN_POINT('Origin',(36.4503693429844,12.25,-9.525));
#71567=CARTESIAN_POINT('',(36.4503693429844,12.25,-9.525));
#71568=CARTESIAN_POINT('',(37.8251846714922,12.25,-11.90625));
#71569=CARTESIAN_POINT('Origin',(37.8251846714922,12.25,-7.14375));
#71570=CARTESIAN_POINT('',(37.8251846714922,12.25,-7.14375));
#71571=CARTESIAN_POINT('Origin',(40.5748153285078,12.25,-7.14375));
#71572=CARTESIAN_POINT('',(40.5748153285078,12.25,-7.14375));
#71573=CARTESIAN_POINT('Origin',(41.9496306570156,12.25,-9.525));
#71574=CARTESIAN_POINT('',(41.9496306570156,12.25,-9.525));
#71575=CARTESIAN_POINT('Origin',(40.5748153285078,12.25,-11.90625));
#71576=CARTESIAN_POINT('',(40.5748153285078,12.25,-11.90625));
#71577=CARTESIAN_POINT('Origin',(37.8251846714922,12.25,-11.90625));
#71782=UNCERTAINTY_MEASURE_WITH_UNIT(LENGTH_MEASURE(0.01),#71796,
'DISTANCE_ACCURACY_VALUE',
'Maximum model space distance between geometric entities at asserted c
onnectivities');
#71783=UNCERTAINTY_MEASURE_WITH_UNIT(LENGTH_MEASURE(0.01),#71796,
'DISTANCE_ACCURACY_VALUE',
'Maximum model space distance between geometric entities at asserted c
onnectivities');
#71794=(
GEOMETRIC_REPRESENTATION_CONTEXT(3)
GLOBAL_UNCERTAINTY_ASSIGNED_CONTEXT((#71782))
GLOBAL_UNIT_ASSIGNED_CONTEXT((#71796,#71798,#71799))
REPRESENTATION_CONTEXT('','3D')
);
#71795=(
GEOMETRIC_REPRESENTATION_CONTEXT(3)
GLOBAL_UNCERTAINTY_ASSIGNED_CONTEXT((#71783))
GLOBAL_UNIT_ASSIGNED_CONTEXT((#71796,#71798,#71799))
REPRESENTATION_CONTEXT('','3D')
);
#71796=(
LENGTH_UNIT()
NAMED_UNIT(*)
SI_UNIT(.MILLI.,.METRE.)
);
#71798=(
NAMED_UNIT(*)
PLANE_ANGLE_UNIT()
SI_UNIT($,.RADIAN.)
);
#71799=(
NAMED_UNIT(*)
SI_UNIT($,.STERADIAN.)
SOLID_ANGLE_UNIT()
);
#71810=SHAPE_DEFINITION_REPRESENTATION(#71821,#72026);
#71821=PRODUCT_DEFINITION_SHAPE('',$,#72038);
#72026=SHAPE_REPRESENTATION('',(#14610),#71794);
#72027=PRODUCT_DEFINITION_CONTEXT('part definition',#72062,'design');
#72038=PRODUCT_DEFINITION('ASME B18.3 SHCS 1-4-20 UNC x 0.75',
'ASME B18.3 SHCS 1-4-20 UNC x 0.75',#72049,#72027);
#72049=PRODUCT_DEFINITION_FORMATION('',$,#72074);
#72062=APPLICATION_CONTEXT(
'Core Data for Automotive Mechanical Design Process');
#72063=PRODUCT_CONTEXT('part definition',#72062,'mechanical');
#72074=PRODUCT('ASME B18.3 SHCS 1-4-20 UNC x 0.75',
'ASME B18.3 SHCS 1-4-20 UNC x 0.75',$,(#72063));
#72085=PRESENTATION_STYLE_ASSIGNMENT((#72096));
#72096=SURFACE_STYLE_USAGE(.BOTH.,#72107);
#72107=SURFACE_SIDE_STYLE('',(#72118));
#72118=SURFACE_STYLE_FILL_AREA(#72129);
#72129=FILL_AREA_STYLE('Opaque(196,201,207)',(#72140));
#72140=FILL_AREA_STYLE_COLOUR('Opaque(196,201,207)',#72151);
#72151=COLOUR_RGB('Opaque(196,201,207)', 0.40784314, 0.44705882, 0.49803922);
ENDSEC;
END-ISO-10303-21;
